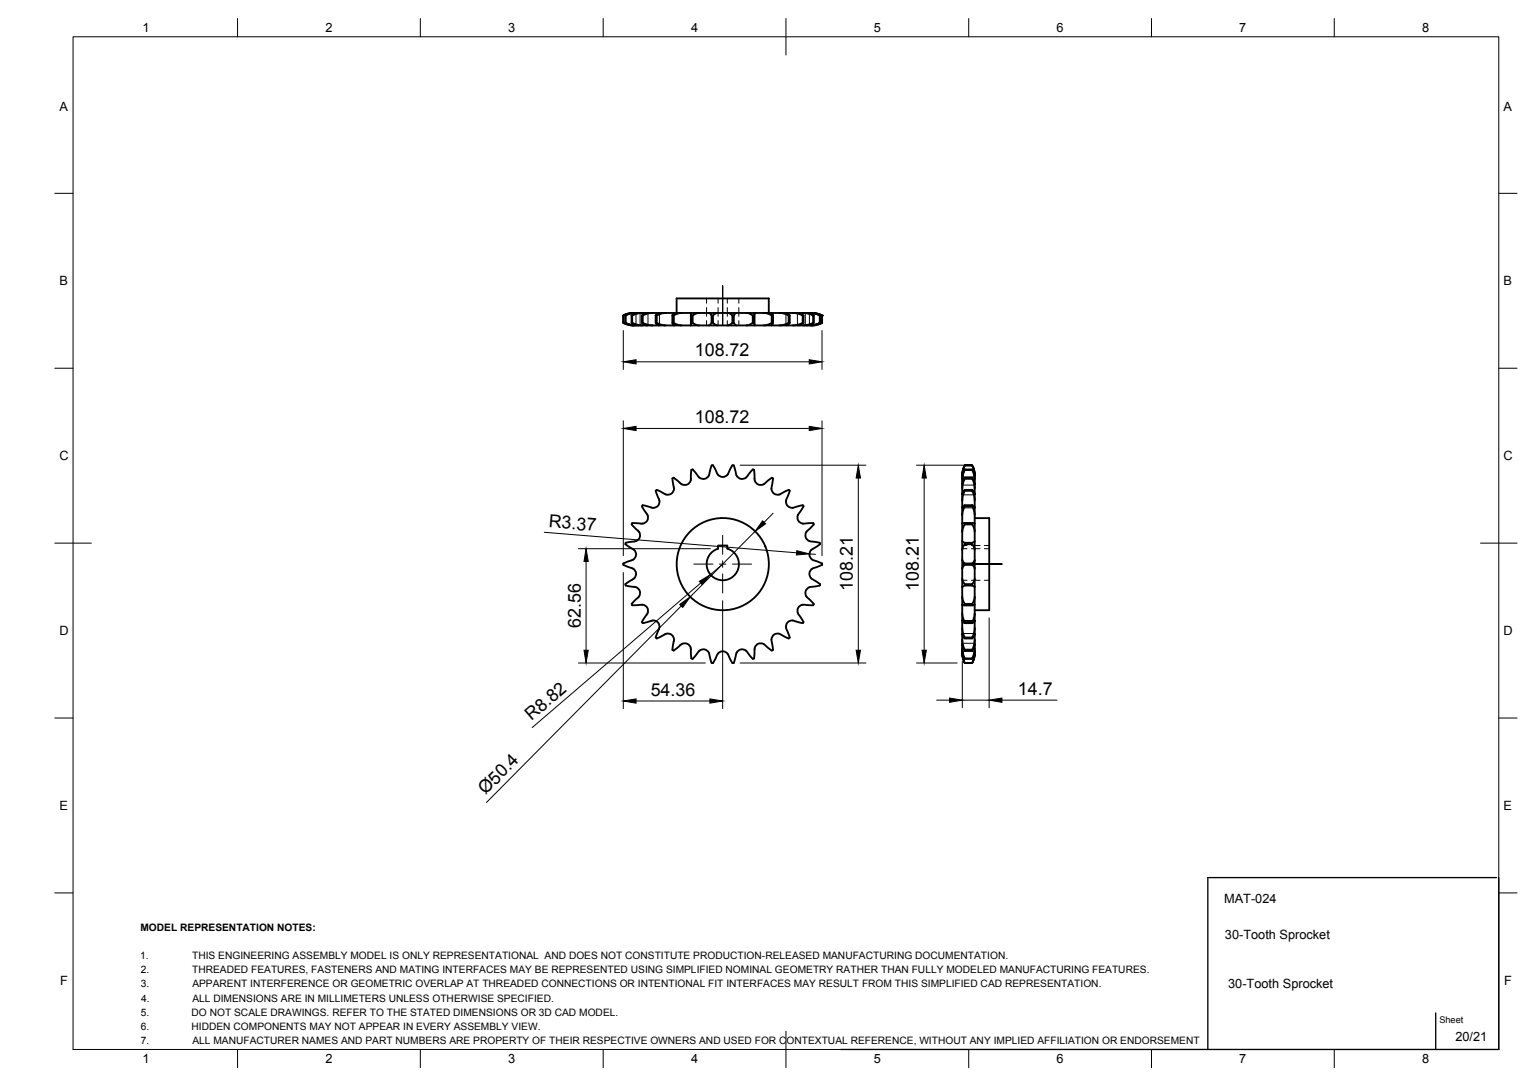
ISO-10303-21;
HEADER;
/* Generated by software containing ST-Developer
 * from STEP Tools, Inc. (www.steptools.com) 
 */

FILE_DESCRIPTION(
/* description */ ('STEP AP214'),
/* implementation_level */ '2;1');

FILE_NAME(
/* name */ '30-Tooth Sprocket.step',
/* time_stamp */ '2026-11-14T06:34:07-08:00',
/* author */ (''),
/* organization */ (''),
/* preprocessor_version */ 'ST-DEVELOPER v20.2',
/* originating_system */ 'Autodesk Translation Framework v15.17.0.0',
/* authorisation */ '');

FILE_SCHEMA (('AUTOMOTIVE_DESIGN { 1 0 10303 214 3 1 1 }'));
ENDSEC;

DATA;
#10=MECHANICAL_DESIGN_GEOMETRIC_PRESENTATION_REPRESENTATION('',(#7281),#310623);
#4055=TOROIDAL_SURFACE('',#103548,25.536,0.336);
#4056=TOROIDAL_SURFACE('',#103592,49.1019873874548,10.668);
#4057=TOROIDAL_SURFACE('',#103597,49.1019873874548,10.668);
#4058=TOROIDAL_SURFACE('',#103651,49.1019873874548,10.668);
#4059=TOROIDAL_SURFACE('',#103653,49.1019873874548,10.668);
#4060=TOROIDAL_SURFACE('',#103655,49.1019873874548,10.668);
#4061=TOROIDAL_SURFACE('',#103657,49.1019873874548,10.668);
#4062=TOROIDAL_SURFACE('',#103659,49.1019873874548,10.668);
#4063=TOROIDAL_SURFACE('',#103661,49.1019873874548,10.668);
#4064=TOROIDAL_SURFACE('',#103663,49.1019873874548,10.668);
#4065=TOROIDAL_SURFACE('',#103665,49.1019873874548,10.668);
#4066=TOROIDAL_SURFACE('',#103667,49.1019873874548,10.668);
#4067=TOROIDAL_SURFACE('',#103669,49.1019873874548,10.668);
#4068=TOROIDAL_SURFACE('',#103671,49.1019873874548,10.668);
#4069=TOROIDAL_SURFACE('',#103673,49.1019873874548,10.668);
#4070=TOROIDAL_SURFACE('',#103675,49.1019873874548,10.668);
#4071=TOROIDAL_SURFACE('',#103677,49.1019873874548,10.668);
#4072=TOROIDAL_SURFACE('',#103679,49.1019873874548,10.668);
#4073=TOROIDAL_SURFACE('',#103681,49.1019873874548,10.668);
#4074=TOROIDAL_SURFACE('',#103683,49.1019873874548,10.668);
#4075=TOROIDAL_SURFACE('',#103685,49.1019873874548,10.668);
#4076=TOROIDAL_SURFACE('',#103687,49.1019873874548,10.668);
#4077=TOROIDAL_SURFACE('',#103689,49.1019873874548,10.668);
#4078=TOROIDAL_SURFACE('',#103691,49.1019873874548,10.668);
#4079=TOROIDAL_SURFACE('',#103693,49.1019873874548,10.668);
#4080=TOROIDAL_SURFACE('',#103695,49.1019873874548,10.668);
#4081=TOROIDAL_SURFACE('',#103697,49.1019873874548,10.668);
#4082=TOROIDAL_SURFACE('',#103699,49.1019873874548,10.668);
#4083=TOROIDAL_SURFACE('',#103701,49.1019873874548,10.668);
#4084=TOROIDAL_SURFACE('',#103703,49.1019873874548,10.668);
#4085=TOROIDAL_SURFACE('',#103705,49.1019873874548,10.668);
#4086=TOROIDAL_SURFACE('',#103763,49.1019873874548,10.668);
#4087=TOROIDAL_SURFACE('',#103765,49.1019873874548,10.668);
#4088=TOROIDAL_SURFACE('',#103767,49.1019873874548,10.668);
#4089=TOROIDAL_SURFACE('',#103769,49.1019873874548,10.668);
#4090=TOROIDAL_SURFACE('',#103771,49.1019873874548,10.668);
#4091=TOROIDAL_SURFACE('',#103773,49.1019873874548,10.668);
#4092=TOROIDAL_SURFACE('',#103775,49.1019873874548,10.668);
#4093=TOROIDAL_SURFACE('',#103777,49.1019873874548,10.668);
#4094=TOROIDAL_SURFACE('',#103779,49.1019873874548,10.668);
#4095=TOROIDAL_SURFACE('',#103781,49.1019873874548,10.668);
#4096=TOROIDAL_SURFACE('',#103783,49.1019873874548,10.668);
#4097=TOROIDAL_SURFACE('',#103785,49.1019873874548,10.668);
#4098=TOROIDAL_SURFACE('',#103787,49.1019873874548,10.668);
#4099=TOROIDAL_SURFACE('',#103789,49.1019873874548,10.668);
#4100=TOROIDAL_SURFACE('',#103791,49.1019873874548,10.668);
#4101=TOROIDAL_SURFACE('',#103793,49.1019873874548,10.668);
#4102=TOROIDAL_SURFACE('',#103795,49.1019873874548,10.668);
#4103=TOROIDAL_SURFACE('',#103797,49.1019873874548,10.668);
#4104=TOROIDAL_SURFACE('',#103799,49.1019873874548,10.668);
#4105=TOROIDAL_SURFACE('',#103801,49.1019873874548,10.668);
#4106=TOROIDAL_SURFACE('',#103803,49.1019873874548,10.668);
#4107=TOROIDAL_SURFACE('',#103805,49.1019873874548,10.668);
#4108=TOROIDAL_SURFACE('',#103807,49.1019873874548,10.668);
#4109=TOROIDAL_SURFACE('',#103809,49.1019873874548,10.668);
#4110=TOROIDAL_SURFACE('',#103811,49.1019873874548,10.668);
#4111=TOROIDAL_SURFACE('',#103813,49.1019873874548,10.668);
#4112=TOROIDAL_SURFACE('',#103815,49.1019873874548,10.668);
#4113=TOROIDAL_SURFACE('',#103817,49.1019873874548,10.668);
#4114=TOROIDAL_SURFACE('',#103819,49.1019873874548,10.668);
#4115=TOROIDAL_SURFACE('',#103823,49.1019873874548,10.668);
#6426=B_SPLINE_CURVE_WITH_KNOTS('',3,(#272477,#272478,#272479,#272480,#272481,
#272482),.UNSPECIFIED.,.F.,.F.,(4,2,4),(-1.6873876187543,-1.63190661744399,
-1.18678936119335),.UNSPECIFIED.);
#6427=B_SPLINE_CURVE_WITH_KNOTS('',3,(#272486,#272487,#272488,#272489,#272490,
#272491,#272492,#272493),.UNSPECIFIED.,.F.,.F.,(4,2,2,4),(-5.73653316281924,
-5.72047347154335,-5.28796112447222,-5.23617773822564),.UNSPECIFIED.);
#6428=B_SPLINE_CURVE_WITH_KNOTS('',3,(#272498,#272499,#272500,#272501,#272502,
#272503,#272504,#272505),.UNSPECIFIED.,.F.,.F.,(4,2,2,4),(-5.73653316281959,
-5.72047347154369,-5.28796112447255,-5.23617773822598),.UNSPECIFIED.);
#6429=B_SPLINE_CURVE_WITH_KNOTS('',3,(#272509,#272510,#272511,#272512,#272513,
#272514),.UNSPECIFIED.,.F.,.F.,(4,2,4),(-1.68738761875429,-1.63190661744397,
-1.18678936119331),.UNSPECIFIED.);
#6430=B_SPLINE_CURVE_WITH_KNOTS('',3,(#272521,#272522,#272523,#272524,#272525,
#272526,#272527,#272528,#272529,#272530),.UNSPECIFIED.,.F.,.F.,(4,3,3,4),
(0.00710274596862205,0.00747376540688557,0.00783502386845829,0.00801837063754701),
 .UNSPECIFIED.);
#6431=B_SPLINE_CURVE_WITH_KNOTS('',3,(#272534,#272535,#272536,#272537),
 .UNSPECIFIED.,.F.,.F.,(4,4),(0.673390429668365,0.765903724821262),
 .UNSPECIFIED.);
#6432=B_SPLINE_CURVE_WITH_KNOTS('',3,(#272541,#272542,#272543,#272544,#272545,
#272546,#272547,#272548,#272549,#272550),.UNSPECIFIED.,.F.,.F.,(4,3,3,4),
(0.00710284094402589,0.00747383068998922,0.00783505699281219,0.0080184642589637),
 .UNSPECIFIED.);
#6433=B_SPLINE_CURVE_WITH_KNOTS('',3,(#272553,#272554,#272555,#272556,#272557,
#272558),.UNSPECIFIED.,.F.,.F.,(4,2,4),(1.75167822390513,1.82489845087556,
1.84415950245262),.UNSPECIFIED.);
#6434=B_SPLINE_CURVE_WITH_KNOTS('',3,(#272564,#272565,#272566,#272567,#272568,
#272569,#272570,#272571,#272572,#272573),.UNSPECIFIED.,.F.,.F.,(4,3,3,4),
(0.00710274294853988,0.00747376648681281,0.00783502929878955,0.00801836762245747),
 .UNSPECIFIED.);
#6435=B_SPLINE_CURVE_WITH_KNOTS('',3,(#272577,#272578,#272579,#272580),
 .UNSPECIFIED.,.F.,.F.,(4,4),(0.673390429683384,0.765903724839824),
 .UNSPECIFIED.);
#6436=B_SPLINE_CURVE_WITH_KNOTS('',3,(#272584,#272585,#272586,#272587,#272588,
#272589,#272590,#272591,#272592,#272593),.UNSPECIFIED.,.F.,.F.,(4,3,3,4),
(0.0071027909646029,0.00747379949023628,0.00783504604208146,0.00801841495400679),
 .UNSPECIFIED.);
#6437=B_SPLINE_CURVE_WITH_KNOTS('',3,(#272596,#272597,#272598,#272599,#272600,
#272601),.UNSPECIFIED.,.F.,.F.,(4,2,4),(1.7516782239595,1.82489845093397,
1.84415950251209),.UNSPECIFIED.);
#6438=B_SPLINE_CURVE_WITH_KNOTS('',3,(#272607,#272608,#272609,#272610,#272611,
#272612,#272613,#272614,#272615,#272616),.UNSPECIFIED.,.F.,.F.,(4,3,3,4),
(0.00710274848401425,0.00747377224143413,0.00783503523508107,0.00801837305550075),
 .UNSPECIFIED.);
#6439=B_SPLINE_CURVE_WITH_KNOTS('',3,(#272620,#272621,#272622,#272623),
 .UNSPECIFIED.,.F.,.F.,(4,4),(0.673390432198586,0.765903727898388),
 .UNSPECIFIED.);
#6440=B_SPLINE_CURVE_WITH_KNOTS('',3,(#272627,#272628,#272629,#272630,#272631,
#272632,#272633,#272634,#272635,#272636),.UNSPECIFIED.,.F.,.F.,(4,3,3,4),
(0.00710275267632021,0.00747377512290787,0.00783503669679513,0.00801837718804213),
 .UNSPECIFIED.);
#6441=B_SPLINE_CURVE_WITH_KNOTS('',3,(#272639,#272640,#272641,#272642,#272643,
#272644),.UNSPECIFIED.,.F.,.F.,(4,2,4),(1.75167822396455,1.82489845093931,
1.84415950251752),.UNSPECIFIED.);
#6442=B_SPLINE_CURVE_WITH_KNOTS('',3,(#272650,#272651,#272652,#272653,#272654,
#272655,#272656,#272657,#272658,#272659),.UNSPECIFIED.,.F.,.F.,(4,3,3,4),
(0.00710274372650064,0.00747376845075347,0.00783503250649641,0.00801836837208912),
 .UNSPECIFIED.);
#6443=B_SPLINE_CURVE_WITH_KNOTS('',3,(#272663,#272664,#272665,#272666),
 .UNSPECIFIED.,.F.,.F.,(4,4),(0.673390432227944,0.765903727934262),
 .UNSPECIFIED.);
#6444=B_SPLINE_CURVE_WITH_KNOTS('',3,(#272670,#272671,#272672,#272673,#272674,
#272675,#272676,#272677,#272678,#272679),.UNSPECIFIED.,.F.,.F.,(4,3,3,4),
(0.00710276617990407,0.00747378388366959,0.00783504033541444,0.00801839050540093),
 .UNSPECIFIED.);
#6445=B_SPLINE_CURVE_WITH_KNOTS('',3,(#272682,#272683,#272684,#272685,#272686,
#272687),.UNSPECIFIED.,.F.,.F.,(4,2,4),(1.7516782239634,1.82489845093825,
1.84415950251648),.UNSPECIFIED.);
#6446=B_SPLINE_CURVE_WITH_KNOTS('',3,(#272691,#272692,#272693,#272694,#272695,
#272696),.UNSPECIFIED.,.F.,.F.,(4,2,4),(0.311414679923399,0.386708223984938,
0.403787209257592),.UNSPECIFIED.);
#6447=B_SPLINE_CURVE_WITH_KNOTS('',3,(#272700,#272701,#272702,#272703),
 .UNSPECIFIED.,.F.,.F.,(4,4),(0.673390427100202,0.765903721697738),
 .UNSPECIFIED.);
#6448=B_SPLINE_CURVE_WITH_KNOTS('',3,(#272707,#272708,#272709,#272710,#272711,
#272712,#272713,#272714,#272715,#272716),.UNSPECIFIED.,.F.,.F.,(4,3,3,4),
(0.00710274287152855,0.00747376729113706,0.00783503103327042,0.00801836753620372),
 .UNSPECIFIED.);
#6449=B_SPLINE_CURVE_WITH_KNOTS('',3,(#272720,#272721,#272722,#272723,#272724,
#272725),.UNSPECIFIED.,.F.,.F.,(4,2,4),(1.75167822395949,1.82489845093397,
1.8441595025121),.UNSPECIFIED.);
#6450=B_SPLINE_CURVE_WITH_KNOTS('',3,(#272730,#272731,#272732,#272733,#272734,
#272735),.UNSPECIFIED.,.F.,.F.,(4,2,4),(0.311414679921635,0.386708223982506,
0.403787209254994),.UNSPECIFIED.);
#6451=B_SPLINE_CURVE_WITH_KNOTS('',3,(#272739,#272740,#272741,#272742),
 .UNSPECIFIED.,.F.,.F.,(4,4),(0.67339042968077,0.765903724836084),
 .UNSPECIFIED.);
#6452=B_SPLINE_CURVE_WITH_KNOTS('',3,(#272746,#272747,#272748,#272749,#272750,
#272751,#272752,#272753,#272754,#272755),.UNSPECIFIED.,.F.,.F.,(4,3,3,4),
(0.00710274556156679,0.00747377006444483,0.00783503387032176,0.00801837017674505),
 .UNSPECIFIED.);
#6453=B_SPLINE_CURVE_WITH_KNOTS('',3,(#272759,#272760,#272761,#272762,#272763,
#272764),.UNSPECIFIED.,.F.,.F.,(4,2,4),(1.75167822393186,1.82489845090426,
1.84415950248185),.UNSPECIFIED.);
#6454=B_SPLINE_CURVE_WITH_KNOTS('',3,(#272769,#272770,#272771,#272772,#272773,
#272774),.UNSPECIFIED.,.F.,.F.,(4,2,4),(1.75167822396114,1.82489845093575,
1.84415950251343),.UNSPECIFIED.);
#6455=B_SPLINE_CURVE_WITH_KNOTS('',3,(#272778,#272779,#272780,#272781,#272782,
#272783,#272784,#272785,#272786,#272787),.UNSPECIFIED.,.F.,.F.,(4,3,3,4),
(0.00710274556156676,0.00747377006444954,0.00783503387033569,0.00801837017674508),
 .UNSPECIFIED.);
#6456=B_SPLINE_CURVE_WITH_KNOTS('',3,(#272791,#272792,#272793,#272794),
 .UNSPECIFIED.,.F.,.F.,(4,4),(0.673390429683286,0.765903724839261),
 .UNSPECIFIED.);
#6457=B_SPLINE_CURVE_WITH_KNOTS('',3,(#272798,#272799,#272800,#272801,#272802,
#272803),.UNSPECIFIED.,.F.,.F.,(4,2,4),(1.38841536190411,1.44431919666813,
1.480702891614),.UNSPECIFIED.);
#6458=B_SPLINE_CURVE_WITH_KNOTS('',3,(#272810,#272811,#272812,#272813,#272814,
#272815,#272816,#272817,#272818,#272819),.UNSPECIFIED.,.F.,.F.,(4,3,3,4),
(0.00710275267632017,0.00747377512292421,0.00783503669676932,0.00801837718804213),
 .UNSPECIFIED.);
#6459=B_SPLINE_CURVE_WITH_KNOTS('',3,(#272823,#272824,#272825,#272826),
 .UNSPECIFIED.,.F.,.F.,(4,4),(0.673390429659051,0.765903724809687),
 .UNSPECIFIED.);
#6460=B_SPLINE_CURVE_WITH_KNOTS('',3,(#272830,#272831,#272832,#272833,#272834,
#272835,#272836,#272837,#272838,#272839),.UNSPECIFIED.,.F.,.F.,(4,3,3,4),
(0.00710274848401431,0.00747377224144616,0.00783503523508854,0.00801837305550078),
 .UNSPECIFIED.);
#6461=B_SPLINE_CURVE_WITH_KNOTS('',3,(#272842,#272843,#272844,#272845,#272846,
#272847),.UNSPECIFIED.,.F.,.F.,(4,2,4),(1.75167822393867,1.82489845091149,
1.8441595024892),.UNSPECIFIED.);
#6462=B_SPLINE_CURVE_WITH_KNOTS('',3,(#272851,#272852,#272853,#272854,#272855,
#272856),.UNSPECIFIED.,.F.,.F.,(4,2,4),(1.75167822389203,1.8248984508612,
1.84415950243739),.UNSPECIFIED.);
#6463=B_SPLINE_CURVE_WITH_KNOTS('',3,(#272860,#272861,#272862,#272863,#272864,
#272865,#272866,#272867,#272868,#272869),.UNSPECIFIED.,.F.,.F.,(4,3,3,4),
(0.00710274287152849,0.00747376729116317,0.00783503103329361,0.00801836753620371),
 .UNSPECIFIED.);
#6464=B_SPLINE_CURVE_WITH_KNOTS('',3,(#272873,#272874,#272875,#272876),
 .UNSPECIFIED.,.F.,.F.,(4,4),(0.673390429665128,0.765903724817488),
 .UNSPECIFIED.);
#6465=B_SPLINE_CURVE_WITH_KNOTS('',3,(#272880,#272881,#272882,#272883,#272884,
#272885),.UNSPECIFIED.,.F.,.F.,(4,2,4),(1.38841536184886,1.444319196609,
1.48070289155233),.UNSPECIFIED.);
#6466=B_SPLINE_CURVE_WITH_KNOTS('',3,(#272892,#272893,#272894,#272895,#272896,
#272897,#272898,#272899,#272900,#272901),.UNSPECIFIED.,.F.,.F.,(4,3,3,4),
(0.00710276617990401,0.00747378388366924,0.00783504033542184,0.00801839050540089),
 .UNSPECIFIED.);
#6467=B_SPLINE_CURVE_WITH_KNOTS('',3,(#272905,#272906,#272907,#272908),
 .UNSPECIFIED.,.F.,.F.,(4,4),(0.673390432231233,0.765903727938084),
 .UNSPECIFIED.);
#6468=B_SPLINE_CURVE_WITH_KNOTS('',3,(#272912,#272913,#272914,#272915,#272916,
#272917,#272918,#272919,#272920,#272921),.UNSPECIFIED.,.F.,.F.,(4,3,3,4),
(0.00710274372650068,0.00747376845078837,0.00783503250653971,0.00801836837208909),
 .UNSPECIFIED.);
#6469=B_SPLINE_CURVE_WITH_KNOTS('',3,(#272924,#272925,#272926,#272927,#272928,
#272929),.UNSPECIFIED.,.F.,.F.,(4,2,4),(1.75167822389501,1.82489845086412,
1.84415950244083),.UNSPECIFIED.);
#6470=B_SPLINE_CURVE_WITH_KNOTS('',3,(#272935,#272936,#272937,#272938,#272939,
#272940,#272941,#272942,#272943,#272944),.UNSPECIFIED.,.F.,.F.,(4,3,3,4),
(0.00710279096460286,0.00747379949026601,0.00783504604209238,0.0080184149540068),
 .UNSPECIFIED.);
#6471=B_SPLINE_CURVE_WITH_KNOTS('',3,(#272948,#272949,#272950,#272951),
 .UNSPECIFIED.,.F.,.F.,(4,4),(0.673390429675743,0.765903724830226),
 .UNSPECIFIED.);
#6472=B_SPLINE_CURVE_WITH_KNOTS('',3,(#272955,#272956,#272957,#272958,#272959,
#272960,#272961,#272962,#272963,#272964),.UNSPECIFIED.,.F.,.F.,(4,3,3,4),
(0.00710274294853991,0.0074737664867412,0.0078350292986902,0.00801836762245745),
 .UNSPECIFIED.);
#6473=B_SPLINE_CURVE_WITH_KNOTS('',3,(#272967,#272968,#272969,#272970,#272971,
#272972),.UNSPECIFIED.,.F.,.F.,(4,2,4),(1.75167822398024,1.82489845095654,
1.8441595025352),.UNSPECIFIED.);
#6474=B_SPLINE_CURVE_WITH_KNOTS('',3,(#272978,#272979,#272980,#272981,#272982,
#272983,#272984,#272985,#272986,#272987),.UNSPECIFIED.,.F.,.F.,(4,3,3,4),
(0.00710284094402584,0.00747383069000615,0.00783505699282562,0.00801846425896367),
 .UNSPECIFIED.);
#6475=B_SPLINE_CURVE_WITH_KNOTS('',3,(#272991,#272992,#272993,#272994),
 .UNSPECIFIED.,.F.,.F.,(4,4),(0.673390429692054,0.765903724850254),
 .UNSPECIFIED.);
#6476=B_SPLINE_CURVE_WITH_KNOTS('',3,(#272998,#272999,#273000,#273001,#273002,
#273003,#273004,#273005,#273006,#273007),.UNSPECIFIED.,.F.,.F.,(4,3,3,4),
(0.00710274596862209,0.00747376540702079,0.00783502386859213,0.00801837063754698),
 .UNSPECIFIED.);
#6477=B_SPLINE_CURVE_WITH_KNOTS('',3,(#273010,#273011,#273012,#273013,#273014,
#273015),.UNSPECIFIED.,.F.,.F.,(4,2,4),(1.75167822394042,1.82489845091343,
1.84415950249118),.UNSPECIFIED.);
#6478=B_SPLINE_CURVE_WITH_KNOTS('',3,(#273021,#273022,#273023,#273024,#273025,
#273026),.UNSPECIFIED.,.F.,.F.,(4,2,4),(-1.68738761875423,-1.63190661744391,
-1.18678936119335),.UNSPECIFIED.);
#6479=B_SPLINE_CURVE_WITH_KNOTS('',3,(#273028,#273029,#273030,#273031,#273032,
#273033,#273034,#273035,#273036,#273037),.UNSPECIFIED.,.F.,.F.,(4,3,3,4),
(0.00710284094402589,0.00747383068999436,0.00783505699281514,0.0080184642589637),
 .UNSPECIFIED.);
#6480=B_SPLINE_CURVE_WITH_KNOTS('',3,(#273041,#273042,#273043,#273044),
 .UNSPECIFIED.,.F.,.F.,(4,4),(0.673390429666604,0.7659037248194),
 .UNSPECIFIED.);
#6481=B_SPLINE_CURVE_WITH_KNOTS('',3,(#273045,#273046,#273047,#273048,#273049,
#273050,#273051,#273052),.UNSPECIFIED.,.F.,.F.,(4,2,2,4),(-5.73653316281647,
-5.7204734715406,-5.28796112446986,-5.23617773822333),.UNSPECIFIED.);
#6482=B_SPLINE_CURVE_WITH_KNOTS('',3,(#273064,#273065,#273066,#273067,#273068,
#273069),.UNSPECIFIED.,.F.,.F.,(4,2,4),(1.75167822396951,1.82489845094498,
1.84415950252339),.UNSPECIFIED.);
#6483=B_SPLINE_CURVE_WITH_KNOTS('',3,(#273070,#273071,#273072,#273073,#273074,
#273075,#273076,#273077),.UNSPECIFIED.,.F.,.F.,(4,2,2,4),(-5.73653316281843,
-5.72047347154254,-5.28796112447152,-5.23617773822495),.UNSPECIFIED.);
#6484=B_SPLINE_CURVE_WITH_KNOTS('',3,(#273079,#273080,#273081,#273082,#273083,
#273084),.UNSPECIFIED.,.F.,.F.,(4,2,4),(-1.68738761875408,-1.63190661744377,
-1.18678936119326),.UNSPECIFIED.);
#6485=B_SPLINE_CURVE_WITH_KNOTS('',3,(#273085,#273086,#273087,#273088,#273089,
#273090,#273091,#273092,#273093,#273094),.UNSPECIFIED.,.F.,.F.,(4,3,3,4),
(0.00710284094402584,0.00747383068999716,0.00783505699282223,0.00801846425896371),
 .UNSPECIFIED.);
#6486=B_SPLINE_CURVE_WITH_KNOTS('',3,(#273200,#273201,#273202,#273203,#273204,
#273205,#273206,#273207),.UNSPECIFIED.,.F.,.F.,(4,2,2,4),(-5.73653316281843,
-5.72047347154255,-5.28796112447153,-5.23617773822497),.UNSPECIFIED.);
#6487=B_SPLINE_CURVE_WITH_KNOTS('',3,(#273211,#273212,#273213,#273214,#273215,
#273216),.UNSPECIFIED.,.F.,.F.,(4,2,4),(-1.68738761875411,-1.6319066174438,
-1.18678936119328),.UNSPECIFIED.);
#6488=B_SPLINE_CURVE_WITH_KNOTS('',3,(#273217,#273218,#273219,#273220,#273221,
#273222,#273223,#273224,#273225,#273226),.UNSPECIFIED.,.F.,.F.,(4,3,3,4),
(0.00710279096460287,0.00747379949022753,0.00783504604206607,0.00801841495400678),
 .UNSPECIFIED.);
#6489=B_SPLINE_CURVE_WITH_KNOTS('',3,(#273227,#273228,#273229,#273230,#273231,
#273232),.UNSPECIFIED.,.F.,.F.,(4,2,4),(1.75167822397008,1.82489845094558,
1.84415950252402),.UNSPECIFIED.);
#6490=B_SPLINE_CURVE_WITH_KNOTS('',3,(#273235,#273236,#273237,#273238,#273239,
#273240,#273241,#273242,#273243,#273244),.UNSPECIFIED.,.F.,.F.,(4,3,3,4),
(0.00710274596862205,0.00747376540693236,0.00783502386849402,0.00801837063754702),
 .UNSPECIFIED.);
#6491=B_SPLINE_CURVE_WITH_KNOTS('',3,(#273246,#273247,#273248,#273249,#273250,
#273251),.UNSPECIFIED.,.F.,.F.,(4,2,4),(1.75167822396416,1.82489845093897,
1.84415950251715),.UNSPECIFIED.);
#6492=B_SPLINE_CURVE_WITH_KNOTS('',3,(#273253,#273254,#273255,#273256,#273257,
#273258,#273259,#273260),.UNSPECIFIED.,.F.,.F.,(4,2,2,4),(-5.73653316281831,
-5.72047347154243,-5.28796112447143,-5.23617773822487),.UNSPECIFIED.);
#6493=B_SPLINE_CURVE_WITH_KNOTS('',3,(#273263,#273264,#273265,#273266,#273267,
#273268),.UNSPECIFIED.,.F.,.F.,(4,2,4),(-1.68738761875401,-1.63190661744371,
-1.18678936119322),.UNSPECIFIED.);
#6494=B_SPLINE_CURVE_WITH_KNOTS('',3,(#273271,#273272,#273273,#273274,#273275,
#273276,#273277,#273278,#273279,#273280),.UNSPECIFIED.,.F.,.F.,(4,3,3,4),
(0.00710274294853987,0.00747376648670428,0.00783502929868148,0.00801836762245748),
 .UNSPECIFIED.);
#6495=B_SPLINE_CURVE_WITH_KNOTS('',3,(#273282,#273283,#273284,#273285,#273286,
#273287),.UNSPECIFIED.,.F.,.F.,(4,2,4),(1.75167822398049,1.82489845095657,
1.84415950253511),.UNSPECIFIED.);
#6496=B_SPLINE_CURVE_WITH_KNOTS('',3,(#273289,#273290,#273291,#273292,#273293,
#273294,#273295,#273296),.UNSPECIFIED.,.F.,.F.,(4,2,2,4),(-5.73653316281822,
-5.72047347154233,-5.28796112447135,-5.23617773822479),.UNSPECIFIED.);
#6497=B_SPLINE_CURVE_WITH_KNOTS('',3,(#273299,#273300,#273301,#273302,#273303,
#273304),.UNSPECIFIED.,.F.,.F.,(4,2,4),(-1.68738761875411,-1.6319066174438,
-1.18678936119327),.UNSPECIFIED.);
#6498=B_SPLINE_CURVE_WITH_KNOTS('',3,(#273307,#273308,#273309,#273310,#273311,
#273312,#273313,#273314,#273315,#273316),.UNSPECIFIED.,.F.,.F.,(4,3,3,4),
(0.00710274372650065,0.00747376845074211,0.00783503250649763,0.00801836837208913),
 .UNSPECIFIED.);
#6499=B_SPLINE_CURVE_WITH_KNOTS('',3,(#273318,#273319,#273320,#273321,#273322,
#273323),.UNSPECIFIED.,.F.,.F.,(4,2,4),(1.75167822398513,1.82489845096143,
1.84415950254005),.UNSPECIFIED.);
#6500=B_SPLINE_CURVE_WITH_KNOTS('',3,(#273325,#273326,#273327,#273328,#273329,
#273330,#273331,#273332),.UNSPECIFIED.,.F.,.F.,(4,2,2,4),(-5.73653316281763,
-5.72047347154175,-5.2879611244708,-5.23617773822424),.UNSPECIFIED.);
#6501=B_SPLINE_CURVE_WITH_KNOTS('',3,(#273335,#273336,#273337,#273338,#273339,
#273340),.UNSPECIFIED.,.F.,.F.,(4,2,4),(-1.68738761875406,-1.63190661744375,
-1.18678936119324),.UNSPECIFIED.);
#6502=B_SPLINE_CURVE_WITH_KNOTS('',3,(#273344,#273345,#273346,#273347,#273348,
#273349,#273350,#273351),.UNSPECIFIED.,.F.,.F.,(4,2,2,4),(-5.73653316281763,
-5.72047347154175,-5.28796112447086,-5.2361777382243),.UNSPECIFIED.);
#6503=B_SPLINE_CURVE_WITH_KNOTS('',3,(#273355,#273356,#273357,#273358,#273359,
#273360),.UNSPECIFIED.,.F.,.F.,(4,2,4),(-1.6873876187539,-1.6319066174436,
-1.18678936119314),.UNSPECIFIED.);
#6504=B_SPLINE_CURVE_WITH_KNOTS('',3,(#273361,#273362,#273363,#273364,#273365,
#273366,#273367,#273368,#273369,#273370),.UNSPECIFIED.,.F.,.F.,(4,3,3,4),
(0.00710275842609582,0.00747377890657602,0.00783503835572276,0.00801838285788017),
 .UNSPECIFIED.);
#6505=B_SPLINE_CURVE_WITH_KNOTS('',3,(#273371,#273372,#273373,#273374,#273375,
#273376),.UNSPECIFIED.,.F.,.F.,(4,2,4),(1.75167822396027,1.82489845093474,
1.84415950251286),.UNSPECIFIED.);
#6506=B_SPLINE_CURVE_WITH_KNOTS('',3,(#273378,#273379,#273380,#273381,#273382,
#273383,#273384,#273385,#273386,#273387),.UNSPECIFIED.,.F.,.F.,(4,3,3,4),
(0.00710277664195228,0.00747379050272964,0.00783504280851268,0.00801840082520104),
 .UNSPECIFIED.);
#6507=B_SPLINE_CURVE_WITH_KNOTS('',3,(#273389,#273390,#273391,#273392,#273393,
#273394),.UNSPECIFIED.,.F.,.F.,(4,2,4),(1.75167822402901,1.82489845100883,
1.84415950258839),.UNSPECIFIED.);
#6508=B_SPLINE_CURVE_WITH_KNOTS('',3,(#273396,#273397,#273398,#273399,#273400,
#273401,#273402,#273403),.UNSPECIFIED.,.F.,.F.,(4,2,2,4),(-5.73653316281821,
-5.72047347154232,-5.28796112447134,-5.23617773822477),.UNSPECIFIED.);
#6509=B_SPLINE_CURVE_WITH_KNOTS('',3,(#273407,#273408,#273409,#273410,#273411,
#273412,#273413,#273414,#273415,#273416),.UNSPECIFIED.,.F.,.F.,(4,3,3,4),
(0.00710274848401426,0.00747377224139712,0.00783503523503374,0.00801837305550079),
 .UNSPECIFIED.);
#6510=B_SPLINE_CURVE_WITH_KNOTS('',3,(#273418,#273419,#273420,#273421,#273422,
#273423),.UNSPECIFIED.,.F.,.F.,(4,2,4),(1.75167822392663,1.82489845089845,
1.84415950247588),.UNSPECIFIED.);
#6511=B_SPLINE_CURVE_WITH_KNOTS('',3,(#273425,#273426,#273427,#273428,#273429,
#273430,#273431,#273432),.UNSPECIFIED.,.F.,.F.,(4,2,2,4),(-5.73653316281796,
-5.72047347154208,-5.28796112447113,-5.23617773822457),.UNSPECIFIED.);
#6512=B_SPLINE_CURVE_WITH_KNOTS('',3,(#273435,#273436,#273437,#273438,#273439,
#273440),.UNSPECIFIED.,.F.,.F.,(4,2,4),(-1.68738761875412,-1.63190661744382,
-1.1867893611933),.UNSPECIFIED.);
#6513=B_SPLINE_CURVE_WITH_KNOTS('',3,(#273444,#273445,#273446,#273447,#273448,
#273449,#273450,#273451),.UNSPECIFIED.,.F.,.F.,(4,2,2,4),(-5.73653316281711,
-5.72047347154123,-5.28796112447036,-5.23617773822381),.UNSPECIFIED.);
#6514=B_SPLINE_CURVE_WITH_KNOTS('',3,(#273455,#273456,#273457,#273458,#273459,
#273460),.UNSPECIFIED.,.F.,.F.,(4,2,4),(-1.68738761875405,-1.63190661744374,
-1.18678936119325),.UNSPECIFIED.);
#6515=B_SPLINE_CURVE_WITH_KNOTS('',3,(#273461,#273462,#273463,#273464,#273465,
#273466,#273467,#273468,#273469,#273470),.UNSPECIFIED.,.F.,.F.,(4,3,3,4),
(0.00710281114521604,0.00747381210003836,0.00783505048827464,0.00801843486213954),
 .UNSPECIFIED.);
#6516=B_SPLINE_CURVE_WITH_KNOTS('',3,(#273471,#273472,#273473,#273474,#273475,
#273476),.UNSPECIFIED.,.F.,.F.,(4,2,4),(1.75167822397278,1.8248984509485,
1.84415950252695),.UNSPECIFIED.);
#6517=B_SPLINE_CURVE_WITH_KNOTS('',3,(#273479,#273480,#273481,#273482,#273483,
#273484,#273485,#273486,#273487,#273488),.UNSPECIFIED.,.F.,.F.,(4,3,3,4),
(0.0071027490873384,0.00747377283389233,0.0078350358106713,0.00801837364807993),
 .UNSPECIFIED.);
#6518=B_SPLINE_CURVE_WITH_KNOTS('',3,(#273490,#273491,#273492,#273493,#273494,
#273495),.UNSPECIFIED.,.F.,.F.,(4,2,4),(1.75167822393089,1.82489845090296,
1.84415950248043),.UNSPECIFIED.);
#6519=B_SPLINE_CURVE_WITH_KNOTS('',3,(#273497,#273498,#273499,#273500,#273501,
#273502,#273503,#273504),.UNSPECIFIED.,.F.,.F.,(4,2,2,4),(-5.73653316281819,
-5.7204734715423,-5.2879611244713,-5.23617773822474),.UNSPECIFIED.);
#6520=B_SPLINE_CURVE_WITH_KNOTS('',3,(#273507,#273508,#273509,#273510,#273511,
#273512),.UNSPECIFIED.,.F.,.F.,(4,2,4),(-1.68738761875405,-1.63190661744374,
-1.18678936119326),.UNSPECIFIED.);
#6521=B_SPLINE_CURVE_WITH_KNOTS('',3,(#273515,#273516,#273517,#273518,#273519,
#273520,#273521,#273522,#273523,#273524),.UNSPECIFIED.,.F.,.F.,(4,3,3,4),
(0.00710274396181581,0.00747376592129383,0.00783502705943546,0.00801836863650809),
 .UNSPECIFIED.);
#6522=B_SPLINE_CURVE_WITH_KNOTS('',3,(#273525,#273526,#273527,#273528,#273529,
#273530),.UNSPECIFIED.,.F.,.F.,(4,2,4),(1.75167822392141,1.82489845089256,
1.84415950246982),.UNSPECIFIED.);
#6523=B_SPLINE_CURVE_WITH_KNOTS('',3,(#273533,#273534,#273535,#273536,#273537,
#273538),.UNSPECIFIED.,.F.,.F.,(4,2,4),(-1.68738761875407,-1.63190661744377,
-1.18678936119326),.UNSPECIFIED.);
#6524=B_SPLINE_CURVE_WITH_KNOTS('',3,(#273542,#273543,#273544,#273545,#273546,
#273547,#273548,#273549),.UNSPECIFIED.,.F.,.F.,(4,2,2,4),(-5.73653316281851,
-5.72047347154262,-5.2879611244716,-5.23617773822503),.UNSPECIFIED.);
#6525=B_SPLINE_CURVE_WITH_KNOTS('',3,(#273553,#273554,#273555,#273556,#273557,
#273558),.UNSPECIFIED.,.F.,.F.,(4,2,4),(-1.68738761875428,-1.63190661744396,
-1.18678936119339),.UNSPECIFIED.);
#6526=B_SPLINE_CURVE_WITH_KNOTS('',3,(#273559,#273560,#273561,#273562,#273563,
#273564,#273565,#273566,#273567,#273568),.UNSPECIFIED.,.F.,.F.,(4,3,3,4),
(0.00710274287152851,0.00747376729109832,0.00783503103323433,0.00801836753620372),
 .UNSPECIFIED.);
#6527=B_SPLINE_CURVE_WITH_KNOTS('',3,(#273569,#273570,#273571,#273572,#273573,
#273574),.UNSPECIFIED.,.F.,.F.,(4,2,4),(1.75167822396654,1.8248984509415,
1.84415950251975),.UNSPECIFIED.);
#6528=B_SPLINE_CURVE_WITH_KNOTS('',3,(#273577,#273578,#273579,#273580,#273581,
#273582,#273583,#273584,#273585,#273586),.UNSPECIFIED.,.F.,.F.,(4,3,3,4),
(0.00710274556156676,0.00747377006442299,0.00783503387029698,0.00801837017674507),
 .UNSPECIFIED.);
#6529=B_SPLINE_CURVE_WITH_KNOTS('',3,(#273588,#273589,#273590,#273591,#273592,
#273593),.UNSPECIFIED.,.F.,.F.,(4,2,4),(1.75167822394173,1.82489845091482,
1.84415950249256),.UNSPECIFIED.);
#6530=B_SPLINE_CURVE_WITH_KNOTS('',3,(#273595,#273596,#273597,#273598,#273599,
#273600,#273601,#273602),.UNSPECIFIED.,.F.,.F.,(4,2,2,4),(-5.73653316281893,
-5.72047347154304,-5.28796112447197,-5.23617773822539),.UNSPECIFIED.);
#6531=B_SPLINE_CURVE_WITH_KNOTS('',3,(#273605,#273606,#273607,#273608,#273609,
#273610),.UNSPECIFIED.,.F.,.F.,(4,2,4),(-1.68738761875412,-1.63190661744381,
-1.1867893611933),.UNSPECIFIED.);
#6532=B_SPLINE_CURVE_WITH_KNOTS('',3,(#273614,#273615,#273616,#273617,#273618,
#273619,#273620,#273621),.UNSPECIFIED.,.F.,.F.,(4,2,2,4),(-5.73653316281756,
-5.72047347154168,-5.28796112447075,-5.2361777382242),.UNSPECIFIED.);
#6533=B_SPLINE_CURVE_WITH_KNOTS('',3,(#273625,#273626,#273627,#273628,#273629,
#273630),.UNSPECIFIED.,.F.,.F.,(4,2,4),(-1.68738761875423,-1.63190661744392,
-1.18678936119336),.UNSPECIFIED.);
#6534=B_SPLINE_CURVE_WITH_KNOTS('',3,(#273631,#273632,#273633,#273634,#273635,
#273636,#273637,#273638,#273639,#273640),.UNSPECIFIED.,.F.,.F.,(4,3,3,4),
(0.00710275267632017,0.00747377512286913,0.00783503669672892,0.00801837718804214),
 .UNSPECIFIED.);
#6535=B_SPLINE_CURVE_WITH_KNOTS('',3,(#273641,#273642,#273643,#273644,#273645,
#273646),.UNSPECIFIED.,.F.,.F.,(4,2,4),(1.75167822394468,1.82489845091785,
1.84415950249561),.UNSPECIFIED.);
#6536=B_SPLINE_CURVE_WITH_KNOTS('',3,(#273649,#273650,#273651,#273652,#273653,
#273654,#273655,#273656,#273657,#273658),.UNSPECIFIED.,.F.,.F.,(4,3,3,4),
(0.00710276617990402,0.00747378388367883,0.00783504033543201,0.00801839050540095),
 .UNSPECIFIED.);
#6537=B_SPLINE_CURVE_WITH_KNOTS('',3,(#273660,#273661,#273662,#273663,#273664,
#273665),.UNSPECIFIED.,.F.,.F.,(4,2,4),(1.75167822395908,1.82489845093353,
1.84415950251173),.UNSPECIFIED.);
#6538=B_SPLINE_CURVE_WITH_KNOTS('',3,(#273667,#273668,#273669,#273670,#273671,
#273672,#273673,#273674),.UNSPECIFIED.,.F.,.F.,(4,2,2,4),(-5.73653316281958,
-5.72047347154368,-5.28796112447252,-5.23617773822594),.UNSPECIFIED.);
#6539=B_SPLINE_CURVE_WITH_KNOTS('',3,(#273677,#273678,#273679,#273680,#273681,
#273682),.UNSPECIFIED.,.F.,.F.,(4,2,4),(-1.68738761875405,-1.63190661744374,
-1.18678936119325),.UNSPECIFIED.);
#6540=B_SPLINE_CURVE_WITH_KNOTS('',3,(#273685,#273686,#273687,#273688,#273689,
#273690,#273691,#273692),.UNSPECIFIED.,.F.,.F.,(4,2,2,4),(-5.73653316281852,
-5.72047347154263,-5.28796112447155,-5.23617773822497),.UNSPECIFIED.);
#6541=B_SPLINE_CURVE_WITH_KNOTS('',3,(#273695,#273696,#273697,#273698,#273699,
#273700),.UNSPECIFIED.,.F.,.F.,(4,2,4),(-1.68738761875409,-1.63190661744378,
-1.18678936119328),.UNSPECIFIED.);
#6542=B_SPLINE_CURVE_WITH_KNOTS('',3,(#273703,#273704,#273705,#273706,#273707,
#273708,#273709,#273710),.UNSPECIFIED.,.F.,.F.,(4,2,2,4),(-5.73653316281855,
-5.72047347154266,-5.28796112447163,-5.23617773822506),.UNSPECIFIED.);
#6543=B_SPLINE_CURVE_WITH_KNOTS('',3,(#273713,#273714,#273715,#273716,#273717,
#273718),.UNSPECIFIED.,.F.,.F.,(4,2,4),(-1.68738761875414,-1.63190661744383,
-1.18678936119329),.UNSPECIFIED.);
#6544=B_SPLINE_CURVE_WITH_KNOTS('',3,(#273721,#273722,#273723,#273724,#273725,
#273726,#273727,#273728),.UNSPECIFIED.,.F.,.F.,(4,2,2,4),(-5.73653316281849,
-5.7204734715426,-5.28796112447158,-5.23617773822501),.UNSPECIFIED.);
#6545=B_SPLINE_CURVE_WITH_KNOTS('',3,(#273731,#273732,#273733,#273734,#273735,
#273736),.UNSPECIFIED.,.F.,.F.,(4,2,4),(-1.68738761875438,-1.63190661744405,
-1.18678936119344),.UNSPECIFIED.);
#6546=B_SPLINE_CURVE_WITH_KNOTS('',3,(#273739,#273740,#273741,#273742,#273743,
#273744,#273745,#273746),.UNSPECIFIED.,.F.,.F.,(4,2,2,4),(-5.73653316281912,
-5.72047347154323,-5.28796112447213,-5.23617773822555),.UNSPECIFIED.);
#6547=B_SPLINE_CURVE_WITH_KNOTS('',3,(#273749,#273750,#273751,#273752,#273753,
#273754),.UNSPECIFIED.,.F.,.F.,(4,2,4),(-1.68738761875427,-1.63190661744396,
-1.18678936119339),.UNSPECIFIED.);
#6548=B_SPLINE_CURVE_WITH_KNOTS('',3,(#273757,#273758,#273759,#273760,#273761,
#273762,#273763,#273764),.UNSPECIFIED.,.F.,.F.,(4,2,2,4),(-5.73653316281971,
-5.72047347154382,-5.28796112447267,-5.23617773822609),.UNSPECIFIED.);
#6549=B_SPLINE_CURVE_WITH_KNOTS('',3,(#273767,#273768,#273769,#273770,#273771,
#273772),.UNSPECIFIED.,.F.,.F.,(4,2,4),(-1.68738761875429,-1.63190661744397,
-1.18678936119339),.UNSPECIFIED.);
#6550=B_SPLINE_CURVE_WITH_KNOTS('',3,(#273775,#273776,#273777,#273778,#273779,
#273780,#273781,#273782),.UNSPECIFIED.,.F.,.F.,(4,2,2,4),(-5.73653316281998,
-5.72047347154409,-5.28796112447289,-5.2361777382263),.UNSPECIFIED.);
#6551=B_SPLINE_CURVE_WITH_KNOTS('',3,(#273785,#273786,#273787,#273788,#273789,
#273790),.UNSPECIFIED.,.F.,.F.,(4,2,4),(-1.68738761875409,-1.63190661744378,
-1.18678936119326),.UNSPECIFIED.);
#6552=B_SPLINE_CURVE_WITH_KNOTS('',3,(#273793,#273794,#273795,#273796,#273797,
#273798),.UNSPECIFIED.,.F.,.F.,(4,2,4),(1.75167822400724,1.82489845098526,
1.84415950256435),.UNSPECIFIED.);
#6553=B_SPLINE_CURVE_WITH_KNOTS('',3,(#273800,#273801,#273802,#273803,#273804,
#273805,#273806,#273807),.UNSPECIFIED.,.F.,.F.,(4,2,2,4),(-5.73653316281915,
-5.72047347154326,-5.28796112447218,-5.2361777382256),.UNSPECIFIED.);
#6554=B_SPLINE_CURVE_WITH_KNOTS('',3,(#273810,#273811,#273812,#273813,#273814,
#273815),.UNSPECIFIED.,.F.,.F.,(4,2,4),(-1.68738761875405,-1.63190661744374,
-1.18678936119324),.UNSPECIFIED.);
#6555=B_SPLINE_CURVE_WITH_KNOTS('',3,(#273818,#273819,#273820,#273821,#273822,
#273823,#273824,#273825),.UNSPECIFIED.,.F.,.F.,(4,2,2,4),(-5.73653316281814,
-5.72047347154225,-5.28796112447131,-5.23617773822475),.UNSPECIFIED.);
#6556=B_SPLINE_CURVE_WITH_KNOTS('',3,(#273828,#273829,#273830,#273831,#273832,
#273833),.UNSPECIFIED.,.F.,.F.,(4,2,4),(-1.68738761875419,-1.63190661744387,
-1.1867893611933),.UNSPECIFIED.);
#6557=B_SPLINE_CURVE_WITH_KNOTS('',3,(#273836,#273837,#273838,#273839,#273840,
#273841,#273842,#273843),.UNSPECIFIED.,.F.,.F.,(4,2,2,4),(-5.73653316281769,
-5.7204734715418,-5.28796112447084,-5.23617773822428),.UNSPECIFIED.);
#6558=B_SPLINE_CURVE_WITH_KNOTS('',3,(#273846,#273847,#273848,#273849,#273850,
#273851),.UNSPECIFIED.,.F.,.F.,(4,2,4),(-1.68738761875417,-1.63190661744386,
-1.18678936119329),.UNSPECIFIED.);
#6559=B_SPLINE_CURVE_WITH_KNOTS('',3,(#273854,#273855,#273856,#273857,#273858,
#273859,#273860,#273861),.UNSPECIFIED.,.F.,.F.,(4,2,2,4),(-5.73653316281814,
-5.72047347154225,-5.2879611244713,-5.23617773822474),.UNSPECIFIED.);
#6560=B_SPLINE_CURVE_WITH_KNOTS('',3,(#273864,#273865,#273866,#273867,#273868,
#273869),.UNSPECIFIED.,.F.,.F.,(4,2,4),(-1.6873876187541,-1.63190661744379,
-1.18678936119325),.UNSPECIFIED.);
#6561=B_SPLINE_CURVE_WITH_KNOTS('',3,(#273872,#273873,#273874,#273875,#273876,
#273877,#273878,#273879),.UNSPECIFIED.,.F.,.F.,(4,2,2,4),(-5.73653316281885,
-5.72047347154296,-5.28796112447182,-5.23617773822524),.UNSPECIFIED.);
#6562=B_SPLINE_CURVE_WITH_KNOTS('',3,(#273883,#273884,#273885,#273886,#273887,
#273888),.UNSPECIFIED.,.F.,.F.,(4,2,4),(-1.68738761875405,-1.63190661744374,
-1.18678936119323),.UNSPECIFIED.);
#6563=B_SPLINE_CURVE_WITH_KNOTS('',3,(#273889,#273890,#273891,#273892,#273893,
#273894,#273895,#273896,#273897,#273898),.UNSPECIFIED.,.F.,.F.,(4,3,3,4),
(0.00710274396181582,0.00747376592129673,0.0078350270594336,0.0080183686365081),
 .UNSPECIFIED.);
#6564=B_SPLINE_CURVE_WITH_KNOTS('',3,(#273902,#273903,#273904,#273905,#273906,
#273907,#273908,#273909),.UNSPECIFIED.,.F.,.F.,(4,2,2,4),(-5.73653316281769,
-5.7204734715418,-5.2879611244709,-5.23617773822434),.UNSPECIFIED.);
#6565=B_SPLINE_CURVE_WITH_KNOTS('',3,(#273913,#273914,#273915,#273916,#273917,
#273918),.UNSPECIFIED.,.F.,.F.,(4,2,4),(-1.68738761875409,-1.63190661744378,
-1.18678936119327),.UNSPECIFIED.);
#6566=B_SPLINE_CURVE_WITH_KNOTS('',3,(#273919,#273920,#273921,#273922,#273923,
#273924,#273925,#273926,#273927,#273928),.UNSPECIFIED.,.F.,.F.,(4,3,3,4),
(0.00710274908733836,0.00747377283388781,0.00783503581067877,0.00801837364807989),
 .UNSPECIFIED.);
#6567=B_SPLINE_CURVE_WITH_KNOTS('',3,(#273929,#273930,#273931,#273932,#273933,
#273934),.UNSPECIFIED.,.F.,.F.,(4,2,4),(1.75167822398879,1.82489845096549,
1.84415950254423),.UNSPECIFIED.);
#6568=B_SPLINE_CURVE_WITH_KNOTS('',3,(#273937,#273938,#273939,#273940,#273941,
#273942,#273943,#273944),.UNSPECIFIED.,.F.,.F.,(4,2,2,4),(-5.73653316281731,
-5.72047347154143,-5.28796112447051,-5.23617773822395),.UNSPECIFIED.);
#6569=B_SPLINE_CURVE_WITH_KNOTS('',3,(#273947,#273948,#273949,#273950,#273951,
#273952),.UNSPECIFIED.,.F.,.F.,(4,2,4),(-1.68738761875397,-1.63190661744366,
-1.18678936119318),.UNSPECIFIED.);
#6570=B_SPLINE_CURVE_WITH_KNOTS('',3,(#273955,#273956,#273957,#273958,#273959,
#273960,#273961,#273962),.UNSPECIFIED.,.F.,.F.,(4,2,2,4),(-5.73653316281751,
-5.72047347154163,-5.28796112447074,-5.23617773822419),.UNSPECIFIED.);
#6571=B_SPLINE_CURVE_WITH_KNOTS('',3,(#273965,#273966,#273967,#273968,#273969,
#273970),.UNSPECIFIED.,.F.,.F.,(4,2,4),(-1.6873876187541,-1.63190661744379,
-1.18678936119324),.UNSPECIFIED.);
#6572=B_SPLINE_CURVE_WITH_KNOTS('',3,(#274137,#274138,#274139,#274140,#274141,
#274142),.UNSPECIFIED.,.F.,.F.,(4,2,4),(-1.68738761875416,-1.63190661744385,
-1.18678936119333),.UNSPECIFIED.);
#6573=B_SPLINE_CURVE_WITH_KNOTS('',3,(#274144,#274145,#274146,#274147,#274148,
#274149,#274150,#274151,#274152,#274153),.UNSPECIFIED.,.F.,.F.,(4,3,3,4),
(0.00710274596862211,0.00747376540693313,0.00783502386849516,0.00801837063754701),
 .UNSPECIFIED.);
#6574=B_SPLINE_CURVE_WITH_KNOTS('',3,(#274157,#274158,#274159,#274160),
 .UNSPECIFIED.,.F.,.F.,(4,4),(0.673390429676812,0.765903724831544),
 .UNSPECIFIED.);
#6575=B_SPLINE_CURVE_WITH_KNOTS('',3,(#274161,#274162,#274163,#274164,#274165,
#274166,#274167,#274168),.UNSPECIFIED.,.F.,.F.,(4,2,2,4),(-5.73653316281784,
-5.72047347154196,-5.287961124471,-5.23617773822444),.UNSPECIFIED.);
#6576=B_SPLINE_CURVE_WITH_KNOTS('',3,(#274172,#274173,#274174,#274175),
 .UNSPECIFIED.,.F.,.F.,(4,4),(0.673390429666292,0.765903724818824),
 .UNSPECIFIED.);
#6577=B_SPLINE_CURVE_WITH_KNOTS('',3,(#274176,#274177,#274178,#274179,#274180,
#274181,#274182,#274183),.UNSPECIFIED.,.F.,.F.,(4,2,2,4),(-5.73653316281748,
-5.7204734715416,-5.28796112447073,-5.23617773822417),.UNSPECIFIED.);
#6578=B_SPLINE_CURVE_WITH_KNOTS('',3,(#274185,#274186,#274187,#274188,#274189,
#274190),.UNSPECIFIED.,.F.,.F.,(4,2,4),(-1.68738761875411,-1.63190661744379,
-1.18678936119327),.UNSPECIFIED.);
#6579=B_SPLINE_CURVE_WITH_KNOTS('',3,(#274192,#274193,#274194,#274195,#274196,
#274197,#274198,#274199,#274200,#274201),.UNSPECIFIED.,.F.,.F.,(4,3,3,4),
(0.0071027909646029,0.00747379949021994,0.00783504604206349,0.00801841495400679),
 .UNSPECIFIED.);
#6580=B_SPLINE_CURVE_WITH_KNOTS('',3,(#274206,#274207,#274208,#274209),
 .UNSPECIFIED.,.F.,.F.,(4,4),(0.673390429691577,0.765903724849725),
 .UNSPECIFIED.);
#6581=B_SPLINE_CURVE_WITH_KNOTS('',3,(#274210,#274211,#274212,#274213,#274214,
#274215,#274216,#274217),.UNSPECIFIED.,.F.,.F.,(4,2,2,4),(-5.73653316281866,
-5.72047347154278,-5.28796112447173,-5.23617773822516),.UNSPECIFIED.);
#6582=B_SPLINE_CURVE_WITH_KNOTS('',3,(#274219,#274220,#274221,#274222,#274223,
#274224),.UNSPECIFIED.,.F.,.F.,(4,2,4),(-1.68738761875417,-1.63190661744386,
-1.18678936119332),.UNSPECIFIED.);
#6583=B_SPLINE_CURVE_WITH_KNOTS('',3,(#274226,#274227,#274228,#274229,#274230,
#274231,#274232,#274233,#274234,#274235),.UNSPECIFIED.,.F.,.F.,(4,3,3,4),
(0.00710276617990406,0.00747378388368516,0.00783504033543666,0.00801839050540092),
 .UNSPECIFIED.);
#6584=B_SPLINE_CURVE_WITH_KNOTS('',3,(#274240,#274241,#274242,#274243),
 .UNSPECIFIED.,.F.,.F.,(4,4),(0.673390429669713,0.765903724823031),
 .UNSPECIFIED.);
#6585=B_SPLINE_CURVE_WITH_KNOTS('',3,(#274244,#274245,#274246,#274247,#274248,
#274249,#274250,#274251),.UNSPECIFIED.,.F.,.F.,(4,2,2,4),(-5.73653316281874,
-5.72047347154286,-5.2879611244718,-5.23617773822523),.UNSPECIFIED.);
#6586=B_SPLINE_CURVE_WITH_KNOTS('',3,(#274253,#274254,#274255,#274256,#274257,
#274258),.UNSPECIFIED.,.F.,.F.,(4,2,4),(-1.68738761875415,-1.63190661744384,
-1.1867893611933),.UNSPECIFIED.);
#6587=B_SPLINE_CURVE_WITH_KNOTS('',3,(#274260,#274261,#274262,#274263,#274264,
#274265,#274266,#274267,#274268,#274269),.UNSPECIFIED.,.F.,.F.,(4,3,3,4),
(0.00710275267632021,0.0074737751228719,0.00783503669673661,0.00801837718804212),
 .UNSPECIFIED.);
#6588=B_SPLINE_CURVE_WITH_KNOTS('',3,(#274273,#274274,#274275,#274276,#274277,
#274278),.UNSPECIFIED.,.F.,.F.,(4,2,4),(-1.68738761875413,-1.63190661744382,
-1.18678936119329),.UNSPECIFIED.);
#6589=B_SPLINE_CURVE_WITH_KNOTS('',3,(#274280,#274281,#274282,#274283,#274284,
#274285,#274286,#274287,#274288,#274289),.UNSPECIFIED.,.F.,.F.,(4,3,3,4),
(0.00710274287152854,0.00747376729108694,0.00783503103322807,0.00801836753620372),
 .UNSPECIFIED.);
#6590=B_SPLINE_CURVE_WITH_KNOTS('',3,(#274293,#274294,#274295,#274296),
 .UNSPECIFIED.,.F.,.F.,(4,4),(0.673390429683854,0.765903724840037),
 .UNSPECIFIED.);
#6591=B_SPLINE_CURVE_WITH_KNOTS('',3,(#274297,#274298,#274299,#274300,#274301,
#274302,#274303,#274304),.UNSPECIFIED.,.F.,.F.,(4,2,2,4),(-5.73653316281854,
-5.72047347154266,-5.28796112447161,-5.23617773822503),.UNSPECIFIED.);
#6592=B_SPLINE_CURVE_WITH_KNOTS('',3,(#274307,#274308,#274309,#274310),
 .UNSPECIFIED.,.F.,.F.,(4,4),(0.673390429668841,0.765903724822033),
 .UNSPECIFIED.);
#6593=B_SPLINE_CURVE_WITH_KNOTS('',3,(#274312,#274313,#274314,#274315,#274316,
#274317),.UNSPECIFIED.,.F.,.F.,(4,2,4),(-1.68738761875431,-1.63190661744399,
-1.18678936119339),.UNSPECIFIED.);
#6594=B_SPLINE_CURVE_WITH_KNOTS('',3,(#274319,#274320,#274321,#274322,#274323,
#274324,#274325,#274326,#274327,#274328),.UNSPECIFIED.,.F.,.F.,(4,3,3,4),
(0.00710274396181585,0.00747376592127879,0.00783502705942774,0.00801836863650806),
 .UNSPECIFIED.);
#6595=B_SPLINE_CURVE_WITH_KNOTS('',3,(#274333,#274334,#274335,#274336),
 .UNSPECIFIED.,.F.,.F.,(4,4),(0.673390429663607,0.765903724815473),
 .UNSPECIFIED.);
#6596=B_SPLINE_CURVE_WITH_KNOTS('',3,(#274337,#274338,#274339,#274340,#274341,
#274342,#274343,#274344),.UNSPECIFIED.,.F.,.F.,(4,2,2,4),(-5.73653316281882,
-5.72047347154294,-5.28796112447192,-5.23617773822535),.UNSPECIFIED.);
#6597=B_SPLINE_CURVE_WITH_KNOTS('',3,(#274346,#274347,#274348,#274349,#274350,
#274351),.UNSPECIFIED.,.F.,.F.,(4,2,4),(-1.68738761875414,-1.63190661744383,
-1.18678936119329),.UNSPECIFIED.);
#6598=B_SPLINE_CURVE_WITH_KNOTS('',3,(#274353,#274354,#274355,#274356,#274357,
#274358,#274359,#274360,#274361,#274362),.UNSPECIFIED.,.F.,.F.,(4,3,3,4),
(0.0071027455615668,0.0074737700644107,0.00783503387028777,0.00801837017674507),
 .UNSPECIFIED.);
#6599=B_SPLINE_CURVE_WITH_KNOTS('',3,(#274366,#274367,#274368,#274369,#274370,
#274371),.UNSPECIFIED.,.F.,.F.,(4,2,4),(-1.68738761875419,-1.63190661744387,
-1.18678936119332),.UNSPECIFIED.);
#6600=B_SPLINE_CURVE_WITH_KNOTS('',3,(#274373,#274374,#274375,#274376,#274377,
#274378,#274379,#274380,#274381,#274382),.UNSPECIFIED.,.F.,.F.,(4,3,3,4),
(0.00710274908733838,0.00747377283384765,0.00783503581062305,0.00801837364807991),
 .UNSPECIFIED.);
#6601=B_SPLINE_CURVE_WITH_KNOTS('',3,(#274386,#274387,#274388,#274389),
 .UNSPECIFIED.,.F.,.F.,(4,4),(0.673390429687081,0.765903724844288),
 .UNSPECIFIED.);
#6602=B_SPLINE_CURVE_WITH_KNOTS('',3,(#274390,#274391,#274392,#274393,#274394,
#274395,#274396,#274397),.UNSPECIFIED.,.F.,.F.,(4,2,2,4),(-5.73653316281885,
-5.72047347154297,-5.28796112447191,-5.23617773822534),.UNSPECIFIED.);
#6603=B_SPLINE_CURVE_WITH_KNOTS('',3,(#274401,#274402,#274403,#274404),
 .UNSPECIFIED.,.F.,.F.,(4,4),(0.673390432246977,0.765903727957335),
 .UNSPECIFIED.);
#6604=B_SPLINE_CURVE_WITH_KNOTS('',3,(#274405,#274406,#274407,#274408,#274409,
#274410,#274411,#274412),.UNSPECIFIED.,.F.,.F.,(4,2,2,4),(-5.73653316281879,
-5.72047347154291,-5.28796112447184,-5.23617773822526),.UNSPECIFIED.);
#6605=B_SPLINE_CURVE_WITH_KNOTS('',3,(#274414,#274415,#274416,#274417,#274418,
#274419),.UNSPECIFIED.,.F.,.F.,(4,2,4),(-1.68738761875414,-1.63190661744383,
-1.1867893611933),.UNSPECIFIED.);
#6606=B_SPLINE_CURVE_WITH_KNOTS('',3,(#274421,#274422,#274423,#274424,#274425,
#274426,#274427,#274428,#274429,#274430),.UNSPECIFIED.,.F.,.F.,(4,3,3,4),
(0.00710281114521608,0.00747381210005874,0.00783505048828664,0.00801843486213951),
 .UNSPECIFIED.);
#6607=B_SPLINE_CURVE_WITH_KNOTS('',3,(#274435,#274436,#274437,#274438),
 .UNSPECIFIED.,.F.,.F.,(4,4),(0.673390429686447,0.765903724843666),
 .UNSPECIFIED.);
#6608=B_SPLINE_CURVE_WITH_KNOTS('',3,(#274439,#274440,#274441,#274442,#274443,
#274444,#274445,#274446),.UNSPECIFIED.,.F.,.F.,(4,2,2,4),(-5.7365331628184,
-5.72047347154252,-5.28796112447152,-5.23617773822495),.UNSPECIFIED.);
#6609=B_SPLINE_CURVE_WITH_KNOTS('',3,(#274448,#274449,#274450,#274451,#274452,
#274453,#274454,#274455,#274456,#274457),.UNSPECIFIED.,.F.,.F.,(4,3,3,4),
(0.00710277664195233,0.00747379050279132,0.00783504280857186,0.00801840082520103),
 .UNSPECIFIED.);
#6610=B_SPLINE_CURVE_WITH_KNOTS('',3,(#274461,#274462,#274463,#274464,#274465,
#274466),.UNSPECIFIED.,.F.,.F.,(4,2,4),(-1.68738761875411,-1.6319066174438,
-1.18678936119329),.UNSPECIFIED.);
#6611=B_SPLINE_CURVE_WITH_KNOTS('',3,(#274468,#274469,#274470,#274471,#274472,
#274473,#274474,#274475,#274476,#274477),.UNSPECIFIED.,.F.,.F.,(4,3,3,4),
(0.00710275842609585,0.00747377890659939,0.0078350383557556,0.00801838285788014),
 .UNSPECIFIED.);
#6612=B_SPLINE_CURVE_WITH_KNOTS('',3,(#274481,#274482,#274483,#274484),
 .UNSPECIFIED.,.F.,.F.,(4,4),(0.673390432223755,0.765903727929032),
 .UNSPECIFIED.);
#6613=B_SPLINE_CURVE_WITH_KNOTS('',3,(#274485,#274486,#274487,#274488,#274489,
#274490,#274491,#274492),.UNSPECIFIED.,.F.,.F.,(4,2,2,4),(-5.73653316281933,
-5.72047347154344,-5.28796112447234,-5.23617773822576),.UNSPECIFIED.);
#6614=B_SPLINE_CURVE_WITH_KNOTS('',3,(#274496,#274497,#274498,#274499),
 .UNSPECIFIED.,.F.,.F.,(4,4),(0.673390429678433,0.765903724833911),
 .UNSPECIFIED.);
#6615=B_SPLINE_CURVE_WITH_KNOTS('',3,(#274500,#274501,#274502,#274503,#274504,
#274505,#274506,#274507),.UNSPECIFIED.,.F.,.F.,(4,2,2,4),(-5.73653316281869,
-5.7204734715428,-5.28796112447175,-5.23617773822517),.UNSPECIFIED.);
#6616=B_SPLINE_CURVE_WITH_KNOTS('',3,(#274509,#274510,#274511,#274512,#274513,
#274514),.UNSPECIFIED.,.F.,.F.,(4,2,4),(-1.68738761875428,-1.63190661744396,
-1.1867893611934),.UNSPECIFIED.);
#6617=B_SPLINE_CURVE_WITH_KNOTS('',3,(#274516,#274517,#274518,#274519,#274520,
#274521,#274522,#274523,#274524,#274525),.UNSPECIFIED.,.F.,.F.,(4,3,3,4),
(0.00710274848401432,0.00747377224140442,0.00783503523505279,0.00801837305550079),
 .UNSPECIFIED.);
#6618=B_SPLINE_CURVE_WITH_KNOTS('',3,(#274529,#274530,#274531,#274532,#274533,
#274534),.UNSPECIFIED.,.F.,.F.,(4,2,4),(-1.68738761875434,-1.63190661744402,
-1.18678936119343),.UNSPECIFIED.);
#6619=B_SPLINE_CURVE_WITH_KNOTS('',3,(#274536,#274537,#274538,#274539,#274540,
#274541,#274542,#274543,#274544,#274545),.UNSPECIFIED.,.F.,.F.,(4,3,3,4),
(0.00710274372650068,0.00747376845073826,0.00783503250649141,0.0080183683720891),
 .UNSPECIFIED.);
#6620=B_SPLINE_CURVE_WITH_KNOTS('',3,(#274549,#274550,#274551,#274552),
 .UNSPECIFIED.,.F.,.F.,(4,4),(0.673390427101013,0.765903721698924),
 .UNSPECIFIED.);
#6621=B_SPLINE_CURVE_WITH_KNOTS('',3,(#274553,#274554,#274555,#274556,#274557,
#274558,#274559,#274560),.UNSPECIFIED.,.F.,.F.,(4,2,2,4),(-5.73653316281909,
-5.7204734715432,-5.28796112447211,-5.23617773822553),.UNSPECIFIED.);
#6622=B_SPLINE_CURVE_WITH_KNOTS('',3,(#274564,#274565,#274566,#274567),
 .UNSPECIFIED.,.F.,.F.,(4,4),(0.673390429693342,0.765903724851547),
 .UNSPECIFIED.);
#6623=B_SPLINE_CURVE_WITH_KNOTS('',3,(#274568,#274569,#274570,#274571,#274572,
#274573,#274574,#274575),.UNSPECIFIED.,.F.,.F.,(4,2,2,4),(-5.73653316281968,
-5.72047347154379,-5.28796112447263,-5.23617773822604),.UNSPECIFIED.);
#6624=B_SPLINE_CURVE_WITH_KNOTS('',3,(#274577,#274578,#274579,#274580,#274581,
#274582),.UNSPECIFIED.,.F.,.F.,(4,2,4),(-1.68738761875421,-1.6319066174439,
-1.18678936119335),.UNSPECIFIED.);
#6625=B_SPLINE_CURVE_WITH_KNOTS('',3,(#274584,#274585,#274586,#274587,#274588,
#274589,#274590,#274591,#274592,#274593),.UNSPECIFIED.,.F.,.F.,(4,3,3,4),
(0.00710274294853989,0.00747376648671073,0.0078350292986873,0.00801836762245744),
 .UNSPECIFIED.);
#6626=B_SPLINE_CURVE_WITH_KNOTS('',3,(#274596,#274597,#274598,#274599,#274600,
#274601),.UNSPECIFIED.,.F.,.F.,(4,2,4),(-1.68738761875434,-1.63190661744402,
-1.18678936119342),.UNSPECIFIED.);
#6627=B_SPLINE_CURVE_WITH_KNOTS('',3,(#274603,#274604,#274605,#274606,#274607,
#274608,#274609,#274610),.UNSPECIFIED.,.F.,.F.,(4,2,2,4),(-5.73653316282004,
-5.72047347154415,-5.28796112447295,-5.23617773822635),.UNSPECIFIED.);
#6628=B_SPLINE_CURVE_WITH_KNOTS('',3,(#274612,#274613,#274614,#274615,#274616,
#274617,#274618,#274619),.UNSPECIFIED.,.F.,.F.,(4,2,2,4),(-5.73653316281866,
-5.72047347154277,-5.28796112447173,-5.23617773822515),.UNSPECIFIED.);
#6629=B_SPLINE_CURVE_WITH_KNOTS('',3,(#274620,#274621,#274622,#274623,#274624,
#274625),.UNSPECIFIED.,.F.,.F.,(4,2,4),(-1.68738761875433,-1.63190661744401,
-1.18678936119343),.UNSPECIFIED.);
#6630=B_SPLINE_CURVE_WITH_KNOTS('',3,(#274628,#274629,#274630,#274631,#274632,
#274633,#274634,#274635),.UNSPECIFIED.,.F.,.F.,(4,2,2,4),(-5.73653316281802,
-5.72047347154213,-5.28796112447117,-5.23617773822461),.UNSPECIFIED.);
#6631=B_SPLINE_CURVE_WITH_KNOTS('',3,(#274636,#274637,#274638,#274639,#274640,
#274641),.UNSPECIFIED.,.F.,.F.,(4,2,4),(-1.68738761875432,-1.631906617444,
-1.18678936119341),.UNSPECIFIED.);
#6632=B_SPLINE_CURVE_WITH_KNOTS('',3,(#274644,#274645,#274646,#274647,#274648,
#274649),.UNSPECIFIED.,.F.,.F.,(4,2,4),(-1.68738761875423,-1.63190661744392,
-1.18678936119335),.UNSPECIFIED.);
#6633=B_SPLINE_CURVE_WITH_KNOTS('',3,(#274651,#274652,#274653,#274654,#274655,
#274656,#274657,#274658),.UNSPECIFIED.,.F.,.F.,(4,2,2,4),(-5.73653316281873,
-5.72047347154284,-5.2879611244718,-5.23617773822523),.UNSPECIFIED.);
#6634=B_SPLINE_CURVE_WITH_KNOTS('',3,(#274660,#274661,#274662,#274663,#274664,
#274665,#274666,#274667),.UNSPECIFIED.,.F.,.F.,(4,2,2,4),(-5.7365331628187,
-5.72047347154281,-5.28796112447176,-5.2361777382252),.UNSPECIFIED.);
#6635=B_SPLINE_CURVE_WITH_KNOTS('',3,(#274668,#274669,#274670,#274671,#274672,
#274673),.UNSPECIFIED.,.F.,.F.,(4,2,4),(-1.6873876187541,-1.63190661744378,
-1.18678936119327),.UNSPECIFIED.);
#6636=B_SPLINE_CURVE_WITH_KNOTS('',3,(#274676,#274677,#274678,#274679,#274680,
#274681),.UNSPECIFIED.,.F.,.F.,(4,2,4),(-1.68738761875444,-1.63190661744411,
-1.18678936119347),.UNSPECIFIED.);
#6637=B_SPLINE_CURVE_WITH_KNOTS('',3,(#274683,#274684,#274685,#274686,#274687,
#274688,#274689,#274690),.UNSPECIFIED.,.F.,.F.,(4,2,2,4),(-5.73653316281952,
-5.72047347154364,-5.2879611244725,-5.23617773822591),.UNSPECIFIED.);
#6638=B_SPLINE_CURVE_WITH_KNOTS('',3,(#274692,#274693,#274694,#274695,#274696,
#274697,#274698,#274699),.UNSPECIFIED.,.F.,.F.,(4,2,2,4),(-5.73653316281812,
-5.72047347154224,-5.28796112447125,-5.23617773822468),.UNSPECIFIED.);
#6639=B_SPLINE_CURVE_WITH_KNOTS('',3,(#274701,#274702,#274703,#274704,#274705,
#274706),.UNSPECIFIED.,.F.,.F.,(4,2,4),(-1.68738761875419,-1.63190661744387,
-1.18678936119332),.UNSPECIFIED.);
#6640=B_SPLINE_CURVE_WITH_KNOTS('',3,(#274708,#274709,#274710,#274711,#274712,
#274713,#274714,#274715,#274716,#274717),.UNSPECIFIED.,.F.,.F.,(4,3,3,4),
(0.00710274396181585,0.0074737659213073,0.00783502705945658,0.00801836863650807),
 .UNSPECIFIED.);
#6641=B_SPLINE_CURVE_WITH_KNOTS('',3,(#274720,#274721,#274722,#274723,#274724,
#274725),.UNSPECIFIED.,.F.,.F.,(4,2,4),(-1.68738761875417,-1.63190661744386,
-1.18678936119332),.UNSPECIFIED.);
#6642=B_SPLINE_CURVE_WITH_KNOTS('',3,(#274727,#274728,#274729,#274730,#274731,
#274732,#274733,#274734),.UNSPECIFIED.,.F.,.F.,(4,2,2,4),(-5.73653316282042,
-5.72047347154453,-5.28796112447321,-5.2361777382266),.UNSPECIFIED.);
#6643=B_SPLINE_CURVE_WITH_KNOTS('',3,(#274736,#274737,#274738,#274739,#274740,
#274741,#274742,#274743),.UNSPECIFIED.,.F.,.F.,(4,2,2,4),(-5.73653316281903,
-5.72047347154315,-5.28796112447213,-5.23617773822556),.UNSPECIFIED.);
#6644=B_SPLINE_CURVE_WITH_KNOTS('',3,(#274744,#274745,#274746,#274747,#274748,
#274749),.UNSPECIFIED.,.F.,.F.,(4,2,4),(-1.68738761875402,-1.63190661744372,
-1.18678936119324),.UNSPECIFIED.);
#6645=B_SPLINE_CURVE_WITH_KNOTS('',3,(#274752,#274753,#274754,#274755,#274756,
#274757,#274758,#274759),.UNSPECIFIED.,.F.,.F.,(4,2,2,4),(-5.73653316282014,
-5.72047347154425,-5.28796112447299,-5.23617773822639),.UNSPECIFIED.);
#6646=B_SPLINE_CURVE_WITH_KNOTS('',3,(#274760,#274761,#274762,#274763,#274764,
#274765),.UNSPECIFIED.,.F.,.F.,(4,2,4),(-1.68738761875435,-1.63190661744403,
-1.18678936119343),.UNSPECIFIED.);
#6647=B_SPLINE_CURVE_WITH_KNOTS('',3,(#274768,#274769,#274770,#274771,#274772,
#274773),.UNSPECIFIED.,.F.,.F.,(4,2,4),(-1.6873876187543,-1.63190661744398,
-1.1867893611934),.UNSPECIFIED.);
#6648=B_SPLINE_CURVE_WITH_KNOTS('',3,(#274777,#274778,#274779,#274780),
 .UNSPECIFIED.,.F.,.F.,(4,4),(0.673390429688366,0.765903724845993),
 .UNSPECIFIED.);
#6649=B_SPLINE_CURVE_WITH_KNOTS('',3,(#274781,#274782,#274783,#274784,#274785,
#274786,#274787,#274788),.UNSPECIFIED.,.F.,.F.,(4,2,2,4),(-5.73653316281831,
-5.72047347154242,-5.28796112447148,-5.23617773822492),.UNSPECIFIED.);
#6650=B_SPLINE_CURVE_WITH_KNOTS('',3,(#274791,#274792,#274793,#274794,#274795,
#274796),.UNSPECIFIED.,.F.,.F.,(4,2,4),(-1.68738761875411,-1.6319066174438,
-1.18678936119327),.UNSPECIFIED.);
#6651=B_SPLINE_CURVE_WITH_KNOTS('',3,(#274798,#274799,#274800,#274801,#274802,
#274803,#274804,#274805,#274806,#274807),.UNSPECIFIED.,.F.,.F.,(4,3,3,4),
(0.00710281114521606,0.00747381210002463,0.00783505048825559,0.00801843486213951),
 .UNSPECIFIED.);
#6652=B_SPLINE_CURVE_WITH_KNOTS('',3,(#274811,#274812,#274813,#274814),
 .UNSPECIFIED.,.F.,.F.,(4,4),(0.673390429663033,0.765903724814501),
 .UNSPECIFIED.);
#6653=B_SPLINE_CURVE_WITH_KNOTS('',3,(#274815,#274816,#274817,#274818,#274819,
#274820,#274821,#274822),.UNSPECIFIED.,.F.,.F.,(4,2,2,4),(-5.73653316281795,
-5.72047347154207,-5.2879611244711,-5.23617773822453),.UNSPECIFIED.);
#6654=B_SPLINE_CURVE_WITH_KNOTS('',3,(#274824,#274825,#274826,#274827,#274828,
#274829,#274830,#274831),.UNSPECIFIED.,.F.,.F.,(4,2,2,4),(-5.73653316281885,
-5.72047347154296,-5.28796112447191,-5.23617773822534),.UNSPECIFIED.);
#6655=B_SPLINE_CURVE_WITH_KNOTS('',3,(#274832,#274833,#274834,#274835,#274836,
#274837),.UNSPECIFIED.,.F.,.F.,(4,2,4),(-1.68738761875433,-1.63190661744402,
-1.18678936119343),.UNSPECIFIED.);
#6656=B_SPLINE_CURVE_WITH_KNOTS('',3,(#274840,#274841,#274842,#274843,#274844,
#274845,#274846,#274847),.UNSPECIFIED.,.F.,.F.,(4,2,2,4),(-5.73653316281845,
-5.72047347154257,-5.28796112447156,-5.23617773822498),.UNSPECIFIED.);
#6657=B_SPLINE_CURVE_WITH_KNOTS('',3,(#274848,#274849,#274850,#274851,#274852,
#274853),.UNSPECIFIED.,.F.,.F.,(4,2,4),(-1.6873876187544,-1.63190661744407,
-1.18678936119345),.UNSPECIFIED.);
#6658=B_SPLINE_CURVE_WITH_KNOTS('',3,(#274857,#274858,#274859,#274860,#274861,
#274862,#274863,#274864,#274865,#274866),.UNSPECIFIED.,.F.,.F.,(4,3,3,4),
(0.00710281114521603,0.00747381210002846,0.00783505048825458,0.00801843486213948),
 .UNSPECIFIED.);
#6659=B_SPLINE_CURVE_WITH_KNOTS('',3,(#274868,#274869,#274870,#274871,#274872,
#274873),.UNSPECIFIED.,.F.,.F.,(4,2,4),(1.75167822400075,1.82489845097847,
1.84415950255741),.UNSPECIFIED.);
#6660=B_SPLINE_CURVE_WITH_KNOTS('',3,(#274875,#274876,#274877,#274878,#274879,
#274880,#274881,#274882),.UNSPECIFIED.,.F.,.F.,(4,2,2,4),(-5.73653316281845,
-5.72047347154257,-5.28796112447152,-5.23617773822495),.UNSPECIFIED.);
#6661=B_SPLINE_CURVE_WITH_KNOTS('',3,(#274885,#274886,#274887,#274888,#274889,
#274890),.UNSPECIFIED.,.F.,.F.,(4,2,4),(-1.68738761875408,-1.63190661744377,
-1.18678936119327),.UNSPECIFIED.);
#6662=B_SPLINE_CURVE_WITH_KNOTS('',3,(#274900,#274901,#274902,#274903),
 .UNSPECIFIED.,.F.,.F.,(4,4),(0.673390429683733,0.765903724840068),
 .UNSPECIFIED.);
#6663=B_SPLINE_CURVE_WITH_KNOTS('',3,(#274904,#274905,#274906,#274907,#274908,
#274909,#274910,#274911),.UNSPECIFIED.,.F.,.F.,(4,2,2,4),(-5.73653316281842,
-5.72047347154254,-5.28796112447156,-5.236177738225),.UNSPECIFIED.);
#6664=B_SPLINE_CURVE_WITH_KNOTS('',3,(#274913,#274914,#274915,#274916,#274917,
#274918),.UNSPECIFIED.,.F.,.F.,(4,2,4),(-1.68738761875398,-1.63190661744368,
-1.18678936119318),.UNSPECIFIED.);
#6665=B_SPLINE_CURVE_WITH_KNOTS('',3,(#274920,#274921,#274922,#274923,#274924,
#274925,#274926,#274927,#274928,#274929),.UNSPECIFIED.,.F.,.F.,(4,3,3,4),
(0.00710274908733839,0.0074737728338415,0.00783503581060294,0.00801837364807991),
 .UNSPECIFIED.);
#7227=SHAPE_REPRESENTATION_RELATIONSHIP('SRR','None',#310900,#7244);
#7244=ADVANCED_BREP_SHAPE_REPRESENTATION('',(#7349),#310609);
#7281=STYLED_ITEM('',(#311003),#7349);
#7349=MANIFOLD_SOLID_BREP('Body1',#93731);
#7627=FACE_BOUND('',#19737,.T.);
#7628=FACE_BOUND('',#19739,.T.);
#7629=FACE_BOUND('',#19828,.T.);
#8535=PLANE('',#103602);
#8536=PLANE('',#103650);
#8537=PLANE('',#103825);
#8538=PLANE('',#103920);
#8539=PLANE('',#103921);
#8540=PLANE('',#103922);
#13741=FACE_OUTER_BOUND('',#19716,.T.);
#13742=FACE_OUTER_BOUND('',#19717,.T.);
#13743=FACE_OUTER_BOUND('',#19718,.T.);
#13744=FACE_OUTER_BOUND('',#19719,.T.);
#13745=FACE_OUTER_BOUND('',#19720,.T.);
#13746=FACE_OUTER_BOUND('',#19721,.T.);
#13747=FACE_OUTER_BOUND('',#19722,.T.);
#13748=FACE_OUTER_BOUND('',#19723,.T.);
#13749=FACE_OUTER_BOUND('',#19724,.T.);
#13750=FACE_OUTER_BOUND('',#19725,.T.);
#13751=FACE_OUTER_BOUND('',#19726,.T.);
#13752=FACE_OUTER_BOUND('',#19727,.T.);
#13753=FACE_OUTER_BOUND('',#19728,.T.);
#13754=FACE_OUTER_BOUND('',#19729,.T.);
#13755=FACE_OUTER_BOUND('',#19730,.T.);
#13756=FACE_OUTER_BOUND('',#19731,.T.);
#13757=FACE_OUTER_BOUND('',#19732,.T.);
#13758=FACE_OUTER_BOUND('',#19733,.T.);
#13759=FACE_OUTER_BOUND('',#19734,.T.);
#13760=FACE_OUTER_BOUND('',#19735,.T.);
#13761=FACE_OUTER_BOUND('',#19736,.T.);
#13762=FACE_OUTER_BOUND('',#19738,.T.);
#13763=FACE_OUTER_BOUND('',#19740,.T.);
#13764=FACE_OUTER_BOUND('',#19741,.T.);
#13765=FACE_OUTER_BOUND('',#19742,.T.);
#13766=FACE_OUTER_BOUND('',#19743,.T.);
#13767=FACE_OUTER_BOUND('',#19744,.T.);
#13768=FACE_OUTER_BOUND('',#19745,.T.);
#13769=FACE_OUTER_BOUND('',#19746,.T.);
#13770=FACE_OUTER_BOUND('',#19747,.T.);
#13771=FACE_OUTER_BOUND('',#19748,.T.);
#13772=FACE_OUTER_BOUND('',#19749,.T.);
#13773=FACE_OUTER_BOUND('',#19750,.T.);
#13774=FACE_OUTER_BOUND('',#19751,.T.);
#13775=FACE_OUTER_BOUND('',#19752,.T.);
#13776=FACE_OUTER_BOUND('',#19753,.T.);
#13777=FACE_OUTER_BOUND('',#19754,.T.);
#13778=FACE_OUTER_BOUND('',#19755,.T.);
#13779=FACE_OUTER_BOUND('',#19756,.T.);
#13780=FACE_OUTER_BOUND('',#19757,.T.);
#13781=FACE_OUTER_BOUND('',#19758,.T.);
#13782=FACE_OUTER_BOUND('',#19759,.T.);
#13783=FACE_OUTER_BOUND('',#19760,.T.);
#13784=FACE_OUTER_BOUND('',#19761,.T.);
#13785=FACE_OUTER_BOUND('',#19762,.T.);
#13786=FACE_OUTER_BOUND('',#19763,.T.);
#13787=FACE_OUTER_BOUND('',#19764,.T.);
#13788=FACE_OUTER_BOUND('',#19765,.T.);
#13789=FACE_OUTER_BOUND('',#19766,.T.);
#13790=FACE_OUTER_BOUND('',#19767,.T.);
#13791=FACE_OUTER_BOUND('',#19768,.T.);
#13792=FACE_OUTER_BOUND('',#19769,.T.);
#13793=FACE_OUTER_BOUND('',#19770,.T.);
#13794=FACE_OUTER_BOUND('',#19771,.T.);
#13795=FACE_OUTER_BOUND('',#19772,.T.);
#13796=FACE_OUTER_BOUND('',#19773,.T.);
#13797=FACE_OUTER_BOUND('',#19774,.T.);
#13798=FACE_OUTER_BOUND('',#19775,.T.);
#13799=FACE_OUTER_BOUND('',#19776,.T.);
#13800=FACE_OUTER_BOUND('',#19777,.T.);
#13801=FACE_OUTER_BOUND('',#19778,.T.);
#13802=FACE_OUTER_BOUND('',#19779,.T.);
#13803=FACE_OUTER_BOUND('',#19780,.T.);
#13804=FACE_OUTER_BOUND('',#19781,.T.);
#13805=FACE_OUTER_BOUND('',#19782,.T.);
#13806=FACE_OUTER_BOUND('',#19783,.T.);
#13807=FACE_OUTER_BOUND('',#19784,.T.);
#13808=FACE_OUTER_BOUND('',#19785,.T.);
#13809=FACE_OUTER_BOUND('',#19786,.T.);
#13810=FACE_OUTER_BOUND('',#19787,.T.);
#13811=FACE_OUTER_BOUND('',#19788,.T.);
#13812=FACE_OUTER_BOUND('',#19789,.T.);
#13813=FACE_OUTER_BOUND('',#19790,.T.);
#13814=FACE_OUTER_BOUND('',#19791,.T.);
#13815=FACE_OUTER_BOUND('',#19792,.T.);
#13816=FACE_OUTER_BOUND('',#19793,.T.);
#13817=FACE_OUTER_BOUND('',#19794,.T.);
#13818=FACE_OUTER_BOUND('',#19795,.T.);
#13819=FACE_OUTER_BOUND('',#19796,.T.);
#13820=FACE_OUTER_BOUND('',#19797,.T.);
#13821=FACE_OUTER_BOUND('',#19798,.T.);
#13822=FACE_OUTER_BOUND('',#19799,.T.);
#13823=FACE_OUTER_BOUND('',#19800,.T.);
#13824=FACE_OUTER_BOUND('',#19801,.T.);
#13825=FACE_OUTER_BOUND('',#19802,.T.);
#13826=FACE_OUTER_BOUND('',#19803,.T.);
#13827=FACE_OUTER_BOUND('',#19804,.T.);
#13828=FACE_OUTER_BOUND('',#19805,.T.);
#13829=FACE_OUTER_BOUND('',#19806,.T.);
#13830=FACE_OUTER_BOUND('',#19807,.T.);
#13831=FACE_OUTER_BOUND('',#19808,.T.);
#13832=FACE_OUTER_BOUND('',#19809,.T.);
#13833=FACE_OUTER_BOUND('',#19810,.T.);
#13834=FACE_OUTER_BOUND('',#19811,.T.);
#13835=FACE_OUTER_BOUND('',#19812,.T.);
#13836=FACE_OUTER_BOUND('',#19813,.T.);
#13837=FACE_OUTER_BOUND('',#19814,.T.);
#13838=FACE_OUTER_BOUND('',#19815,.T.);
#13839=FACE_OUTER_BOUND('',#19816,.T.);
#13840=FACE_OUTER_BOUND('',#19817,.T.);
#13841=FACE_OUTER_BOUND('',#19818,.T.);
#13842=FACE_OUTER_BOUND('',#19819,.T.);
#13843=FACE_OUTER_BOUND('',#19820,.T.);
#13844=FACE_OUTER_BOUND('',#19821,.T.);
#13845=FACE_OUTER_BOUND('',#19822,.T.);
#13846=FACE_OUTER_BOUND('',#19823,.T.);
#13847=FACE_OUTER_BOUND('',#19824,.T.);
#13848=FACE_OUTER_BOUND('',#19825,.T.);
#13849=FACE_OUTER_BOUND('',#19826,.T.);
#13850=FACE_OUTER_BOUND('',#19827,.T.);
#13851=FACE_OUTER_BOUND('',#19829,.T.);
#13852=FACE_OUTER_BOUND('',#19830,.T.);
#13853=FACE_OUTER_BOUND('',#19831,.T.);
#13854=FACE_OUTER_BOUND('',#19832,.T.);
#13855=FACE_OUTER_BOUND('',#19833,.T.);
#13856=FACE_OUTER_BOUND('',#19834,.T.);
#13857=FACE_OUTER_BOUND('',#19835,.T.);
#13858=FACE_OUTER_BOUND('',#19836,.T.);
#13859=FACE_OUTER_BOUND('',#19837,.T.);
#13860=FACE_OUTER_BOUND('',#19838,.T.);
#13861=FACE_OUTER_BOUND('',#19839,.T.);
#13862=FACE_OUTER_BOUND('',#19840,.T.);
#13863=FACE_OUTER_BOUND('',#19841,.T.);
#13864=FACE_OUTER_BOUND('',#19842,.T.);
#13865=FACE_OUTER_BOUND('',#19843,.T.);
#13866=FACE_OUTER_BOUND('',#19844,.T.);
#13867=FACE_OUTER_BOUND('',#19845,.T.);
#13868=FACE_OUTER_BOUND('',#19846,.T.);
#13869=FACE_OUTER_BOUND('',#19847,.T.);
#13870=FACE_OUTER_BOUND('',#19848,.T.);
#13871=FACE_OUTER_BOUND('',#19849,.T.);
#13872=FACE_OUTER_BOUND('',#19850,.T.);
#13873=FACE_OUTER_BOUND('',#19851,.T.);
#13874=FACE_OUTER_BOUND('',#19852,.T.);
#13875=FACE_OUTER_BOUND('',#19853,.T.);
#13876=FACE_OUTER_BOUND('',#19854,.T.);
#13877=FACE_OUTER_BOUND('',#19855,.T.);
#13878=FACE_OUTER_BOUND('',#19856,.T.);
#13879=FACE_OUTER_BOUND('',#19857,.T.);
#13880=FACE_OUTER_BOUND('',#19858,.T.);
#13881=FACE_OUTER_BOUND('',#19859,.T.);
#13882=FACE_OUTER_BOUND('',#19860,.T.);
#13883=FACE_OUTER_BOUND('',#19861,.T.);
#13884=FACE_OUTER_BOUND('',#19862,.T.);
#13885=FACE_OUTER_BOUND('',#19863,.T.);
#13886=FACE_OUTER_BOUND('',#19864,.T.);
#13887=FACE_OUTER_BOUND('',#19865,.T.);
#13888=FACE_OUTER_BOUND('',#19866,.T.);
#13889=FACE_OUTER_BOUND('',#19867,.T.);
#13890=FACE_OUTER_BOUND('',#19868,.T.);
#13891=FACE_OUTER_BOUND('',#19869,.T.);
#13892=FACE_OUTER_BOUND('',#19870,.T.);
#13893=FACE_OUTER_BOUND('',#19871,.T.);
#13894=FACE_OUTER_BOUND('',#19872,.T.);
#13895=FACE_OUTER_BOUND('',#19873,.T.);
#13896=FACE_OUTER_BOUND('',#19874,.T.);
#13897=FACE_OUTER_BOUND('',#19875,.T.);
#13898=FACE_OUTER_BOUND('',#19876,.T.);
#13899=FACE_OUTER_BOUND('',#19877,.T.);
#13900=FACE_OUTER_BOUND('',#19878,.T.);
#13901=FACE_OUTER_BOUND('',#19879,.T.);
#13902=FACE_OUTER_BOUND('',#19880,.T.);
#13903=FACE_OUTER_BOUND('',#19881,.T.);
#13904=FACE_OUTER_BOUND('',#19882,.T.);
#13905=FACE_OUTER_BOUND('',#19883,.T.);
#13906=FACE_OUTER_BOUND('',#19884,.T.);
#13907=FACE_OUTER_BOUND('',#19885,.T.);
#13908=FACE_OUTER_BOUND('',#19886,.T.);
#13909=FACE_OUTER_BOUND('',#19887,.T.);
#13910=FACE_OUTER_BOUND('',#19888,.T.);
#13911=FACE_OUTER_BOUND('',#19889,.T.);
#13912=FACE_OUTER_BOUND('',#19890,.T.);
#13913=FACE_OUTER_BOUND('',#19891,.T.);
#13914=FACE_OUTER_BOUND('',#19892,.T.);
#13915=FACE_OUTER_BOUND('',#19893,.T.);
#13916=FACE_OUTER_BOUND('',#19894,.T.);
#13917=FACE_OUTER_BOUND('',#19895,.T.);
#13918=FACE_OUTER_BOUND('',#19896,.T.);
#13919=FACE_OUTER_BOUND('',#19897,.T.);
#13920=FACE_OUTER_BOUND('',#19898,.T.);
#13921=FACE_OUTER_BOUND('',#19899,.T.);
#13922=FACE_OUTER_BOUND('',#19900,.T.);
#13923=FACE_OUTER_BOUND('',#19901,.T.);
#13924=FACE_OUTER_BOUND('',#19902,.T.);
#13925=FACE_OUTER_BOUND('',#19903,.T.);
#13926=FACE_OUTER_BOUND('',#19904,.T.);
#13927=FACE_OUTER_BOUND('',#19905,.T.);
#13928=FACE_OUTER_BOUND('',#19906,.T.);
#13929=FACE_OUTER_BOUND('',#19907,.T.);
#19716=EDGE_LOOP('',(#82321,#82322,#82323,#82324));
#19717=EDGE_LOOP('',(#82325,#82326,#82327,#82328));
#19718=EDGE_LOOP('',(#82329,#82330,#82331,#82332));
#19719=EDGE_LOOP('',(#82333,#82334,#82335,#82336));
#19720=EDGE_LOOP('',(#82337,#82338,#82339,#82340,#82341,#82342,#82343,#82344));
#19721=EDGE_LOOP('',(#82345,#82346,#82347,#82348,#82349,#82350,#82351,#82352));
#19722=EDGE_LOOP('',(#82353,#82354,#82355,#82356,#82357,#82358,#82359,#82360));
#19723=EDGE_LOOP('',(#82361,#82362,#82363,#82364,#82365,#82366,#82367,#82368));
#19724=EDGE_LOOP('',(#82369,#82370,#82371,#82372,#82373,#82374,#82375,#82376));
#19725=EDGE_LOOP('',(#82377,#82378,#82379,#82380,#82381,#82382,#82383,#82384));
#19726=EDGE_LOOP('',(#82385,#82386,#82387,#82388,#82389,#82390,#82391,#82392));
#19727=EDGE_LOOP('',(#82393,#82394,#82395,#82396,#82397,#82398,#82399,#82400));
#19728=EDGE_LOOP('',(#82401,#82402,#82403,#82404,#82405,#82406,#82407,#82408));
#19729=EDGE_LOOP('',(#82409,#82410,#82411,#82412,#82413,#82414,#82415,#82416));
#19730=EDGE_LOOP('',(#82417,#82418,#82419,#82420,#82421,#82422,#82423,#82424));
#19731=EDGE_LOOP('',(#82425,#82426,#82427,#82428,#82429,#82430,#82431,#82432));
#19732=EDGE_LOOP('',(#82433,#82434,#82435,#82436,#82437,#82438));
#19733=EDGE_LOOP('',(#82439,#82440,#82441,#82442));
#19734=EDGE_LOOP('',(#82443,#82444,#82445,#82446,#82447,#82448));
#19735=EDGE_LOOP('',(#82449,#82450,#82451,#82452));
#19736=EDGE_LOOP('',(#82453,#82454,#82455,#82456,#82457,#82458,#82459,#82460,
#82461,#82462,#82463,#82464,#82465,#82466,#82467,#82468,#82469,#82470,#82471,
#82472,#82473,#82474,#82475,#82476,#82477,#82478,#82479,#82480,#82481,#82482,
#82483,#82484,#82485,#82486,#82487,#82488,#82489,#82490,#82491,#82492,#82493,
#82494,#82495,#82496,#82497,#82498,#82499,#82500,#82501,#82502,#82503,#82504,
#82505,#82506,#82507,#82508,#82509,#82510,#82511,#82512));
#19737=EDGE_LOOP('',(#82513,#82514,#82515,#82516));
#19738=EDGE_LOOP('',(#82517));
#19739=EDGE_LOOP('',(#82518,#82519,#82520,#82521));
#19740=EDGE_LOOP('',(#82522,#82523,#82524,#82525,#82526,#82527));
#19741=EDGE_LOOP('',(#82528,#82529,#82530,#82531,#82532,#82533));
#19742=EDGE_LOOP('',(#82534,#82535,#82536,#82537,#82538,#82539));
#19743=EDGE_LOOP('',(#82540,#82541,#82542,#82543,#82544,#82545));
#19744=EDGE_LOOP('',(#82546,#82547,#82548,#82549,#82550,#82551));
#19745=EDGE_LOOP('',(#82552,#82553,#82554,#82555,#82556,#82557));
#19746=EDGE_LOOP('',(#82558,#82559,#82560,#82561,#82562,#82563));
#19747=EDGE_LOOP('',(#82564,#82565,#82566,#82567,#82568,#82569));
#19748=EDGE_LOOP('',(#82570,#82571,#82572,#82573,#82574,#82575));
#19749=EDGE_LOOP('',(#82576,#82577,#82578,#82579,#82580,#82581));
#19750=EDGE_LOOP('',(#82582,#82583,#82584,#82585,#82586,#82587));
#19751=EDGE_LOOP('',(#82588,#82589,#82590,#82591,#82592,#82593));
#19752=EDGE_LOOP('',(#82594,#82595,#82596,#82597,#82598,#82599));
#19753=EDGE_LOOP('',(#82600,#82601,#82602,#82603,#82604,#82605));
#19754=EDGE_LOOP('',(#82606,#82607,#82608,#82609,#82610,#82611));
#19755=EDGE_LOOP('',(#82612,#82613,#82614,#82615,#82616,#82617));
#19756=EDGE_LOOP('',(#82618,#82619,#82620,#82621,#82622,#82623));
#19757=EDGE_LOOP('',(#82624,#82625,#82626,#82627,#82628,#82629));
#19758=EDGE_LOOP('',(#82630,#82631,#82632,#82633,#82634,#82635));
#19759=EDGE_LOOP('',(#82636,#82637,#82638,#82639,#82640,#82641));
#19760=EDGE_LOOP('',(#82642,#82643,#82644,#82645,#82646,#82647));
#19761=EDGE_LOOP('',(#82648,#82649,#82650,#82651,#82652,#82653));
#19762=EDGE_LOOP('',(#82654,#82655,#82656,#82657,#82658,#82659));
#19763=EDGE_LOOP('',(#82660,#82661,#82662,#82663,#82664,#82665));
#19764=EDGE_LOOP('',(#82666,#82667,#82668,#82669,#82670,#82671));
#19765=EDGE_LOOP('',(#82672,#82673,#82674,#82675,#82676,#82677));
#19766=EDGE_LOOP('',(#82678,#82679,#82680,#82681,#82682,#82683));
#19767=EDGE_LOOP('',(#82684,#82685,#82686,#82687,#82688,#82689));
#19768=EDGE_LOOP('',(#82690,#82691,#82692,#82693));
#19769=EDGE_LOOP('',(#82694,#82695,#82696,#82697));
#19770=EDGE_LOOP('',(#82698,#82699,#82700,#82701));
#19771=EDGE_LOOP('',(#82702,#82703,#82704,#82705));
#19772=EDGE_LOOP('',(#82706,#82707,#82708,#82709));
#19773=EDGE_LOOP('',(#82710,#82711,#82712,#82713));
#19774=EDGE_LOOP('',(#82714,#82715,#82716,#82717));
#19775=EDGE_LOOP('',(#82718,#82719,#82720,#82721));
#19776=EDGE_LOOP('',(#82722,#82723,#82724,#82725));
#19777=EDGE_LOOP('',(#82726,#82727,#82728,#82729));
#19778=EDGE_LOOP('',(#82730,#82731,#82732,#82733));
#19779=EDGE_LOOP('',(#82734,#82735,#82736,#82737));
#19780=EDGE_LOOP('',(#82738,#82739,#82740,#82741));
#19781=EDGE_LOOP('',(#82742,#82743,#82744,#82745));
#19782=EDGE_LOOP('',(#82746,#82747,#82748,#82749));
#19783=EDGE_LOOP('',(#82750,#82751,#82752,#82753));
#19784=EDGE_LOOP('',(#82754,#82755,#82756,#82757));
#19785=EDGE_LOOP('',(#82758,#82759,#82760,#82761));
#19786=EDGE_LOOP('',(#82762,#82763,#82764,#82765));
#19787=EDGE_LOOP('',(#82766,#82767,#82768,#82769));
#19788=EDGE_LOOP('',(#82770,#82771,#82772,#82773));
#19789=EDGE_LOOP('',(#82774,#82775,#82776,#82777));
#19790=EDGE_LOOP('',(#82778,#82779,#82780,#82781));
#19791=EDGE_LOOP('',(#82782,#82783,#82784,#82785));
#19792=EDGE_LOOP('',(#82786,#82787,#82788,#82789));
#19793=EDGE_LOOP('',(#82790,#82791,#82792,#82793));
#19794=EDGE_LOOP('',(#82794,#82795,#82796,#82797));
#19795=EDGE_LOOP('',(#82798,#82799,#82800,#82801));
#19796=EDGE_LOOP('',(#82802,#82803,#82804,#82805,#82806,#82807));
#19797=EDGE_LOOP('',(#82808,#82809,#82810,#82811,#82812,#82813));
#19798=EDGE_LOOP('',(#82814,#82815,#82816,#82817,#82818,#82819));
#19799=EDGE_LOOP('',(#82820,#82821,#82822,#82823,#82824,#82825));
#19800=EDGE_LOOP('',(#82826,#82827,#82828,#82829,#82830,#82831));
#19801=EDGE_LOOP('',(#82832,#82833,#82834,#82835,#82836,#82837));
#19802=EDGE_LOOP('',(#82838,#82839,#82840,#82841,#82842,#82843));
#19803=EDGE_LOOP('',(#82844,#82845,#82846,#82847,#82848,#82849));
#19804=EDGE_LOOP('',(#82850,#82851,#82852,#82853,#82854,#82855));
#19805=EDGE_LOOP('',(#82856,#82857,#82858,#82859,#82860,#82861));
#19806=EDGE_LOOP('',(#82862,#82863,#82864,#82865,#82866,#82867));
#19807=EDGE_LOOP('',(#82868,#82869,#82870,#82871,#82872,#82873));
#19808=EDGE_LOOP('',(#82874,#82875,#82876,#82877,#82878,#82879));
#19809=EDGE_LOOP('',(#82880,#82881,#82882,#82883,#82884,#82885));
#19810=EDGE_LOOP('',(#82886,#82887,#82888,#82889,#82890,#82891));
#19811=EDGE_LOOP('',(#82892,#82893,#82894,#82895,#82896,#82897));
#19812=EDGE_LOOP('',(#82898,#82899,#82900,#82901,#82902,#82903));
#19813=EDGE_LOOP('',(#82904,#82905,#82906,#82907,#82908,#82909));
#19814=EDGE_LOOP('',(#82910,#82911,#82912,#82913,#82914,#82915));
#19815=EDGE_LOOP('',(#82916,#82917,#82918,#82919,#82920,#82921));
#19816=EDGE_LOOP('',(#82922,#82923,#82924,#82925,#82926,#82927));
#19817=EDGE_LOOP('',(#82928,#82929,#82930,#82931,#82932,#82933));
#19818=EDGE_LOOP('',(#82934,#82935,#82936,#82937,#82938,#82939));
#19819=EDGE_LOOP('',(#82940,#82941,#82942,#82943,#82944,#82945));
#19820=EDGE_LOOP('',(#82946,#82947,#82948,#82949,#82950,#82951));
#19821=EDGE_LOOP('',(#82952,#82953,#82954,#82955,#82956,#82957));
#19822=EDGE_LOOP('',(#82958,#82959,#82960,#82961,#82962,#82963));
#19823=EDGE_LOOP('',(#82964,#82965,#82966,#82967,#82968,#82969));
#19824=EDGE_LOOP('',(#82970,#82971,#82972,#82973,#82974,#82975));
#19825=EDGE_LOOP('',(#82976,#82977,#82978,#82979));
#19826=EDGE_LOOP('',(#82980,#82981,#82982,#82983,#82984,#82985));
#19827=EDGE_LOOP('',(#82986,#82987,#82988,#82989,#82990,#82991,#82992,#82993,
#82994,#82995,#82996,#82997,#82998,#82999,#83000,#83001,#83002,#83003,#83004,
#83005,#83006,#83007,#83008,#83009,#83010,#83011,#83012,#83013,#83014,#83015,
#83016,#83017,#83018,#83019,#83020,#83021,#83022,#83023,#83024,#83025,#83026,
#83027,#83028,#83029,#83030,#83031,#83032,#83033,#83034,#83035,#83036,#83037,
#83038,#83039,#83040,#83041,#83042,#83043,#83044,#83045));
#19828=EDGE_LOOP('',(#83046));
#19829=EDGE_LOOP('',(#83047,#83048,#83049,#83050));
#19830=EDGE_LOOP('',(#83051,#83052,#83053,#83054));
#19831=EDGE_LOOP('',(#83055,#83056,#83057,#83058,#83059,#83060,#83061,#83062));
#19832=EDGE_LOOP('',(#83063,#83064,#83065,#83066));
#19833=EDGE_LOOP('',(#83067,#83068,#83069,#83070));
#19834=EDGE_LOOP('',(#83071,#83072,#83073,#83074,#83075,#83076,#83077,#83078));
#19835=EDGE_LOOP('',(#83079,#83080,#83081,#83082));
#19836=EDGE_LOOP('',(#83083,#83084,#83085,#83086));
#19837=EDGE_LOOP('',(#83087,#83088,#83089,#83090));
#19838=EDGE_LOOP('',(#83091,#83092,#83093,#83094));
#19839=EDGE_LOOP('',(#83095,#83096,#83097,#83098));
#19840=EDGE_LOOP('',(#83099,#83100,#83101,#83102));
#19841=EDGE_LOOP('',(#83103,#83104,#83105,#83106));
#19842=EDGE_LOOP('',(#83107,#83108,#83109,#83110));
#19843=EDGE_LOOP('',(#83111,#83112,#83113,#83114,#83115,#83116,#83117,#83118));
#19844=EDGE_LOOP('',(#83119,#83120,#83121,#83122));
#19845=EDGE_LOOP('',(#83123,#83124,#83125,#83126));
#19846=EDGE_LOOP('',(#83127,#83128,#83129,#83130));
#19847=EDGE_LOOP('',(#83131,#83132,#83133,#83134));
#19848=EDGE_LOOP('',(#83135,#83136,#83137,#83138));
#19849=EDGE_LOOP('',(#83139,#83140,#83141,#83142));
#19850=EDGE_LOOP('',(#83143,#83144,#83145,#83146));
#19851=EDGE_LOOP('',(#83147,#83148,#83149,#83150));
#19852=EDGE_LOOP('',(#83151,#83152,#83153,#83154,#83155,#83156,#83157,#83158));
#19853=EDGE_LOOP('',(#83159,#83160,#83161,#83162));
#19854=EDGE_LOOP('',(#83163,#83164,#83165,#83166));
#19855=EDGE_LOOP('',(#83167,#83168,#83169,#83170));
#19856=EDGE_LOOP('',(#83171,#83172,#83173,#83174));
#19857=EDGE_LOOP('',(#83175,#83176,#83177,#83178));
#19858=EDGE_LOOP('',(#83179,#83180,#83181,#83182));
#19859=EDGE_LOOP('',(#83183,#83184,#83185,#83186));
#19860=EDGE_LOOP('',(#83187,#83188,#83189,#83190));
#19861=EDGE_LOOP('',(#83191,#83192,#83193,#83194));
#19862=EDGE_LOOP('',(#83195,#83196,#83197,#83198));
#19863=EDGE_LOOP('',(#83199,#83200,#83201,#83202));
#19864=EDGE_LOOP('',(#83203,#83204,#83205,#83206));
#19865=EDGE_LOOP('',(#83207,#83208,#83209,#83210));
#19866=EDGE_LOOP('',(#83211,#83212,#83213,#83214));
#19867=EDGE_LOOP('',(#83215,#83216,#83217,#83218,#83219,#83220,#83221,#83222));
#19868=EDGE_LOOP('',(#83223,#83224,#83225,#83226));
#19869=EDGE_LOOP('',(#83227,#83228,#83229,#83230));
#19870=EDGE_LOOP('',(#83231,#83232,#83233,#83234,#83235,#83236,#83237,#83238));
#19871=EDGE_LOOP('',(#83239,#83240,#83241,#83242));
#19872=EDGE_LOOP('',(#83243,#83244,#83245,#83246));
#19873=EDGE_LOOP('',(#83247,#83248,#83249,#83250,#83251,#83252,#83253,#83254));
#19874=EDGE_LOOP('',(#83255,#83256,#83257,#83258));
#19875=EDGE_LOOP('',(#83259,#83260,#83261,#83262,#83263,#83264,#83265,#83266));
#19876=EDGE_LOOP('',(#83267,#83268,#83269,#83270));
#19877=EDGE_LOOP('',(#83271,#83272,#83273,#83274));
#19878=EDGE_LOOP('',(#83275,#83276,#83277,#83278,#83279,#83280,#83281,#83282));
#19879=EDGE_LOOP('',(#83283,#83284,#83285,#83286));
#19880=EDGE_LOOP('',(#83287,#83288,#83289,#83290));
#19881=EDGE_LOOP('',(#83291,#83292,#83293,#83294,#83295,#83296,#83297,#83298));
#19882=EDGE_LOOP('',(#83299,#83300,#83301,#83302));
#19883=EDGE_LOOP('',(#83303,#83304,#83305,#83306));
#19884=EDGE_LOOP('',(#83307,#83308,#83309,#83310,#83311,#83312,#83313,#83314));
#19885=EDGE_LOOP('',(#83315,#83316,#83317,#83318));
#19886=EDGE_LOOP('',(#83319,#83320,#83321,#83322));
#19887=EDGE_LOOP('',(#83323,#83324,#83325,#83326,#83327,#83328,#83329,#83330));
#19888=EDGE_LOOP('',(#83331,#83332,#83333,#83334));
#19889=EDGE_LOOP('',(#83335,#83336,#83337,#83338));
#19890=EDGE_LOOP('',(#83339,#83340,#83341,#83342,#83343,#83344,#83345,#83346));
#19891=EDGE_LOOP('',(#83347,#83348,#83349,#83350));
#19892=EDGE_LOOP('',(#83351,#83352,#83353,#83354,#83355,#83356,#83357,#83358));
#19893=EDGE_LOOP('',(#83359,#83360,#83361,#83362));
#19894=EDGE_LOOP('',(#83363,#83364,#83365,#83366));
#19895=EDGE_LOOP('',(#83367,#83368,#83369,#83370,#83371,#83372,#83373,#83374));
#19896=EDGE_LOOP('',(#83375,#83376,#83377,#83378));
#19897=EDGE_LOOP('',(#83379,#83380,#83381,#83382));
#19898=EDGE_LOOP('',(#83383,#83384,#83385,#83386,#83387,#83388,#83389,#83390));
#19899=EDGE_LOOP('',(#83391,#83392,#83393,#83394));
#19900=EDGE_LOOP('',(#83395,#83396,#83397,#83398));
#19901=EDGE_LOOP('',(#83399,#83400,#83401,#83402,#83403,#83404,#83405,#83406));
#19902=EDGE_LOOP('',(#83407,#83408,#83409,#83410));
#19903=EDGE_LOOP('',(#83411,#83412,#83413,#83414));
#19904=EDGE_LOOP('',(#83415,#83416,#83417,#83418,#83419,#83420,#83421,#83422));
#19905=EDGE_LOOP('',(#83423,#83424,#83425,#83426));
#19906=EDGE_LOOP('',(#83427,#83428,#83429,#83430));
#19907=EDGE_LOOP('',(#83431,#83432,#83433,#83434));
#24286=LINE('',#272472,#28633);
#24287=LINE('',#272484,#28634);
#24288=LINE('',#272494,#28635);
#24289=LINE('',#272507,#28636);
#24290=LINE('',#272515,#28637);
#24291=LINE('',#272532,#28638);
#24292=LINE('',#272552,#28639);
#24293=LINE('',#272575,#28640);
#24294=LINE('',#272595,#28641);
#24295=LINE('',#272618,#28642);
#24296=LINE('',#272638,#28643);
#24297=LINE('',#272661,#28644);
#24298=LINE('',#272681,#28645);
#24299=LINE('',#272698,#28646);
#24300=LINE('',#272718,#28647);
#24301=LINE('',#272737,#28648);
#24302=LINE('',#272757,#28649);
#24303=LINE('',#272789,#28650);
#24304=LINE('',#272804,#28651);
#24305=LINE('',#272821,#28652);
#24306=LINE('',#272841,#28653);
#24307=LINE('',#272871,#28654);
#24308=LINE('',#272886,#28655);
#24309=LINE('',#272903,#28656);
#24310=LINE('',#272923,#28657);
#24311=LINE('',#272946,#28658);
#24312=LINE('',#272966,#28659);
#24313=LINE('',#272989,#28660);
#24314=LINE('',#273009,#28661);
#24315=LINE('',#273057,#28662);
#24316=LINE('',#273058,#28663);
#24317=LINE('',#273100,#28664);
#24318=LINE('',#273103,#28665);
#24319=LINE('',#273187,#28666);
#24320=LINE('',#273189,#28667);
#24321=LINE('',#273190,#28668);
#24322=LINE('',#273193,#28669);
#24323=LINE('',#273195,#28670);
#24324=LINE('',#273196,#28671);
#24325=LINE('',#273973,#28672);
#24326=LINE('',#273976,#28673);
#24327=LINE('',#273979,#28674);
#24328=LINE('',#273981,#28675);
#24329=LINE('',#273985,#28676);
#24330=LINE('',#273987,#28677);
#24331=LINE('',#273991,#28678);
#24332=LINE('',#273993,#28679);
#24333=LINE('',#273997,#28680);
#24334=LINE('',#274000,#28681);
#24335=LINE('',#274003,#28682);
#24336=LINE('',#274007,#28683);
#24337=LINE('',#274009,#28684);
#24338=LINE('',#274013,#28685);
#24339=LINE('',#274016,#28686);
#24340=LINE('',#274019,#28687);
#24341=LINE('',#274021,#28688);
#24342=LINE('',#274025,#28689);
#24343=LINE('',#274029,#28690);
#24344=LINE('',#274032,#28691);
#24345=LINE('',#274035,#28692);
#24346=LINE('',#274037,#28693);
#24347=LINE('',#274041,#28694);
#24348=LINE('',#274044,#28695);
#24349=LINE('',#274047,#28696);
#24350=LINE('',#274049,#28697);
#24351=LINE('',#274053,#28698);
#24352=LINE('',#274056,#28699);
#24353=LINE('',#274059,#28700);
#24354=LINE('',#274061,#28701);
#24355=LINE('',#274065,#28702);
#24356=LINE('',#274067,#28703);
#24357=LINE('',#274071,#28704);
#24358=LINE('',#274074,#28705);
#24359=LINE('',#274077,#28706);
#24360=LINE('',#274079,#28707);
#24361=LINE('',#274083,#28708);
#24362=LINE('',#274086,#28709);
#24363=LINE('',#274089,#28710);
#24364=LINE('',#274091,#28711);
#24365=LINE('',#274095,#28712);
#24366=LINE('',#274098,#28713);
#24367=LINE('',#274101,#28714);
#24368=LINE('',#274103,#28715);
#24369=LINE('',#274107,#28716);
#24370=LINE('',#274109,#28717);
#24371=LINE('',#274113,#28718);
#24372=LINE('',#274116,#28719);
#24373=LINE('',#274119,#28720);
#24374=LINE('',#274122,#28721);
#24375=LINE('',#274125,#28722);
#24376=LINE('',#274127,#28723);
#24377=LINE('',#274131,#28724);
#24378=LINE('',#274133,#28725);
#24379=LINE('',#274893,#28726);
#24380=LINE('',#274895,#28727);
#24381=LINE('',#274951,#28728);
#24382=LINE('',#274953,#28729);
#24383=LINE('',#274956,#28730);
#24384=LINE('',#274958,#28731);
#24385=LINE('',#274967,#28732);
#24386=LINE('',#274969,#28733);
#24387=LINE('',#274978,#28734);
#24388=LINE('',#274980,#28735);
#24389=LINE('',#274995,#28736);
#24390=LINE('',#274997,#28737);
#24391=LINE('',#275000,#28738);
#24392=LINE('',#275002,#28739);
#24393=LINE('',#275005,#28740);
#24394=LINE('',#275007,#28741);
#24395=LINE('',#275010,#28742);
#24396=LINE('',#275013,#28743);
#24397=LINE('',#275015,#28744);
#24398=LINE('',#275018,#28745);
#24399=LINE('',#275020,#28746);
#24400=LINE('',#275023,#28747);
#24401=LINE('',#275025,#28748);
#24402=LINE('',#275028,#28749);
#24403=LINE('',#275030,#28750);
#24404=LINE('',#275033,#28751);
#24405=LINE('',#275035,#28752);
#24406=LINE('',#275038,#28753);
#24407=LINE('',#275041,#28754);
#24408=LINE('',#275043,#28755);
#24409=LINE('',#275046,#28756);
#24410=LINE('',#275048,#28757);
#24411=LINE('',#275051,#28758);
#24412=LINE('',#275053,#28759);
#24413=LINE('',#275056,#28760);
#24414=LINE('',#275058,#28761);
#24415=LINE('',#275061,#28762);
#24416=LINE('',#275062,#28763);
#28633=VECTOR('',#127849,25.2);
#28634=VECTOR('',#127854,1000.);
#28635=VECTOR('',#127855,1000.);
#28636=VECTOR('',#127858,1000.);
#28637=VECTOR('',#127859,1000.);
#28638=VECTOR('',#127864,1000.);
#28639=VECTOR('',#127867,1000.);
#28640=VECTOR('',#127872,1000.);
#28641=VECTOR('',#127875,1000.);
#28642=VECTOR('',#127880,1000.);
#28643=VECTOR('',#127883,1000.);
#28644=VECTOR('',#127888,1000.);
#28645=VECTOR('',#127891,1000.);
#28646=VECTOR('',#127894,1000.);
#28647=VECTOR('',#127897,1000.);
#28648=VECTOR('',#127902,1000.);
#28649=VECTOR('',#127905,1000.);
#28650=VECTOR('',#127912,1000.);
#28651=VECTOR('',#127915,1000.);
#28652=VECTOR('',#127920,1000.);
#28653=VECTOR('',#127923,1000.);
#28654=VECTOR('',#127928,1000.);
#28655=VECTOR('',#127931,1000.);
#28656=VECTOR('',#127936,1000.);
#28657=VECTOR('',#127939,1000.);
#28658=VECTOR('',#127944,1000.);
#28659=VECTOR('',#127947,1000.);
#28660=VECTOR('',#127952,1000.);
#28661=VECTOR('',#127955,1000.);
#28662=VECTOR('',#127966,1000.);
#28663=VECTOR('',#127967,1000.);
#28664=VECTOR('',#127976,1000.);
#28665=VECTOR('',#127979,1000.);
#28666=VECTOR('',#128076,1000.);
#28667=VECTOR('',#128077,1000.);
#28668=VECTOR('',#128078,1000.);
#28669=VECTOR('',#128081,1000.);
#28670=VECTOR('',#128082,1000.);
#28671=VECTOR('',#128083,1000.);
#28672=VECTOR('',#128198,1000.);
#28673=VECTOR('',#128201,1000.);
#28674=VECTOR('',#128204,1000.);
#28675=VECTOR('',#128205,1000.);
#28676=VECTOR('',#128210,1000.);
#28677=VECTOR('',#128211,1000.);
#28678=VECTOR('',#128216,1000.);
#28679=VECTOR('',#128217,1000.);
#28680=VECTOR('',#128222,1000.);
#28681=VECTOR('',#128225,1000.);
#28682=VECTOR('',#128228,1000.);
#28683=VECTOR('',#128233,1000.);
#28684=VECTOR('',#128234,1000.);
#28685=VECTOR('',#128239,1000.);
#28686=VECTOR('',#128242,1000.);
#28687=VECTOR('',#128245,1000.);
#28688=VECTOR('',#128246,1000.);
#28689=VECTOR('',#128251,1000.);
#28690=VECTOR('',#128256,1000.);
#28691=VECTOR('',#128259,1000.);
#28692=VECTOR('',#128262,1000.);
#28693=VECTOR('',#128263,1000.);
#28694=VECTOR('',#128268,1000.);
#28695=VECTOR('',#128271,1000.);
#28696=VECTOR('',#128274,1000.);
#28697=VECTOR('',#128275,1000.);
#28698=VECTOR('',#128280,1000.);
#28699=VECTOR('',#128283,1000.);
#28700=VECTOR('',#128286,1000.);
#28701=VECTOR('',#128287,1000.);
#28702=VECTOR('',#128292,1000.);
#28703=VECTOR('',#128293,1000.);
#28704=VECTOR('',#128298,1000.);
#28705=VECTOR('',#128301,1000.);
#28706=VECTOR('',#128304,1000.);
#28707=VECTOR('',#128305,1000.);
#28708=VECTOR('',#128310,1000.);
#28709=VECTOR('',#128313,1000.);
#28710=VECTOR('',#128316,1000.);
#28711=VECTOR('',#128317,1000.);
#28712=VECTOR('',#128322,1000.);
#28713=VECTOR('',#128325,1000.);
#28714=VECTOR('',#128328,1000.);
#28715=VECTOR('',#128329,1000.);
#28716=VECTOR('',#128334,1000.);
#28717=VECTOR('',#128335,1000.);
#28718=VECTOR('',#128340,1000.);
#28719=VECTOR('',#128343,1000.);
#28720=VECTOR('',#128346,1000.);
#28721=VECTOR('',#128349,1000.);
#28722=VECTOR('',#128352,1000.);
#28723=VECTOR('',#128353,1000.);
#28724=VECTOR('',#128358,1000.);
#28725=VECTOR('',#128359,1000.);
#28726=VECTOR('',#128480,1000.);
#28727=VECTOR('',#128481,1000.);
#28728=VECTOR('',#128528,1000.);
#28729=VECTOR('',#128531,1000.);
#28730=VECTOR('',#128536,1000.);
#28731=VECTOR('',#128539,1000.);
#28732=VECTOR('',#128556,1000.);
#28733=VECTOR('',#128559,1000.);
#28734=VECTOR('',#128576,1000.);
#28735=VECTOR('',#128579,1000.);
#28736=VECTOR('',#128608,1000.);
#28737=VECTOR('',#128611,1000.);
#28738=VECTOR('',#128616,1000.);
#28739=VECTOR('',#128619,1000.);
#28740=VECTOR('',#128624,1000.);
#28741=VECTOR('',#128627,1000.);
#28742=VECTOR('',#128632,1000.);
#28743=VECTOR('',#128637,1000.);
#28744=VECTOR('',#128640,1000.);
#28745=VECTOR('',#128645,1000.);
#28746=VECTOR('',#128648,1000.);
#28747=VECTOR('',#128653,1000.);
#28748=VECTOR('',#128656,1000.);
#28749=VECTOR('',#128661,1000.);
#28750=VECTOR('',#128664,1000.);
#28751=VECTOR('',#128669,1000.);
#28752=VECTOR('',#128672,1000.);
#28753=VECTOR('',#128677,1000.);
#28754=VECTOR('',#128682,1000.);
#28755=VECTOR('',#128685,1000.);
#28756=VECTOR('',#128690,1000.);
#28757=VECTOR('',#128693,1000.);
#28758=VECTOR('',#128698,1000.);
#28759=VECTOR('',#128701,1000.);
#28760=VECTOR('',#128706,1000.);
#28761=VECTOR('',#128709,1000.);
#28762=VECTOR('',#128714,1000.);
#28763=VECTOR('',#128715,1000.);
#34665=CIRCLE('',#103549,25.536);
#34666=CIRCLE('',#103550,0.336);
#34667=CIRCLE('',#103551,25.2);
#34668=CIRCLE('',#103553,25.2);
#34669=CIRCLE('',#103557,3.36814799999999);
#34670=CIRCLE('',#103558,3.36814799999999);
#34671=CIRCLE('',#103560,3.368148);
#34672=CIRCLE('',#103561,3.36814799999999);
#34673=CIRCLE('',#103563,3.36814799999999);
#34674=CIRCLE('',#103564,3.36814799999999);
#34675=CIRCLE('',#103566,3.36814799999999);
#34676=CIRCLE('',#103567,3.36814799999999);
#34677=CIRCLE('',#103569,3.36814799999999);
#34678=CIRCLE('',#103570,3.36814799999999);
#34679=CIRCLE('',#103572,3.36814799999999);
#34680=CIRCLE('',#103573,3.368148);
#34681=CIRCLE('',#103575,3.36814799999999);
#34682=CIRCLE('',#103576,3.36814799999999);
#34683=CIRCLE('',#103578,3.36814799999999);
#34684=CIRCLE('',#103579,3.36814799999999);
#34685=CIRCLE('',#103581,3.368148);
#34686=CIRCLE('',#103582,3.36814799999999);
#34687=CIRCLE('',#103584,3.36814799999999);
#34688=CIRCLE('',#103585,3.36814799999999);
#34689=CIRCLE('',#103587,3.36814799999999);
#34690=CIRCLE('',#103588,3.36814799999999);
#34691=CIRCLE('',#103590,3.368148);
#34692=CIRCLE('',#103591,3.36814799999999);
#34693=CIRCLE('',#103593,54.361863151615);
#34694=CIRCLE('',#103594,49.1019873874548);
#34695=CIRCLE('',#103596,54.361863151615);
#34696=CIRCLE('',#103598,49.1019873874548);
#34697=CIRCLE('',#103600,8.82);
#34698=CIRCLE('',#103601,8.82);
#34699=CIRCLE('',#103603,3.368148);
#34700=CIRCLE('',#103604,49.1019873874548);
#34701=CIRCLE('',#103605,3.368148);
#34702=CIRCLE('',#103606,49.1019873874548);
#34703=CIRCLE('',#103607,3.36814799999999);
#34704=CIRCLE('',#103608,49.1019873874548);
#34705=CIRCLE('',#103609,3.368148);
#34706=CIRCLE('',#103610,49.1019873874548);
#34707=CIRCLE('',#103611,3.368148);
#34708=CIRCLE('',#103612,49.1019873874548);
#34709=CIRCLE('',#103613,3.36814799999999);
#34710=CIRCLE('',#103614,49.1019873874548);
#34711=CIRCLE('',#103615,3.36814799999999);
#34712=CIRCLE('',#103616,49.1019873874548);
#34713=CIRCLE('',#103617,3.36814799999999);
#34714=CIRCLE('',#103618,49.1019873874548);
#34715=CIRCLE('',#103619,3.36814799999999);
#34716=CIRCLE('',#103620,49.1019873874548);
#34717=CIRCLE('',#103621,49.1019873874548);
#34718=CIRCLE('',#103622,49.1019873874548);
#34719=CIRCLE('',#103623,49.1019873874548);
#34720=CIRCLE('',#103624,49.1019873874548);
#34721=CIRCLE('',#103625,49.1019873874548);
#34722=CIRCLE('',#103626,49.1019873874548);
#34723=CIRCLE('',#103627,49.1019873874548);
#34724=CIRCLE('',#103628,49.1019873874548);
#34725=CIRCLE('',#103629,49.1019873874548);
#34726=CIRCLE('',#103630,49.1019873874548);
#34727=CIRCLE('',#103631,49.1019873874548);
#34728=CIRCLE('',#103632,49.1019873874548);
#34729=CIRCLE('',#103633,3.36814799999999);
#34730=CIRCLE('',#103634,49.1019873874548);
#34731=CIRCLE('',#103635,3.36814799999999);
#34732=CIRCLE('',#103636,49.1019873874548);
#34733=CIRCLE('',#103637,3.36814799999999);
#34734=CIRCLE('',#103638,49.1019873874548);
#34735=CIRCLE('',#103639,3.36814799999999);
#34736=CIRCLE('',#103640,49.1019873874548);
#34737=CIRCLE('',#103641,3.36814799999999);
#34738=CIRCLE('',#103642,49.1019873874548);
#34739=CIRCLE('',#103643,3.36814799999999);
#34740=CIRCLE('',#103644,49.1019873874548);
#34741=CIRCLE('',#103645,3.368148);
#34742=CIRCLE('',#103646,49.1019873874548);
#34743=CIRCLE('',#103647,3.36814799999999);
#34744=CIRCLE('',#103648,49.1019873874548);
#34745=CIRCLE('',#103649,3.368148);
#34746=CIRCLE('',#103652,54.361863151615);
#34747=CIRCLE('',#103654,54.361863151615);
#34748=CIRCLE('',#103656,54.361863151615);
#34749=CIRCLE('',#103658,54.361863151615);
#34750=CIRCLE('',#103660,54.361863151615);
#34751=CIRCLE('',#103662,54.361863151615);
#34752=CIRCLE('',#103664,54.361863151615);
#34753=CIRCLE('',#103666,54.361863151615);
#34754=CIRCLE('',#103668,54.361863151615);
#34755=CIRCLE('',#103670,54.361863151615);
#34756=CIRCLE('',#103672,54.361863151615);
#34757=CIRCLE('',#103674,54.361863151615);
#34758=CIRCLE('',#103676,54.361863151615);
#34759=CIRCLE('',#103678,54.361863151615);
#34760=CIRCLE('',#103680,54.361863151615);
#34761=CIRCLE('',#103682,54.361863151615);
#34762=CIRCLE('',#103684,54.361863151615);
#34763=CIRCLE('',#103686,54.361863151615);
#34764=CIRCLE('',#103688,54.361863151615);
#34765=CIRCLE('',#103690,54.361863151615);
#34766=CIRCLE('',#103692,54.361863151615);
#34767=CIRCLE('',#103694,54.361863151615);
#34768=CIRCLE('',#103696,54.361863151615);
#34769=CIRCLE('',#103698,54.361863151615);
#34770=CIRCLE('',#103700,54.361863151615);
#34771=CIRCLE('',#103702,54.361863151615);
#34772=CIRCLE('',#103704,54.361863151615);
#34773=CIRCLE('',#103706,54.361863151615);
#34774=CIRCLE('',#103708,54.361863151615);
#34775=CIRCLE('',#103710,54.361863151615);
#34776=CIRCLE('',#103712,54.361863151615);
#34777=CIRCLE('',#103714,54.361863151615);
#34778=CIRCLE('',#103716,54.361863151615);
#34779=CIRCLE('',#103718,54.361863151615);
#34780=CIRCLE('',#103720,54.361863151615);
#34781=CIRCLE('',#103722,54.361863151615);
#34782=CIRCLE('',#103724,54.361863151615);
#34783=CIRCLE('',#103726,54.361863151615);
#34784=CIRCLE('',#103728,54.361863151615);
#34785=CIRCLE('',#103730,54.361863151615);
#34786=CIRCLE('',#103732,54.361863151615);
#34787=CIRCLE('',#103734,54.361863151615);
#34788=CIRCLE('',#103736,54.361863151615);
#34789=CIRCLE('',#103738,54.361863151615);
#34790=CIRCLE('',#103740,54.361863151615);
#34791=CIRCLE('',#103742,54.361863151615);
#34792=CIRCLE('',#103744,54.361863151615);
#34793=CIRCLE('',#103746,54.361863151615);
#34794=CIRCLE('',#103748,54.361863151615);
#34795=CIRCLE('',#103750,54.361863151615);
#34796=CIRCLE('',#103752,54.361863151615);
#34797=CIRCLE('',#103754,54.361863151615);
#34798=CIRCLE('',#103756,54.361863151615);
#34799=CIRCLE('',#103758,54.361863151615);
#34800=CIRCLE('',#103760,54.361863151615);
#34801=CIRCLE('',#103762,54.361863151615);
#34802=CIRCLE('',#103764,49.1019873874548);
#34803=CIRCLE('',#103766,49.1019873874548);
#34804=CIRCLE('',#103768,49.1019873874548);
#34805=CIRCLE('',#103770,49.1019873874548);
#34806=CIRCLE('',#103772,49.1019873874548);
#34807=CIRCLE('',#103774,49.1019873874548);
#34808=CIRCLE('',#103776,49.1019873874548);
#34809=CIRCLE('',#103778,49.1019873874548);
#34810=CIRCLE('',#103780,49.1019873874548);
#34811=CIRCLE('',#103782,49.1019873874548);
#34812=CIRCLE('',#103784,49.1019873874548);
#34813=CIRCLE('',#103786,49.1019873874548);
#34814=CIRCLE('',#103788,49.1019873874548);
#34815=CIRCLE('',#103790,49.1019873874548);
#34816=CIRCLE('',#103792,49.1019873874548);
#34817=CIRCLE('',#103794,49.1019873874548);
#34818=CIRCLE('',#103796,49.1019873874548);
#34819=CIRCLE('',#103798,49.1019873874548);
#34820=CIRCLE('',#103800,49.1019873874548);
#34821=CIRCLE('',#103802,49.1019873874548);
#34822=CIRCLE('',#103804,49.1019873874548);
#34823=CIRCLE('',#103806,49.1019873874548);
#34824=CIRCLE('',#103808,49.1019873874548);
#34825=CIRCLE('',#103810,49.1019873874548);
#34826=CIRCLE('',#103812,49.1019873874548);
#34827=CIRCLE('',#103814,49.1019873874548);
#34828=CIRCLE('',#103816,49.1019873874548);
#34829=CIRCLE('',#103818,49.1019873874548);
#34830=CIRCLE('',#103820,54.361863151615);
#34831=CIRCLE('',#103822,54.361863151615);
#34832=CIRCLE('',#103824,49.1019873874548);
#34833=CIRCLE('',#103826,3.36814799999999);
#34834=CIRCLE('',#103827,3.36814799999999);
#34835=CIRCLE('',#103828,3.36814799999999);
#34836=CIRCLE('',#103829,3.36814799999999);
#34837=CIRCLE('',#103830,3.36814799999999);
#34838=CIRCLE('',#103831,3.36814799999999);
#34839=CIRCLE('',#103832,3.36814799999999);
#34840=CIRCLE('',#103833,3.36814799999999);
#34841=CIRCLE('',#103834,3.36814799999999);
#34842=CIRCLE('',#103835,3.36814799999999);
#34843=CIRCLE('',#103836,3.36814799999999);
#34844=CIRCLE('',#103837,3.36814799999999);
#34845=CIRCLE('',#103838,3.36814799999999);
#34846=CIRCLE('',#103839,3.36814799999999);
#34847=CIRCLE('',#103840,3.36814799999999);
#34848=CIRCLE('',#103841,3.36814799999999);
#34849=CIRCLE('',#103842,3.36814799999999);
#34850=CIRCLE('',#103843,3.36814799999999);
#42454=VERTEX_POINT('',#272465);
#42455=VERTEX_POINT('',#272467);
#42456=VERTEX_POINT('',#272471);
#42457=VERTEX_POINT('',#272475);
#42458=VERTEX_POINT('',#272476);
#42459=VERTEX_POINT('',#272483);
#42460=VERTEX_POINT('',#272485);
#42461=VERTEX_POINT('',#272496);
#42462=VERTEX_POINT('',#272497);
#42463=VERTEX_POINT('',#272506);
#42464=VERTEX_POINT('',#272508);
#42465=VERTEX_POINT('',#272517);
#42466=VERTEX_POINT('',#272518);
#42467=VERTEX_POINT('',#272520);
#42468=VERTEX_POINT('',#272531);
#42469=VERTEX_POINT('',#272533);
#42470=VERTEX_POINT('',#272538);
#42471=VERTEX_POINT('',#272540);
#42472=VERTEX_POINT('',#272551);
#42473=VERTEX_POINT('',#272560);
#42474=VERTEX_POINT('',#272561);
#42475=VERTEX_POINT('',#272563);
#42476=VERTEX_POINT('',#272574);
#42477=VERTEX_POINT('',#272576);
#42478=VERTEX_POINT('',#272581);
#42479=VERTEX_POINT('',#272583);
#42480=VERTEX_POINT('',#272594);
#42481=VERTEX_POINT('',#272603);
#42482=VERTEX_POINT('',#272604);
#42483=VERTEX_POINT('',#272606);
#42484=VERTEX_POINT('',#272617);
#42485=VERTEX_POINT('',#272619);
#42486=VERTEX_POINT('',#272624);
#42487=VERTEX_POINT('',#272626);
#42488=VERTEX_POINT('',#272637);
#42489=VERTEX_POINT('',#272646);
#42490=VERTEX_POINT('',#272647);
#42491=VERTEX_POINT('',#272649);
#42492=VERTEX_POINT('',#272660);
#42493=VERTEX_POINT('',#272662);
#42494=VERTEX_POINT('',#272667);
#42495=VERTEX_POINT('',#272669);
#42496=VERTEX_POINT('',#272680);
#42497=VERTEX_POINT('',#272689);
#42498=VERTEX_POINT('',#272690);
#42499=VERTEX_POINT('',#272697);
#42500=VERTEX_POINT('',#272699);
#42501=VERTEX_POINT('',#272704);
#42502=VERTEX_POINT('',#272706);
#42503=VERTEX_POINT('',#272717);
#42504=VERTEX_POINT('',#272719);
#42505=VERTEX_POINT('',#272728);
#42506=VERTEX_POINT('',#272729);
#42507=VERTEX_POINT('',#272736);
#42508=VERTEX_POINT('',#272738);
#42509=VERTEX_POINT('',#272743);
#42510=VERTEX_POINT('',#272745);
#42511=VERTEX_POINT('',#272756);
#42512=VERTEX_POINT('',#272758);
#42513=VERTEX_POINT('',#272767);
#42514=VERTEX_POINT('',#272768);
#42515=VERTEX_POINT('',#272775);
#42516=VERTEX_POINT('',#272777);
#42517=VERTEX_POINT('',#272788);
#42518=VERTEX_POINT('',#272790);
#42519=VERTEX_POINT('',#272795);
#42520=VERTEX_POINT('',#272797);
#42521=VERTEX_POINT('',#272806);
#42522=VERTEX_POINT('',#272807);
#42523=VERTEX_POINT('',#272809);
#42524=VERTEX_POINT('',#272820);
#42525=VERTEX_POINT('',#272822);
#42526=VERTEX_POINT('',#272827);
#42527=VERTEX_POINT('',#272829);
#42528=VERTEX_POINT('',#272840);
#42529=VERTEX_POINT('',#272849);
#42530=VERTEX_POINT('',#272850);
#42531=VERTEX_POINT('',#272857);
#42532=VERTEX_POINT('',#272859);
#42533=VERTEX_POINT('',#272870);
#42534=VERTEX_POINT('',#272872);
#42535=VERTEX_POINT('',#272877);
#42536=VERTEX_POINT('',#272879);
#42537=VERTEX_POINT('',#272888);
#42538=VERTEX_POINT('',#272889);
#42539=VERTEX_POINT('',#272891);
#42540=VERTEX_POINT('',#272902);
#42541=VERTEX_POINT('',#272904);
#42542=VERTEX_POINT('',#272909);
#42543=VERTEX_POINT('',#272911);
#42544=VERTEX_POINT('',#272922);
#42545=VERTEX_POINT('',#272931);
#42546=VERTEX_POINT('',#272932);
#42547=VERTEX_POINT('',#272934);
#42548=VERTEX_POINT('',#272945);
#42549=VERTEX_POINT('',#272947);
#42550=VERTEX_POINT('',#272952);
#42551=VERTEX_POINT('',#272954);
#42552=VERTEX_POINT('',#272965);
#42553=VERTEX_POINT('',#272974);
#42554=VERTEX_POINT('',#272975);
#42555=VERTEX_POINT('',#272977);
#42556=VERTEX_POINT('',#272988);
#42557=VERTEX_POINT('',#272990);
#42558=VERTEX_POINT('',#272995);
#42559=VERTEX_POINT('',#272997);
#42560=VERTEX_POINT('',#273008);
#42561=VERTEX_POINT('',#273017);
#42562=VERTEX_POINT('',#273018);
#42563=VERTEX_POINT('',#273020);
#42564=VERTEX_POINT('',#273027);
#42565=VERTEX_POINT('',#273038);
#42566=VERTEX_POINT('',#273040);
#42567=VERTEX_POINT('',#273054);
#42568=VERTEX_POINT('',#273055);
#42569=VERTEX_POINT('',#273060);
#42570=VERTEX_POINT('',#273061);
#42571=VERTEX_POINT('',#273063);
#42572=VERTEX_POINT('',#273078);
#42573=VERTEX_POINT('',#273096);
#42574=VERTEX_POINT('',#273097);
#42575=VERTEX_POINT('',#273099);
#42576=VERTEX_POINT('',#273101);
#42577=VERTEX_POINT('',#273105);
#42578=VERTEX_POINT('',#273107);
#42579=VERTEX_POINT('',#273109);
#42580=VERTEX_POINT('',#273111);
#42581=VERTEX_POINT('',#273113);
#42582=VERTEX_POINT('',#273115);
#42583=VERTEX_POINT('',#273117);
#42584=VERTEX_POINT('',#273119);
#42585=VERTEX_POINT('',#273121);
#42586=VERTEX_POINT('',#273123);
#42587=VERTEX_POINT('',#273125);
#42588=VERTEX_POINT('',#273127);
#42589=VERTEX_POINT('',#273129);
#42590=VERTEX_POINT('',#273131);
#42591=VERTEX_POINT('',#273133);
#42592=VERTEX_POINT('',#273135);
#42593=VERTEX_POINT('',#273137);
#42594=VERTEX_POINT('',#273151);
#42595=VERTEX_POINT('',#273153);
#42596=VERTEX_POINT('',#273155);
#42597=VERTEX_POINT('',#273157);
#42598=VERTEX_POINT('',#273159);
#42599=VERTEX_POINT('',#273161);
#42600=VERTEX_POINT('',#273163);
#42601=VERTEX_POINT('',#273165);
#42602=VERTEX_POINT('',#273167);
#42603=VERTEX_POINT('',#273169);
#42604=VERTEX_POINT('',#273171);
#42605=VERTEX_POINT('',#273173);
#42606=VERTEX_POINT('',#273175);
#42607=VERTEX_POINT('',#273177);
#42608=VERTEX_POINT('',#273179);
#42609=VERTEX_POINT('',#273181);
#42610=VERTEX_POINT('',#273183);
#42611=VERTEX_POINT('',#273186);
#42612=VERTEX_POINT('',#273188);
#42613=VERTEX_POINT('',#273192);
#42614=VERTEX_POINT('',#273194);
#42615=VERTEX_POINT('',#273198);
#42616=VERTEX_POINT('',#273199);
#42617=VERTEX_POINT('',#273208);
#42618=VERTEX_POINT('',#273210);
#42619=VERTEX_POINT('',#273234);
#42620=VERTEX_POINT('',#273245);
#42621=VERTEX_POINT('',#273252);
#42622=VERTEX_POINT('',#273261);
#42623=VERTEX_POINT('',#273270);
#42624=VERTEX_POINT('',#273281);
#42625=VERTEX_POINT('',#273288);
#42626=VERTEX_POINT('',#273297);
#42627=VERTEX_POINT('',#273306);
#42628=VERTEX_POINT('',#273317);
#42629=VERTEX_POINT('',#273324);
#42630=VERTEX_POINT('',#273333);
#42631=VERTEX_POINT('',#273342);
#42632=VERTEX_POINT('',#273343);
#42633=VERTEX_POINT('',#273352);
#42634=VERTEX_POINT('',#273354);
#42635=VERTEX_POINT('',#273388);
#42636=VERTEX_POINT('',#273395);
#42637=VERTEX_POINT('',#273406);
#42638=VERTEX_POINT('',#273417);
#42639=VERTEX_POINT('',#273424);
#42640=VERTEX_POINT('',#273433);
#42641=VERTEX_POINT('',#273442);
#42642=VERTEX_POINT('',#273443);
#42643=VERTEX_POINT('',#273452);
#42644=VERTEX_POINT('',#273454);
#42645=VERTEX_POINT('',#273478);
#42646=VERTEX_POINT('',#273489);
#42647=VERTEX_POINT('',#273496);
#42648=VERTEX_POINT('',#273505);
#42649=VERTEX_POINT('',#273514);
#42650=VERTEX_POINT('',#273531);
#42651=VERTEX_POINT('',#273540);
#42652=VERTEX_POINT('',#273541);
#42653=VERTEX_POINT('',#273550);
#42654=VERTEX_POINT('',#273552);
#42655=VERTEX_POINT('',#273576);
#42656=VERTEX_POINT('',#273587);
#42657=VERTEX_POINT('',#273594);
#42658=VERTEX_POINT('',#273603);
#42659=VERTEX_POINT('',#273612);
#42660=VERTEX_POINT('',#273613);
#42661=VERTEX_POINT('',#273622);
#42662=VERTEX_POINT('',#273624);
#42663=VERTEX_POINT('',#273648);
#42664=VERTEX_POINT('',#273659);
#42665=VERTEX_POINT('',#273666);
#42666=VERTEX_POINT('',#273675);
#42667=VERTEX_POINT('',#273684);
#42668=VERTEX_POINT('',#273693);
#42669=VERTEX_POINT('',#273702);
#42670=VERTEX_POINT('',#273711);
#42671=VERTEX_POINT('',#273720);
#42672=VERTEX_POINT('',#273729);
#42673=VERTEX_POINT('',#273738);
#42674=VERTEX_POINT('',#273747);
#42675=VERTEX_POINT('',#273756);
#42676=VERTEX_POINT('',#273765);
#42677=VERTEX_POINT('',#273774);
#42678=VERTEX_POINT('',#273783);
#42679=VERTEX_POINT('',#273792);
#42680=VERTEX_POINT('',#273799);
#42681=VERTEX_POINT('',#273808);
#42682=VERTEX_POINT('',#273817);
#42683=VERTEX_POINT('',#273826);
#42684=VERTEX_POINT('',#273835);
#42685=VERTEX_POINT('',#273844);
#42686=VERTEX_POINT('',#273853);
#42687=VERTEX_POINT('',#273862);
#42688=VERTEX_POINT('',#273871);
#42689=VERTEX_POINT('',#273880);
#42690=VERTEX_POINT('',#273882);
#42691=VERTEX_POINT('',#273900);
#42692=VERTEX_POINT('',#273901);
#42693=VERTEX_POINT('',#273910);
#42694=VERTEX_POINT('',#273912);
#42695=VERTEX_POINT('',#273936);
#42696=VERTEX_POINT('',#273945);
#42697=VERTEX_POINT('',#273954);
#42698=VERTEX_POINT('',#273963);
#42699=VERTEX_POINT('',#273972);
#42700=VERTEX_POINT('',#273974);
#42701=VERTEX_POINT('',#273978);
#42702=VERTEX_POINT('',#273980);
#42703=VERTEX_POINT('',#273984);
#42704=VERTEX_POINT('',#273986);
#42705=VERTEX_POINT('',#273990);
#42706=VERTEX_POINT('',#273992);
#42707=VERTEX_POINT('',#273996);
#42708=VERTEX_POINT('',#273998);
#42709=VERTEX_POINT('',#274002);
#42710=VERTEX_POINT('',#274006);
#42711=VERTEX_POINT('',#274008);
#42712=VERTEX_POINT('',#274012);
#42713=VERTEX_POINT('',#274014);
#42714=VERTEX_POINT('',#274018);
#42715=VERTEX_POINT('',#274020);
#42716=VERTEX_POINT('',#274024);
#42717=VERTEX_POINT('',#274028);
#42718=VERTEX_POINT('',#274030);
#42719=VERTEX_POINT('',#274034);
#42720=VERTEX_POINT('',#274036);
#42721=VERTEX_POINT('',#274040);
#42722=VERTEX_POINT('',#274042);
#42723=VERTEX_POINT('',#274046);
#42724=VERTEX_POINT('',#274048);
#42725=VERTEX_POINT('',#274052);
#42726=VERTEX_POINT('',#274054);
#42727=VERTEX_POINT('',#274058);
#42728=VERTEX_POINT('',#274060);
#42729=VERTEX_POINT('',#274064);
#42730=VERTEX_POINT('',#274066);
#42731=VERTEX_POINT('',#274070);
#42732=VERTEX_POINT('',#274072);
#42733=VERTEX_POINT('',#274076);
#42734=VERTEX_POINT('',#274078);
#42735=VERTEX_POINT('',#274082);
#42736=VERTEX_POINT('',#274084);
#42737=VERTEX_POINT('',#274088);
#42738=VERTEX_POINT('',#274090);
#42739=VERTEX_POINT('',#274094);
#42740=VERTEX_POINT('',#274096);
#42741=VERTEX_POINT('',#274100);
#42742=VERTEX_POINT('',#274102);
#42743=VERTEX_POINT('',#274106);
#42744=VERTEX_POINT('',#274108);
#42745=VERTEX_POINT('',#274112);
#42746=VERTEX_POINT('',#274114);
#42747=VERTEX_POINT('',#274118);
#42748=VERTEX_POINT('',#274120);
#42749=VERTEX_POINT('',#274124);
#42750=VERTEX_POINT('',#274126);
#42751=VERTEX_POINT('',#274130);
#42752=VERTEX_POINT('',#274132);
#42753=VERTEX_POINT('',#274136);
#42754=VERTEX_POINT('',#274143);
#42755=VERTEX_POINT('',#274154);
#42756=VERTEX_POINT('',#274156);
#42757=VERTEX_POINT('',#274170);
#42758=VERTEX_POINT('',#274171);
#42759=VERTEX_POINT('',#274184);
#42760=VERTEX_POINT('',#274191);
#42761=VERTEX_POINT('',#274204);
#42762=VERTEX_POINT('',#274205);
#42763=VERTEX_POINT('',#274218);
#42764=VERTEX_POINT('',#274225);
#42765=VERTEX_POINT('',#274238);
#42766=VERTEX_POINT('',#274239);
#42767=VERTEX_POINT('',#274252);
#42768=VERTEX_POINT('',#274259);
#42769=VERTEX_POINT('',#274272);
#42770=VERTEX_POINT('',#274279);
#42771=VERTEX_POINT('',#274290);
#42772=VERTEX_POINT('',#274292);
#42773=VERTEX_POINT('',#274306);
#42774=VERTEX_POINT('',#274311);
#42775=VERTEX_POINT('',#274318);
#42776=VERTEX_POINT('',#274331);
#42777=VERTEX_POINT('',#274332);
#42778=VERTEX_POINT('',#274345);
#42779=VERTEX_POINT('',#274352);
#42780=VERTEX_POINT('',#274365);
#42781=VERTEX_POINT('',#274372);
#42782=VERTEX_POINT('',#274383);
#42783=VERTEX_POINT('',#274385);
#42784=VERTEX_POINT('',#274399);
#42785=VERTEX_POINT('',#274400);
#42786=VERTEX_POINT('',#274413);
#42787=VERTEX_POINT('',#274420);
#42788=VERTEX_POINT('',#274433);
#42789=VERTEX_POINT('',#274434);
#42790=VERTEX_POINT('',#274447);
#42791=VERTEX_POINT('',#274460);
#42792=VERTEX_POINT('',#274467);
#42793=VERTEX_POINT('',#274478);
#42794=VERTEX_POINT('',#274480);
#42795=VERTEX_POINT('',#274494);
#42796=VERTEX_POINT('',#274495);
#42797=VERTEX_POINT('',#274508);
#42798=VERTEX_POINT('',#274515);
#42799=VERTEX_POINT('',#274528);
#42800=VERTEX_POINT('',#274535);
#42801=VERTEX_POINT('',#274546);
#42802=VERTEX_POINT('',#274548);
#42803=VERTEX_POINT('',#274562);
#42804=VERTEX_POINT('',#274563);
#42805=VERTEX_POINT('',#274576);
#42806=VERTEX_POINT('',#274583);
#42807=VERTEX_POINT('',#274700);
#42808=VERTEX_POINT('',#274707);
#42809=VERTEX_POINT('',#274774);
#42810=VERTEX_POINT('',#274776);
#42811=VERTEX_POINT('',#274790);
#42812=VERTEX_POINT('',#274797);
#42813=VERTEX_POINT('',#274808);
#42814=VERTEX_POINT('',#274810);
#42815=VERTEX_POINT('',#274856);
#42816=VERTEX_POINT('',#274867);
#42817=VERTEX_POINT('',#274874);
#42818=VERTEX_POINT('',#274883);
#42819=VERTEX_POINT('',#274892);
#42820=VERTEX_POINT('',#274894);
#42821=VERTEX_POINT('',#274898);
#42822=VERTEX_POINT('',#274899);
#42823=VERTEX_POINT('',#274912);
#42824=VERTEX_POINT('',#274919);
#55940=EDGE_CURVE('',#42454,#42454,#34665,.T.);
#55941=EDGE_CURVE('',#42454,#42455,#34666,.T.);
#55942=EDGE_CURVE('',#42455,#42455,#34667,.T.);
#55943=EDGE_CURVE('',#42455,#42456,#24286,.T.);
#55944=EDGE_CURVE('',#42456,#42456,#34668,.T.);
#55945=EDGE_CURVE('',#42457,#42458,#6426,.T.);
#55946=EDGE_CURVE('',#42458,#42459,#24287,.T.);
#55947=EDGE_CURVE('',#42459,#42460,#6427,.T.);
#55948=EDGE_CURVE('',#42457,#42460,#24288,.T.);
#55949=EDGE_CURVE('',#42461,#42462,#6428,.T.);
#55950=EDGE_CURVE('',#42462,#42463,#24289,.T.);
#55951=EDGE_CURVE('',#42463,#42464,#6429,.T.);
#55952=EDGE_CURVE('',#42464,#42461,#24290,.T.);
#55953=EDGE_CURVE('',#42465,#42466,#34669,.T.);
#55954=EDGE_CURVE('',#42466,#42467,#6430,.T.);
#55955=EDGE_CURVE('',#42467,#42468,#24291,.T.);
#55956=EDGE_CURVE('',#42468,#42469,#6431,.T.);
#55957=EDGE_CURVE('',#42469,#42470,#34670,.T.);
#55958=EDGE_CURVE('',#42470,#42471,#6432,.T.);
#55959=EDGE_CURVE('',#42472,#42471,#24292,.T.);
#55960=EDGE_CURVE('',#42472,#42465,#6433,.T.);
#55961=EDGE_CURVE('',#42473,#42474,#34671,.T.);
#55962=EDGE_CURVE('',#42474,#42475,#6434,.T.);
#55963=EDGE_CURVE('',#42475,#42476,#24293,.T.);
#55964=EDGE_CURVE('',#42476,#42477,#6435,.T.);
#55965=EDGE_CURVE('',#42477,#42478,#34672,.T.);
#55966=EDGE_CURVE('',#42478,#42479,#6436,.T.);
#55967=EDGE_CURVE('',#42480,#42479,#24294,.T.);
#55968=EDGE_CURVE('',#42480,#42473,#6437,.T.);
#55969=EDGE_CURVE('',#42481,#42482,#34673,.T.);
#55970=EDGE_CURVE('',#42482,#42483,#6438,.T.);
#55971=EDGE_CURVE('',#42483,#42484,#24295,.T.);
#55972=EDGE_CURVE('',#42484,#42485,#6439,.T.);
#55973=EDGE_CURVE('',#42485,#42486,#34674,.T.);
#55974=EDGE_CURVE('',#42486,#42487,#6440,.T.);
#55975=EDGE_CURVE('',#42488,#42487,#24296,.T.);
#55976=EDGE_CURVE('',#42488,#42481,#6441,.T.);
#55977=EDGE_CURVE('',#42489,#42490,#34675,.T.);
#55978=EDGE_CURVE('',#42490,#42491,#6442,.T.);
#55979=EDGE_CURVE('',#42491,#42492,#24297,.T.);
#55980=EDGE_CURVE('',#42492,#42493,#6443,.T.);
#55981=EDGE_CURVE('',#42493,#42494,#34676,.T.);
#55982=EDGE_CURVE('',#42494,#42495,#6444,.T.);
#55983=EDGE_CURVE('',#42496,#42495,#24298,.T.);
#55984=EDGE_CURVE('',#42496,#42489,#6445,.T.);
#55985=EDGE_CURVE('',#42497,#42498,#6446,.T.);
#55986=EDGE_CURVE('',#42498,#42499,#24299,.T.);
#55987=EDGE_CURVE('',#42499,#42500,#6447,.T.);
#55988=EDGE_CURVE('',#42500,#42501,#34677,.T.);
#55989=EDGE_CURVE('',#42501,#42502,#6448,.T.);
#55990=EDGE_CURVE('',#42503,#42502,#24300,.T.);
#55991=EDGE_CURVE('',#42503,#42504,#6449,.T.);
#55992=EDGE_CURVE('',#42504,#42497,#34678,.T.);
#55993=EDGE_CURVE('',#42505,#42506,#6450,.T.);
#55994=EDGE_CURVE('',#42506,#42507,#24301,.T.);
#55995=EDGE_CURVE('',#42507,#42508,#6451,.T.);
#55996=EDGE_CURVE('',#42508,#42509,#34679,.T.);
#55997=EDGE_CURVE('',#42509,#42510,#6452,.T.);
#55998=EDGE_CURVE('',#42511,#42510,#24302,.T.);
#55999=EDGE_CURVE('',#42511,#42512,#6453,.T.);
#56000=EDGE_CURVE('',#42512,#42505,#34680,.T.);
#56001=EDGE_CURVE('',#42513,#42514,#6454,.T.);
#56002=EDGE_CURVE('',#42514,#42515,#34681,.T.);
#56003=EDGE_CURVE('',#42515,#42516,#6455,.T.);
#56004=EDGE_CURVE('',#42516,#42517,#24303,.T.);
#56005=EDGE_CURVE('',#42517,#42518,#6456,.T.);
#56006=EDGE_CURVE('',#42518,#42519,#34682,.T.);
#56007=EDGE_CURVE('',#42519,#42520,#6457,.T.);
#56008=EDGE_CURVE('',#42513,#42520,#24304,.T.);
#56009=EDGE_CURVE('',#42521,#42522,#34683,.T.);
#56010=EDGE_CURVE('',#42522,#42523,#6458,.T.);
#56011=EDGE_CURVE('',#42523,#42524,#24305,.T.);
#56012=EDGE_CURVE('',#42524,#42525,#6459,.T.);
#56013=EDGE_CURVE('',#42525,#42526,#34684,.T.);
#56014=EDGE_CURVE('',#42526,#42527,#6460,.T.);
#56015=EDGE_CURVE('',#42528,#42527,#24306,.T.);
#56016=EDGE_CURVE('',#42528,#42521,#6461,.T.);
#56017=EDGE_CURVE('',#42529,#42530,#6462,.T.);
#56018=EDGE_CURVE('',#42530,#42531,#34685,.T.);
#56019=EDGE_CURVE('',#42531,#42532,#6463,.T.);
#56020=EDGE_CURVE('',#42532,#42533,#24307,.T.);
#56021=EDGE_CURVE('',#42533,#42534,#6464,.T.);
#56022=EDGE_CURVE('',#42534,#42535,#34686,.T.);
#56023=EDGE_CURVE('',#42535,#42536,#6465,.T.);
#56024=EDGE_CURVE('',#42529,#42536,#24308,.T.);
#56025=EDGE_CURVE('',#42537,#42538,#34687,.T.);
#56026=EDGE_CURVE('',#42538,#42539,#6466,.T.);
#56027=EDGE_CURVE('',#42539,#42540,#24309,.T.);
#56028=EDGE_CURVE('',#42540,#42541,#6467,.T.);
#56029=EDGE_CURVE('',#42541,#42542,#34688,.T.);
#56030=EDGE_CURVE('',#42542,#42543,#6468,.T.);
#56031=EDGE_CURVE('',#42544,#42543,#24310,.T.);
#56032=EDGE_CURVE('',#42544,#42537,#6469,.T.);
#56033=EDGE_CURVE('',#42545,#42546,#34689,.T.);
#56034=EDGE_CURVE('',#42546,#42547,#6470,.T.);
#56035=EDGE_CURVE('',#42547,#42548,#24311,.T.);
#56036=EDGE_CURVE('',#42548,#42549,#6471,.T.);
#56037=EDGE_CURVE('',#42549,#42550,#34690,.T.);
#56038=EDGE_CURVE('',#42550,#42551,#6472,.T.);
#56039=EDGE_CURVE('',#42552,#42551,#24312,.T.);
#56040=EDGE_CURVE('',#42552,#42545,#6473,.T.);
#56041=EDGE_CURVE('',#42553,#42554,#34691,.T.);
#56042=EDGE_CURVE('',#42554,#42555,#6474,.T.);
#56043=EDGE_CURVE('',#42555,#42556,#24313,.T.);
#56044=EDGE_CURVE('',#42556,#42557,#6475,.T.);
#56045=EDGE_CURVE('',#42557,#42558,#34692,.T.);
#56046=EDGE_CURVE('',#42558,#42559,#6476,.T.);
#56047=EDGE_CURVE('',#42560,#42559,#24314,.T.);
#56048=EDGE_CURVE('',#42560,#42553,#6477,.T.);
#56049=EDGE_CURVE('',#42561,#42562,#34693,.T.);
#56050=EDGE_CURVE('',#42563,#42562,#6478,.T.);
#56051=EDGE_CURVE('',#42564,#42563,#6479,.T.);
#56052=EDGE_CURVE('',#42565,#42564,#34694,.T.);
#56053=EDGE_CURVE('',#42566,#42565,#6480,.T.);
#56054=EDGE_CURVE('',#42561,#42566,#6481,.T.);
#56055=EDGE_CURVE('',#42567,#42568,#34695,.T.);
#56056=EDGE_CURVE('',#42562,#42568,#24315,.T.);
#56057=EDGE_CURVE('',#42567,#42561,#24316,.T.);
#56058=EDGE_CURVE('',#42569,#42570,#34696,.T.);
#56059=EDGE_CURVE('',#42571,#42570,#6482,.T.);
#56060=EDGE_CURVE('',#42568,#42571,#6483,.T.);
#56061=EDGE_CURVE('',#42572,#42567,#6484,.T.);
#56062=EDGE_CURVE('',#42569,#42572,#6485,.T.);
#56063=EDGE_CURVE('',#42573,#42574,#34697,.T.);
#56064=EDGE_CURVE('',#42574,#42575,#24317,.T.);
#56065=EDGE_CURVE('',#42576,#42575,#34698,.T.);
#56066=EDGE_CURVE('',#42576,#42573,#24318,.T.);
#56067=EDGE_CURVE('',#42577,#42569,#34699,.T.);
#56068=EDGE_CURVE('',#42578,#42577,#34700,.T.);
#56069=EDGE_CURVE('',#42579,#42578,#34701,.T.);
#56070=EDGE_CURVE('',#42580,#42579,#34702,.T.);
#56071=EDGE_CURVE('',#42581,#42580,#34703,.T.);
#56072=EDGE_CURVE('',#42582,#42581,#34704,.T.);
#56073=EDGE_CURVE('',#42583,#42582,#34705,.T.);
#56074=EDGE_CURVE('',#42584,#42583,#34706,.T.);
#56075=EDGE_CURVE('',#42585,#42584,#34707,.T.);
#56076=EDGE_CURVE('',#42586,#42585,#34708,.T.);
#56077=EDGE_CURVE('',#42587,#42586,#34709,.T.);
#56078=EDGE_CURVE('',#42588,#42587,#34710,.T.);
#56079=EDGE_CURVE('',#42589,#42588,#34711,.T.);
#56080=EDGE_CURVE('',#42590,#42589,#34712,.T.);
#56081=EDGE_CURVE('',#42591,#42590,#34713,.T.);
#56082=EDGE_CURVE('',#42592,#42591,#34714,.T.);
#56083=EDGE_CURVE('',#42593,#42592,#34715,.T.);
#56084=EDGE_CURVE('',#42497,#42593,#34716,.T.);
#56085=EDGE_CURVE('',#42505,#42504,#34717,.T.);
#56086=EDGE_CURVE('',#42482,#42512,#34718,.T.);
#56087=EDGE_CURVE('',#42490,#42481,#34719,.T.);
#56088=EDGE_CURVE('',#42474,#42489,#34720,.T.);
#56089=EDGE_CURVE('',#42466,#42473,#34721,.T.);
#56090=EDGE_CURVE('',#42554,#42465,#34722,.T.);
#56091=EDGE_CURVE('',#42546,#42553,#34723,.T.);
#56092=EDGE_CURVE('',#42538,#42545,#34724,.T.);
#56093=EDGE_CURVE('',#42522,#42537,#34725,.T.);
#56094=EDGE_CURVE('',#42515,#42521,#34726,.T.);
#56095=EDGE_CURVE('',#42531,#42514,#34727,.T.);
#56096=EDGE_CURVE('',#42594,#42530,#34728,.T.);
#56097=EDGE_CURVE('',#42595,#42594,#34729,.T.);
#56098=EDGE_CURVE('',#42596,#42595,#34730,.T.);
#56099=EDGE_CURVE('',#42597,#42596,#34731,.T.);
#56100=EDGE_CURVE('',#42598,#42597,#34732,.T.);
#56101=EDGE_CURVE('',#42599,#42598,#34733,.T.);
#56102=EDGE_CURVE('',#42600,#42599,#34734,.T.);
#56103=EDGE_CURVE('',#42601,#42600,#34735,.T.);
#56104=EDGE_CURVE('',#42602,#42601,#34736,.T.);
#56105=EDGE_CURVE('',#42603,#42602,#34737,.T.);
#56106=EDGE_CURVE('',#42604,#42603,#34738,.T.);
#56107=EDGE_CURVE('',#42605,#42604,#34739,.T.);
#56108=EDGE_CURVE('',#42606,#42605,#34740,.T.);
#56109=EDGE_CURVE('',#42607,#42606,#34741,.T.);
#56110=EDGE_CURVE('',#42608,#42607,#34742,.T.);
#56111=EDGE_CURVE('',#42609,#42608,#34743,.T.);
#56112=EDGE_CURVE('',#42610,#42609,#34744,.T.);
#56113=EDGE_CURVE('',#42570,#42610,#34745,.T.);
#56114=EDGE_CURVE('',#42574,#42611,#24319,.T.);
#56115=EDGE_CURVE('',#42612,#42573,#24320,.T.);
#56116=EDGE_CURVE('',#42611,#42612,#24321,.T.);
#56117=EDGE_CURVE('',#42575,#42613,#24322,.T.);
#56118=EDGE_CURVE('',#42613,#42614,#24323,.T.);
#56119=EDGE_CURVE('',#42614,#42576,#24324,.T.);
#56120=EDGE_CURVE('',#42615,#42616,#6486,.T.);
#56121=EDGE_CURVE('',#42617,#42615,#34746,.T.);
#56122=EDGE_CURVE('',#42618,#42617,#6487,.T.);
#56123=EDGE_CURVE('',#42578,#42618,#6488,.T.);
#56124=EDGE_CURVE('',#42616,#42577,#6489,.T.);
#56125=EDGE_CURVE('',#42610,#42619,#6490,.T.);
#56126=EDGE_CURVE('',#42620,#42609,#6491,.T.);
#56127=EDGE_CURVE('',#42621,#42620,#6492,.T.);
#56128=EDGE_CURVE('',#42622,#42621,#34747,.T.);
#56129=EDGE_CURVE('',#42619,#42622,#6493,.T.);
#56130=EDGE_CURVE('',#42608,#42623,#6494,.T.);
#56131=EDGE_CURVE('',#42624,#42607,#6495,.T.);
#56132=EDGE_CURVE('',#42625,#42624,#6496,.T.);
#56133=EDGE_CURVE('',#42626,#42625,#34748,.T.);
#56134=EDGE_CURVE('',#42623,#42626,#6497,.T.);
#56135=EDGE_CURVE('',#42606,#42627,#6498,.T.);
#56136=EDGE_CURVE('',#42628,#42605,#6499,.T.);
#56137=EDGE_CURVE('',#42629,#42628,#6500,.T.);
#56138=EDGE_CURVE('',#42630,#42629,#34749,.T.);
#56139=EDGE_CURVE('',#42627,#42630,#6501,.T.);
#56140=EDGE_CURVE('',#42631,#42632,#6502,.T.);
#56141=EDGE_CURVE('',#42633,#42631,#34750,.T.);
#56142=EDGE_CURVE('',#42634,#42633,#6503,.T.);
#56143=EDGE_CURVE('',#42602,#42634,#6504,.T.);
#56144=EDGE_CURVE('',#42632,#42601,#6505,.T.);
#56145=EDGE_CURVE('',#42600,#42457,#6506,.T.);
#56146=EDGE_CURVE('',#42635,#42599,#6507,.T.);
#56147=EDGE_CURVE('',#42636,#42635,#6508,.T.);
#56148=EDGE_CURVE('',#42458,#42636,#34751,.T.);
#56149=EDGE_CURVE('',#42604,#42637,#6509,.T.);
#56150=EDGE_CURVE('',#42638,#42603,#6510,.T.);
#56151=EDGE_CURVE('',#42639,#42638,#6511,.T.);
#56152=EDGE_CURVE('',#42640,#42639,#34752,.T.);
#56153=EDGE_CURVE('',#42637,#42640,#6512,.T.);
#56154=EDGE_CURVE('',#42641,#42642,#6513,.T.);
#56155=EDGE_CURVE('',#42643,#42641,#34753,.T.);
#56156=EDGE_CURVE('',#42644,#42643,#6514,.T.);
#56157=EDGE_CURVE('',#42592,#42644,#6515,.T.);
#56158=EDGE_CURVE('',#42642,#42591,#6516,.T.);
#56159=EDGE_CURVE('',#42590,#42645,#6517,.T.);
#56160=EDGE_CURVE('',#42646,#42589,#6518,.T.);
#56161=EDGE_CURVE('',#42647,#42646,#6519,.T.);
#56162=EDGE_CURVE('',#42648,#42647,#34754,.T.);
#56163=EDGE_CURVE('',#42645,#42648,#6520,.T.);
#56164=EDGE_CURVE('',#42588,#42649,#6521,.T.);
#56165=EDGE_CURVE('',#42462,#42587,#6522,.T.);
#56166=EDGE_CURVE('',#42650,#42461,#34755,.T.);
#56167=EDGE_CURVE('',#42649,#42650,#6523,.T.);
#56168=EDGE_CURVE('',#42651,#42652,#6524,.T.);
#56169=EDGE_CURVE('',#42653,#42651,#34756,.T.);
#56170=EDGE_CURVE('',#42654,#42653,#6525,.T.);
#56171=EDGE_CURVE('',#42586,#42654,#6526,.T.);
#56172=EDGE_CURVE('',#42652,#42585,#6527,.T.);
#56173=EDGE_CURVE('',#42584,#42655,#6528,.T.);
#56174=EDGE_CURVE('',#42656,#42583,#6529,.T.);
#56175=EDGE_CURVE('',#42657,#42656,#6530,.T.);
#56176=EDGE_CURVE('',#42658,#42657,#34757,.T.);
#56177=EDGE_CURVE('',#42655,#42658,#6531,.T.);
#56178=EDGE_CURVE('',#42659,#42660,#6532,.T.);
#56179=EDGE_CURVE('',#42661,#42659,#34758,.T.);
#56180=EDGE_CURVE('',#42662,#42661,#6533,.T.);
#56181=EDGE_CURVE('',#42582,#42662,#6534,.T.);
#56182=EDGE_CURVE('',#42660,#42581,#6535,.T.);
#56183=EDGE_CURVE('',#42580,#42663,#6536,.T.);
#56184=EDGE_CURVE('',#42664,#42579,#6537,.T.);
#56185=EDGE_CURVE('',#42665,#42664,#6538,.T.);
#56186=EDGE_CURVE('',#42666,#42665,#34759,.T.);
#56187=EDGE_CURVE('',#42663,#42666,#6539,.T.);
#56188=EDGE_CURVE('',#42667,#42472,#6540,.T.);
#56189=EDGE_CURVE('',#42668,#42667,#34760,.T.);
#56190=EDGE_CURVE('',#42555,#42668,#6541,.T.);
#56191=EDGE_CURVE('',#42669,#42480,#6542,.T.);
#56192=EDGE_CURVE('',#42670,#42669,#34761,.T.);
#56193=EDGE_CURVE('',#42467,#42670,#6543,.T.);
#56194=EDGE_CURVE('',#42671,#42496,#6544,.T.);
#56195=EDGE_CURVE('',#42672,#42671,#34762,.T.);
#56196=EDGE_CURVE('',#42475,#42672,#6545,.T.);
#56197=EDGE_CURVE('',#42673,#42488,#6546,.T.);
#56198=EDGE_CURVE('',#42674,#42673,#34763,.T.);
#56199=EDGE_CURVE('',#42491,#42674,#6547,.T.);
#56200=EDGE_CURVE('',#42675,#42511,#6548,.T.);
#56201=EDGE_CURVE('',#42676,#42675,#34764,.T.);
#56202=EDGE_CURVE('',#42483,#42676,#6549,.T.);
#56203=EDGE_CURVE('',#42677,#42503,#6550,.T.);
#56204=EDGE_CURVE('',#42678,#42677,#34765,.T.);
#56205=EDGE_CURVE('',#42506,#42678,#6551,.T.);
#56206=EDGE_CURVE('',#42679,#42593,#6552,.T.);
#56207=EDGE_CURVE('',#42680,#42679,#6553,.T.);
#56208=EDGE_CURVE('',#42681,#42680,#34766,.T.);
#56209=EDGE_CURVE('',#42498,#42681,#6554,.T.);
#56210=EDGE_CURVE('',#42682,#42513,#6555,.T.);
#56211=EDGE_CURVE('',#42683,#42682,#34767,.T.);
#56212=EDGE_CURVE('',#42532,#42683,#6556,.T.);
#56213=EDGE_CURVE('',#42684,#42528,#6557,.T.);
#56214=EDGE_CURVE('',#42685,#42684,#34768,.T.);
#56215=EDGE_CURVE('',#42516,#42685,#6558,.T.);
#56216=EDGE_CURVE('',#42686,#42544,#6559,.T.);
#56217=EDGE_CURVE('',#42687,#42686,#34769,.T.);
#56218=EDGE_CURVE('',#42523,#42687,#6560,.T.);
#56219=EDGE_CURVE('',#42688,#42529,#6561,.T.);
#56220=EDGE_CURVE('',#42689,#42688,#34770,.T.);
#56221=EDGE_CURVE('',#42690,#42689,#6562,.T.);
#56222=EDGE_CURVE('',#42594,#42690,#6563,.T.);
#56223=EDGE_CURVE('',#42691,#42692,#6564,.T.);
#56224=EDGE_CURVE('',#42693,#42691,#34771,.T.);
#56225=EDGE_CURVE('',#42694,#42693,#6565,.T.);
#56226=EDGE_CURVE('',#42596,#42694,#6566,.T.);
#56227=EDGE_CURVE('',#42692,#42595,#6567,.T.);
#56228=EDGE_CURVE('',#42695,#42552,#6568,.T.);
#56229=EDGE_CURVE('',#42696,#42695,#34772,.T.);
#56230=EDGE_CURVE('',#42539,#42696,#6569,.T.);
#56231=EDGE_CURVE('',#42697,#42560,#6570,.T.);
#56232=EDGE_CURVE('',#42698,#42697,#34773,.T.);
#56233=EDGE_CURVE('',#42547,#42698,#6571,.T.);
#56234=EDGE_CURVE('',#42699,#42615,#24325,.T.);
#56235=EDGE_CURVE('',#42700,#42699,#34774,.T.);
#56236=EDGE_CURVE('',#42617,#42700,#24326,.T.);
#56237=EDGE_CURVE('',#42622,#42701,#24327,.T.);
#56238=EDGE_CURVE('',#42702,#42621,#24328,.T.);
#56239=EDGE_CURVE('',#42701,#42702,#34775,.T.);
#56240=EDGE_CURVE('',#42626,#42703,#24329,.T.);
#56241=EDGE_CURVE('',#42704,#42625,#24330,.T.);
#56242=EDGE_CURVE('',#42703,#42704,#34776,.T.);
#56243=EDGE_CURVE('',#42630,#42705,#24331,.T.);
#56244=EDGE_CURVE('',#42706,#42629,#24332,.T.);
#56245=EDGE_CURVE('',#42705,#42706,#34777,.T.);
#56246=EDGE_CURVE('',#42707,#42631,#24333,.T.);
#56247=EDGE_CURVE('',#42708,#42707,#34778,.T.);
#56248=EDGE_CURVE('',#42633,#42708,#24334,.T.);
#56249=EDGE_CURVE('',#42709,#42636,#24335,.T.);
#56250=EDGE_CURVE('',#42459,#42709,#34779,.T.);
#56251=EDGE_CURVE('',#42640,#42710,#24336,.T.);
#56252=EDGE_CURVE('',#42711,#42639,#24337,.T.);
#56253=EDGE_CURVE('',#42710,#42711,#34780,.T.);
#56254=EDGE_CURVE('',#42712,#42641,#24338,.T.);
#56255=EDGE_CURVE('',#42713,#42712,#34781,.T.);
#56256=EDGE_CURVE('',#42643,#42713,#24339,.T.);
#56257=EDGE_CURVE('',#42648,#42714,#24340,.T.);
#56258=EDGE_CURVE('',#42715,#42647,#24341,.T.);
#56259=EDGE_CURVE('',#42714,#42715,#34782,.T.);
#56260=EDGE_CURVE('',#42650,#42716,#24342,.T.);
#56261=EDGE_CURVE('',#42716,#42464,#34783,.T.);
#56262=EDGE_CURVE('',#42717,#42651,#24343,.T.);
#56263=EDGE_CURVE('',#42718,#42717,#34784,.T.);
#56264=EDGE_CURVE('',#42653,#42718,#24344,.T.);
#56265=EDGE_CURVE('',#42658,#42719,#24345,.T.);
#56266=EDGE_CURVE('',#42720,#42657,#24346,.T.);
#56267=EDGE_CURVE('',#42719,#42720,#34785,.T.);
#56268=EDGE_CURVE('',#42721,#42659,#24347,.T.);
#56269=EDGE_CURVE('',#42722,#42721,#34786,.T.);
#56270=EDGE_CURVE('',#42661,#42722,#24348,.T.);
#56271=EDGE_CURVE('',#42666,#42723,#24349,.T.);
#56272=EDGE_CURVE('',#42724,#42665,#24350,.T.);
#56273=EDGE_CURVE('',#42723,#42724,#34787,.T.);
#56274=EDGE_CURVE('',#42725,#42667,#24351,.T.);
#56275=EDGE_CURVE('',#42726,#42725,#34788,.T.);
#56276=EDGE_CURVE('',#42668,#42726,#24352,.T.);
#56277=EDGE_CURVE('',#42670,#42727,#24353,.T.);
#56278=EDGE_CURVE('',#42728,#42669,#24354,.T.);
#56279=EDGE_CURVE('',#42727,#42728,#34789,.T.);
#56280=EDGE_CURVE('',#42672,#42729,#24355,.T.);
#56281=EDGE_CURVE('',#42730,#42671,#24356,.T.);
#56282=EDGE_CURVE('',#42729,#42730,#34790,.T.);
#56283=EDGE_CURVE('',#42731,#42673,#24357,.T.);
#56284=EDGE_CURVE('',#42732,#42731,#34791,.T.);
#56285=EDGE_CURVE('',#42674,#42732,#24358,.T.);
#56286=EDGE_CURVE('',#42676,#42733,#24359,.T.);
#56287=EDGE_CURVE('',#42734,#42675,#24360,.T.);
#56288=EDGE_CURVE('',#42733,#42734,#34792,.T.);
#56289=EDGE_CURVE('',#42735,#42677,#24361,.T.);
#56290=EDGE_CURVE('',#42736,#42735,#34793,.T.);
#56291=EDGE_CURVE('',#42678,#42736,#24362,.T.);
#56292=EDGE_CURVE('',#42681,#42737,#24363,.T.);
#56293=EDGE_CURVE('',#42738,#42680,#24364,.T.);
#56294=EDGE_CURVE('',#42737,#42738,#34794,.T.);
#56295=EDGE_CURVE('',#42739,#42682,#24365,.T.);
#56296=EDGE_CURVE('',#42740,#42739,#34795,.T.);
#56297=EDGE_CURVE('',#42683,#42740,#24366,.T.);
#56298=EDGE_CURVE('',#42685,#42741,#24367,.T.);
#56299=EDGE_CURVE('',#42742,#42684,#24368,.T.);
#56300=EDGE_CURVE('',#42741,#42742,#34796,.T.);
#56301=EDGE_CURVE('',#42687,#42743,#24369,.T.);
#56302=EDGE_CURVE('',#42744,#42686,#24370,.T.);
#56303=EDGE_CURVE('',#42743,#42744,#34797,.T.);
#56304=EDGE_CURVE('',#42745,#42688,#24371,.T.);
#56305=EDGE_CURVE('',#42746,#42745,#34798,.T.);
#56306=EDGE_CURVE('',#42689,#42746,#24372,.T.);
#56307=EDGE_CURVE('',#42747,#42691,#24373,.T.);
#56308=EDGE_CURVE('',#42748,#42747,#34799,.T.);
#56309=EDGE_CURVE('',#42693,#42748,#24374,.T.);
#56310=EDGE_CURVE('',#42696,#42749,#24375,.T.);
#56311=EDGE_CURVE('',#42750,#42695,#24376,.T.);
#56312=EDGE_CURVE('',#42749,#42750,#34800,.T.);
#56313=EDGE_CURVE('',#42698,#42751,#24377,.T.);
#56314=EDGE_CURVE('',#42752,#42697,#24378,.T.);
#56315=EDGE_CURVE('',#42751,#42752,#34801,.T.);
#56316=EDGE_CURVE('',#42753,#42699,#6572,.T.);
#56317=EDGE_CURVE('',#42754,#42753,#6573,.T.);
#56318=EDGE_CURVE('',#42755,#42754,#34802,.T.);
#56319=EDGE_CURVE('',#42756,#42755,#6574,.T.);
#56320=EDGE_CURVE('',#42700,#42756,#6575,.T.);
#56321=EDGE_CURVE('',#42757,#42758,#6576,.T.);
#56322=EDGE_CURVE('',#42701,#42757,#6577,.T.);
#56323=EDGE_CURVE('',#42759,#42702,#6578,.T.);
#56324=EDGE_CURVE('',#42760,#42759,#6579,.T.);
#56325=EDGE_CURVE('',#42758,#42760,#34803,.T.);
#56326=EDGE_CURVE('',#42761,#42762,#6580,.T.);
#56327=EDGE_CURVE('',#42703,#42761,#6581,.T.);
#56328=EDGE_CURVE('',#42763,#42704,#6582,.T.);
#56329=EDGE_CURVE('',#42764,#42763,#6583,.T.);
#56330=EDGE_CURVE('',#42762,#42764,#34804,.T.);
#56331=EDGE_CURVE('',#42765,#42766,#6584,.T.);
#56332=EDGE_CURVE('',#42705,#42765,#6585,.T.);
#56333=EDGE_CURVE('',#42767,#42706,#6586,.T.);
#56334=EDGE_CURVE('',#42768,#42767,#6587,.T.);
#56335=EDGE_CURVE('',#42766,#42768,#34805,.T.);
#56336=EDGE_CURVE('',#42769,#42707,#6588,.T.);
#56337=EDGE_CURVE('',#42770,#42769,#6589,.T.);
#56338=EDGE_CURVE('',#42771,#42770,#34806,.T.);
#56339=EDGE_CURVE('',#42772,#42771,#6590,.T.);
#56340=EDGE_CURVE('',#42708,#42772,#6591,.T.);
#56341=EDGE_CURVE('',#42460,#42773,#6592,.T.);
#56342=EDGE_CURVE('',#42774,#42709,#6593,.T.);
#56343=EDGE_CURVE('',#42775,#42774,#6594,.T.);
#56344=EDGE_CURVE('',#42773,#42775,#34807,.T.);
#56345=EDGE_CURVE('',#42776,#42777,#6595,.T.);
#56346=EDGE_CURVE('',#42710,#42776,#6596,.T.);
#56347=EDGE_CURVE('',#42778,#42711,#6597,.T.);
#56348=EDGE_CURVE('',#42779,#42778,#6598,.T.);
#56349=EDGE_CURVE('',#42777,#42779,#34808,.T.);
#56350=EDGE_CURVE('',#42780,#42712,#6599,.T.);
#56351=EDGE_CURVE('',#42781,#42780,#6600,.T.);
#56352=EDGE_CURVE('',#42782,#42781,#34809,.T.);
#56353=EDGE_CURVE('',#42783,#42782,#6601,.T.);
#56354=EDGE_CURVE('',#42713,#42783,#6602,.T.);
#56355=EDGE_CURVE('',#42784,#42785,#6603,.T.);
#56356=EDGE_CURVE('',#42714,#42784,#6604,.T.);
#56357=EDGE_CURVE('',#42786,#42715,#6605,.T.);
#56358=EDGE_CURVE('',#42787,#42786,#6606,.T.);
#56359=EDGE_CURVE('',#42785,#42787,#34810,.T.);
#56360=EDGE_CURVE('',#42788,#42789,#6607,.T.);
#56361=EDGE_CURVE('',#42716,#42788,#6608,.T.);
#56362=EDGE_CURVE('',#42790,#42463,#6609,.T.);
#56363=EDGE_CURVE('',#42789,#42790,#34811,.T.);
#56364=EDGE_CURVE('',#42791,#42717,#6610,.T.);
#56365=EDGE_CURVE('',#42792,#42791,#6611,.T.);
#56366=EDGE_CURVE('',#42793,#42792,#34812,.T.);
#56367=EDGE_CURVE('',#42794,#42793,#6612,.T.);
#56368=EDGE_CURVE('',#42718,#42794,#6613,.T.);
#56369=EDGE_CURVE('',#42795,#42796,#6614,.T.);
#56370=EDGE_CURVE('',#42719,#42795,#6615,.T.);
#56371=EDGE_CURVE('',#42797,#42720,#6616,.T.);
#56372=EDGE_CURVE('',#42798,#42797,#6617,.T.);
#56373=EDGE_CURVE('',#42796,#42798,#34813,.T.);
#56374=EDGE_CURVE('',#42799,#42721,#6618,.T.);
#56375=EDGE_CURVE('',#42800,#42799,#6619,.T.);
#56376=EDGE_CURVE('',#42801,#42800,#34814,.T.);
#56377=EDGE_CURVE('',#42802,#42801,#6620,.T.);
#56378=EDGE_CURVE('',#42722,#42802,#6621,.T.);
#56379=EDGE_CURVE('',#42803,#42804,#6622,.T.);
#56380=EDGE_CURVE('',#42723,#42803,#6623,.T.);
#56381=EDGE_CURVE('',#42805,#42724,#6624,.T.);
#56382=EDGE_CURVE('',#42806,#42805,#6625,.T.);
#56383=EDGE_CURVE('',#42804,#42806,#34815,.T.);
#56384=EDGE_CURVE('',#42471,#42725,#6626,.T.);
#56385=EDGE_CURVE('',#42557,#42470,#34816,.T.);
#56386=EDGE_CURVE('',#42726,#42556,#6627,.T.);
#56387=EDGE_CURVE('',#42727,#42468,#6628,.T.);
#56388=EDGE_CURVE('',#42479,#42728,#6629,.T.);
#56389=EDGE_CURVE('',#42469,#42478,#34817,.T.);
#56390=EDGE_CURVE('',#42729,#42476,#6630,.T.);
#56391=EDGE_CURVE('',#42495,#42730,#6631,.T.);
#56392=EDGE_CURVE('',#42477,#42494,#34818,.T.);
#56393=EDGE_CURVE('',#42487,#42731,#6632,.T.);
#56394=EDGE_CURVE('',#42493,#42486,#34819,.T.);
#56395=EDGE_CURVE('',#42732,#42492,#6633,.T.);
#56396=EDGE_CURVE('',#42733,#42484,#6634,.T.);
#56397=EDGE_CURVE('',#42510,#42734,#6635,.T.);
#56398=EDGE_CURVE('',#42485,#42509,#34820,.T.);
#56399=EDGE_CURVE('',#42502,#42735,#6636,.T.);
#56400=EDGE_CURVE('',#42508,#42501,#34821,.T.);
#56401=EDGE_CURVE('',#42736,#42507,#6637,.T.);
#56402=EDGE_CURVE('',#42737,#42499,#6638,.T.);
#56403=EDGE_CURVE('',#42807,#42738,#6639,.T.);
#56404=EDGE_CURVE('',#42808,#42807,#6640,.T.);
#56405=EDGE_CURVE('',#42500,#42808,#34822,.T.);
#56406=EDGE_CURVE('',#42520,#42739,#6641,.T.);
#56407=EDGE_CURVE('',#42534,#42519,#34823,.T.);
#56408=EDGE_CURVE('',#42740,#42533,#6642,.T.);
#56409=EDGE_CURVE('',#42741,#42517,#6643,.T.);
#56410=EDGE_CURVE('',#42527,#42742,#6644,.T.);
#56411=EDGE_CURVE('',#42518,#42526,#34824,.T.);
#56412=EDGE_CURVE('',#42743,#42524,#6645,.T.);
#56413=EDGE_CURVE('',#42543,#42744,#6646,.T.);
#56414=EDGE_CURVE('',#42525,#42542,#34825,.T.);
#56415=EDGE_CURVE('',#42536,#42745,#6647,.T.);
#56416=EDGE_CURVE('',#42809,#42535,#34826,.T.);
#56417=EDGE_CURVE('',#42810,#42809,#6648,.T.);
#56418=EDGE_CURVE('',#42746,#42810,#6649,.T.);
#56419=EDGE_CURVE('',#42811,#42747,#6650,.T.);
#56420=EDGE_CURVE('',#42812,#42811,#6651,.T.);
#56421=EDGE_CURVE('',#42813,#42812,#34827,.T.);
#56422=EDGE_CURVE('',#42814,#42813,#6652,.T.);
#56423=EDGE_CURVE('',#42748,#42814,#6653,.T.);
#56424=EDGE_CURVE('',#42749,#42540,#6654,.T.);
#56425=EDGE_CURVE('',#42551,#42750,#6655,.T.);
#56426=EDGE_CURVE('',#42541,#42550,#34828,.T.);
#56427=EDGE_CURVE('',#42751,#42548,#6656,.T.);
#56428=EDGE_CURVE('',#42559,#42752,#6657,.T.);
#56429=EDGE_CURVE('',#42549,#42558,#34829,.T.);
#56430=EDGE_CURVE('',#42598,#42815,#6658,.T.);
#56431=EDGE_CURVE('',#42816,#42597,#6659,.T.);
#56432=EDGE_CURVE('',#42817,#42816,#6660,.T.);
#56433=EDGE_CURVE('',#42818,#42817,#34830,.T.);
#56434=EDGE_CURVE('',#42815,#42818,#6661,.T.);
#56435=EDGE_CURVE('',#42818,#42819,#24379,.T.);
#56436=EDGE_CURVE('',#42820,#42817,#24380,.T.);
#56437=EDGE_CURVE('',#42819,#42820,#34831,.T.);
#56438=EDGE_CURVE('',#42821,#42822,#6662,.T.);
#56439=EDGE_CURVE('',#42819,#42821,#6663,.T.);
#56440=EDGE_CURVE('',#42823,#42820,#6664,.T.);
#56441=EDGE_CURVE('',#42824,#42823,#6665,.T.);
#56442=EDGE_CURVE('',#42822,#42824,#34832,.T.);
#56443=EDGE_CURVE('',#42565,#42754,#34833,.T.);
#56444=EDGE_CURVE('',#42758,#42564,#34834,.T.);
#56445=EDGE_CURVE('',#42762,#42760,#34835,.T.);
#56446=EDGE_CURVE('',#42766,#42764,#34836,.T.);
#56447=EDGE_CURVE('',#42777,#42768,#34837,.T.);
#56448=EDGE_CURVE('',#42771,#42779,#34838,.T.);
#56449=EDGE_CURVE('',#42773,#42770,#34839,.T.);
#56450=EDGE_CURVE('',#42822,#42775,#34840,.T.);
#56451=EDGE_CURVE('',#42813,#42824,#34841,.T.);
#56452=EDGE_CURVE('',#42809,#42812,#34842,.T.);
#56453=EDGE_CURVE('',#42782,#42808,#34843,.T.);
#56454=EDGE_CURVE('',#42785,#42781,#34844,.T.);
#56455=EDGE_CURVE('',#42789,#42787,#34845,.T.);
#56456=EDGE_CURVE('',#42793,#42790,#34846,.T.);
#56457=EDGE_CURVE('',#42796,#42792,#34847,.T.);
#56458=EDGE_CURVE('',#42801,#42798,#34848,.T.);
#56459=EDGE_CURVE('',#42804,#42800,#34849,.T.);
#56460=EDGE_CURVE('',#42755,#42806,#34850,.T.);
#56461=EDGE_CURVE('',#42816,#42823,#24381,.T.);
#56462=EDGE_CURVE('',#42694,#42814,#24382,.T.);
#56463=EDGE_CURVE('',#42635,#42774,#24383,.T.);
#56464=EDGE_CURVE('',#42815,#42821,#24384,.T.);
#56465=EDGE_CURVE('',#42692,#42811,#24385,.T.);
#56466=EDGE_CURVE('',#42690,#42810,#24386,.T.);
#56467=EDGE_CURVE('',#42679,#42807,#24387,.T.);
#56468=EDGE_CURVE('',#42644,#42783,#24388,.T.);
#56469=EDGE_CURVE('',#42664,#42805,#24389,.T.);
#56470=EDGE_CURVE('',#42618,#42756,#24390,.T.);
#56471=EDGE_CURVE('',#42656,#42797,#24391,.T.);
#56472=EDGE_CURVE('',#42662,#42802,#24392,.T.);
#56473=EDGE_CURVE('',#42660,#42799,#24393,.T.);
#56474=EDGE_CURVE('',#42663,#42803,#24394,.T.);
#56475=EDGE_CURVE('',#42654,#42794,#24395,.T.);
#56476=EDGE_CURVE('',#42652,#42791,#24396,.T.);
#56477=EDGE_CURVE('',#42655,#42795,#24397,.T.);
#56478=EDGE_CURVE('',#42646,#42786,#24398,.T.);
#56479=EDGE_CURVE('',#42649,#42788,#24399,.T.);
#56480=EDGE_CURVE('',#42642,#42780,#24400,.T.);
#56481=EDGE_CURVE('',#42645,#42784,#24401,.T.);
#56482=EDGE_CURVE('',#42638,#42778,#24402,.T.);
#56483=EDGE_CURVE('',#42634,#42772,#24403,.T.);
#56484=EDGE_CURVE('',#42628,#42767,#24404,.T.);
#56485=EDGE_CURVE('',#42637,#42776,#24405,.T.);
#56486=EDGE_CURVE('',#42632,#42769,#24406,.T.);
#56487=EDGE_CURVE('',#42624,#42763,#24407,.T.);
#56488=EDGE_CURVE('',#42627,#42765,#24408,.T.);
#56489=EDGE_CURVE('',#42620,#42759,#24409,.T.);
#56490=EDGE_CURVE('',#42623,#42761,#24410,.T.);
#56491=EDGE_CURVE('',#42571,#42563,#24411,.T.);
#56492=EDGE_CURVE('',#42619,#42757,#24412,.T.);
#56493=EDGE_CURVE('',#42616,#42753,#24413,.T.);
#56494=EDGE_CURVE('',#42572,#42566,#24414,.T.);
#56495=EDGE_CURVE('',#42612,#42614,#24415,.T.);
#56496=EDGE_CURVE('',#42611,#42613,#24416,.T.);
#82321=ORIENTED_EDGE('',*,*,#55940,.F.);
#82322=ORIENTED_EDGE('',*,*,#55941,.T.);
#82323=ORIENTED_EDGE('',*,*,#55942,.F.);
#82324=ORIENTED_EDGE('',*,*,#55941,.F.);
#82325=ORIENTED_EDGE('',*,*,#55942,.T.);
#82326=ORIENTED_EDGE('',*,*,#55943,.T.);
#82327=ORIENTED_EDGE('',*,*,#55944,.F.);
#82328=ORIENTED_EDGE('',*,*,#55943,.F.);
#82329=ORIENTED_EDGE('',*,*,#55945,.T.);
#82330=ORIENTED_EDGE('',*,*,#55946,.T.);
#82331=ORIENTED_EDGE('',*,*,#55947,.T.);
#82332=ORIENTED_EDGE('',*,*,#55948,.F.);
#82333=ORIENTED_EDGE('',*,*,#55949,.T.);
#82334=ORIENTED_EDGE('',*,*,#55950,.T.);
#82335=ORIENTED_EDGE('',*,*,#55951,.T.);
#82336=ORIENTED_EDGE('',*,*,#55952,.T.);
#82337=ORIENTED_EDGE('',*,*,#55953,.T.);
#82338=ORIENTED_EDGE('',*,*,#55954,.T.);
#82339=ORIENTED_EDGE('',*,*,#55955,.T.);
#82340=ORIENTED_EDGE('',*,*,#55956,.T.);
#82341=ORIENTED_EDGE('',*,*,#55957,.T.);
#82342=ORIENTED_EDGE('',*,*,#55958,.T.);
#82343=ORIENTED_EDGE('',*,*,#55959,.F.);
#82344=ORIENTED_EDGE('',*,*,#55960,.T.);
#82345=ORIENTED_EDGE('',*,*,#55961,.T.);
#82346=ORIENTED_EDGE('',*,*,#55962,.T.);
#82347=ORIENTED_EDGE('',*,*,#55963,.T.);
#82348=ORIENTED_EDGE('',*,*,#55964,.T.);
#82349=ORIENTED_EDGE('',*,*,#55965,.T.);
#82350=ORIENTED_EDGE('',*,*,#55966,.T.);
#82351=ORIENTED_EDGE('',*,*,#55967,.F.);
#82352=ORIENTED_EDGE('',*,*,#55968,.T.);
#82353=ORIENTED_EDGE('',*,*,#55969,.T.);
#82354=ORIENTED_EDGE('',*,*,#55970,.T.);
#82355=ORIENTED_EDGE('',*,*,#55971,.T.);
#82356=ORIENTED_EDGE('',*,*,#55972,.T.);
#82357=ORIENTED_EDGE('',*,*,#55973,.T.);
#82358=ORIENTED_EDGE('',*,*,#55974,.T.);
#82359=ORIENTED_EDGE('',*,*,#55975,.F.);
#82360=ORIENTED_EDGE('',*,*,#55976,.T.);
#82361=ORIENTED_EDGE('',*,*,#55977,.T.);
#82362=ORIENTED_EDGE('',*,*,#55978,.T.);
#82363=ORIENTED_EDGE('',*,*,#55979,.T.);
#82364=ORIENTED_EDGE('',*,*,#55980,.T.);
#82365=ORIENTED_EDGE('',*,*,#55981,.T.);
#82366=ORIENTED_EDGE('',*,*,#55982,.T.);
#82367=ORIENTED_EDGE('',*,*,#55983,.F.);
#82368=ORIENTED_EDGE('',*,*,#55984,.T.);
#82369=ORIENTED_EDGE('',*,*,#55985,.T.);
#82370=ORIENTED_EDGE('',*,*,#55986,.T.);
#82371=ORIENTED_EDGE('',*,*,#55987,.T.);
#82372=ORIENTED_EDGE('',*,*,#55988,.T.);
#82373=ORIENTED_EDGE('',*,*,#55989,.T.);
#82374=ORIENTED_EDGE('',*,*,#55990,.F.);
#82375=ORIENTED_EDGE('',*,*,#55991,.T.);
#82376=ORIENTED_EDGE('',*,*,#55992,.T.);
#82377=ORIENTED_EDGE('',*,*,#55993,.T.);
#82378=ORIENTED_EDGE('',*,*,#55994,.T.);
#82379=ORIENTED_EDGE('',*,*,#55995,.T.);
#82380=ORIENTED_EDGE('',*,*,#55996,.T.);
#82381=ORIENTED_EDGE('',*,*,#55997,.T.);
#82382=ORIENTED_EDGE('',*,*,#55998,.F.);
#82383=ORIENTED_EDGE('',*,*,#55999,.T.);
#82384=ORIENTED_EDGE('',*,*,#56000,.T.);
#82385=ORIENTED_EDGE('',*,*,#56001,.T.);
#82386=ORIENTED_EDGE('',*,*,#56002,.T.);
#82387=ORIENTED_EDGE('',*,*,#56003,.T.);
#82388=ORIENTED_EDGE('',*,*,#56004,.T.);
#82389=ORIENTED_EDGE('',*,*,#56005,.T.);
#82390=ORIENTED_EDGE('',*,*,#56006,.T.);
#82391=ORIENTED_EDGE('',*,*,#56007,.T.);
#82392=ORIENTED_EDGE('',*,*,#56008,.F.);
#82393=ORIENTED_EDGE('',*,*,#56009,.T.);
#82394=ORIENTED_EDGE('',*,*,#56010,.T.);
#82395=ORIENTED_EDGE('',*,*,#56011,.T.);
#82396=ORIENTED_EDGE('',*,*,#56012,.T.);
#82397=ORIENTED_EDGE('',*,*,#56013,.T.);
#82398=ORIENTED_EDGE('',*,*,#56014,.T.);
#82399=ORIENTED_EDGE('',*,*,#56015,.F.);
#82400=ORIENTED_EDGE('',*,*,#56016,.T.);
#82401=ORIENTED_EDGE('',*,*,#56017,.T.);
#82402=ORIENTED_EDGE('',*,*,#56018,.T.);
#82403=ORIENTED_EDGE('',*,*,#56019,.T.);
#82404=ORIENTED_EDGE('',*,*,#56020,.T.);
#82405=ORIENTED_EDGE('',*,*,#56021,.T.);
#82406=ORIENTED_EDGE('',*,*,#56022,.T.);
#82407=ORIENTED_EDGE('',*,*,#56023,.T.);
#82408=ORIENTED_EDGE('',*,*,#56024,.F.);
#82409=ORIENTED_EDGE('',*,*,#56025,.T.);
#82410=ORIENTED_EDGE('',*,*,#56026,.T.);
#82411=ORIENTED_EDGE('',*,*,#56027,.T.);
#82412=ORIENTED_EDGE('',*,*,#56028,.T.);
#82413=ORIENTED_EDGE('',*,*,#56029,.T.);
#82414=ORIENTED_EDGE('',*,*,#56030,.T.);
#82415=ORIENTED_EDGE('',*,*,#56031,.F.);
#82416=ORIENTED_EDGE('',*,*,#56032,.T.);
#82417=ORIENTED_EDGE('',*,*,#56033,.T.);
#82418=ORIENTED_EDGE('',*,*,#56034,.T.);
#82419=ORIENTED_EDGE('',*,*,#56035,.T.);
#82420=ORIENTED_EDGE('',*,*,#56036,.T.);
#82421=ORIENTED_EDGE('',*,*,#56037,.T.);
#82422=ORIENTED_EDGE('',*,*,#56038,.T.);
#82423=ORIENTED_EDGE('',*,*,#56039,.F.);
#82424=ORIENTED_EDGE('',*,*,#56040,.T.);
#82425=ORIENTED_EDGE('',*,*,#56041,.T.);
#82426=ORIENTED_EDGE('',*,*,#56042,.T.);
#82427=ORIENTED_EDGE('',*,*,#56043,.T.);
#82428=ORIENTED_EDGE('',*,*,#56044,.T.);
#82429=ORIENTED_EDGE('',*,*,#56045,.T.);
#82430=ORIENTED_EDGE('',*,*,#56046,.T.);
#82431=ORIENTED_EDGE('',*,*,#56047,.F.);
#82432=ORIENTED_EDGE('',*,*,#56048,.T.);
#82433=ORIENTED_EDGE('',*,*,#56049,.T.);
#82434=ORIENTED_EDGE('',*,*,#56050,.F.);
#82435=ORIENTED_EDGE('',*,*,#56051,.F.);
#82436=ORIENTED_EDGE('',*,*,#56052,.F.);
#82437=ORIENTED_EDGE('',*,*,#56053,.F.);
#82438=ORIENTED_EDGE('',*,*,#56054,.F.);
#82439=ORIENTED_EDGE('',*,*,#56055,.T.);
#82440=ORIENTED_EDGE('',*,*,#56056,.F.);
#82441=ORIENTED_EDGE('',*,*,#56049,.F.);
#82442=ORIENTED_EDGE('',*,*,#56057,.F.);
#82443=ORIENTED_EDGE('',*,*,#56058,.T.);
#82444=ORIENTED_EDGE('',*,*,#56059,.F.);
#82445=ORIENTED_EDGE('',*,*,#56060,.F.);
#82446=ORIENTED_EDGE('',*,*,#56055,.F.);
#82447=ORIENTED_EDGE('',*,*,#56061,.F.);
#82448=ORIENTED_EDGE('',*,*,#56062,.F.);
#82449=ORIENTED_EDGE('',*,*,#56063,.T.);
#82450=ORIENTED_EDGE('',*,*,#56064,.T.);
#82451=ORIENTED_EDGE('',*,*,#56065,.F.);
#82452=ORIENTED_EDGE('',*,*,#56066,.T.);
#82453=ORIENTED_EDGE('',*,*,#56067,.F.);
#82454=ORIENTED_EDGE('',*,*,#56068,.F.);
#82455=ORIENTED_EDGE('',*,*,#56069,.F.);
#82456=ORIENTED_EDGE('',*,*,#56070,.F.);
#82457=ORIENTED_EDGE('',*,*,#56071,.F.);
#82458=ORIENTED_EDGE('',*,*,#56072,.F.);
#82459=ORIENTED_EDGE('',*,*,#56073,.F.);
#82460=ORIENTED_EDGE('',*,*,#56074,.F.);
#82461=ORIENTED_EDGE('',*,*,#56075,.F.);
#82462=ORIENTED_EDGE('',*,*,#56076,.F.);
#82463=ORIENTED_EDGE('',*,*,#56077,.F.);
#82464=ORIENTED_EDGE('',*,*,#56078,.F.);
#82465=ORIENTED_EDGE('',*,*,#56079,.F.);
#82466=ORIENTED_EDGE('',*,*,#56080,.F.);
#82467=ORIENTED_EDGE('',*,*,#56081,.F.);
#82468=ORIENTED_EDGE('',*,*,#56082,.F.);
#82469=ORIENTED_EDGE('',*,*,#56083,.F.);
#82470=ORIENTED_EDGE('',*,*,#56084,.F.);
#82471=ORIENTED_EDGE('',*,*,#55992,.F.);
#82472=ORIENTED_EDGE('',*,*,#56085,.F.);
#82473=ORIENTED_EDGE('',*,*,#56000,.F.);
#82474=ORIENTED_EDGE('',*,*,#56086,.F.);
#82475=ORIENTED_EDGE('',*,*,#55969,.F.);
#82476=ORIENTED_EDGE('',*,*,#56087,.F.);
#82477=ORIENTED_EDGE('',*,*,#55977,.F.);
#82478=ORIENTED_EDGE('',*,*,#56088,.F.);
#82479=ORIENTED_EDGE('',*,*,#55961,.F.);
#82480=ORIENTED_EDGE('',*,*,#56089,.F.);
#82481=ORIENTED_EDGE('',*,*,#55953,.F.);
#82482=ORIENTED_EDGE('',*,*,#56090,.F.);
#82483=ORIENTED_EDGE('',*,*,#56041,.F.);
#82484=ORIENTED_EDGE('',*,*,#56091,.F.);
#82485=ORIENTED_EDGE('',*,*,#56033,.F.);
#82486=ORIENTED_EDGE('',*,*,#56092,.F.);
#82487=ORIENTED_EDGE('',*,*,#56025,.F.);
#82488=ORIENTED_EDGE('',*,*,#56093,.F.);
#82489=ORIENTED_EDGE('',*,*,#56009,.F.);
#82490=ORIENTED_EDGE('',*,*,#56094,.F.);
#82491=ORIENTED_EDGE('',*,*,#56002,.F.);
#82492=ORIENTED_EDGE('',*,*,#56095,.F.);
#82493=ORIENTED_EDGE('',*,*,#56018,.F.);
#82494=ORIENTED_EDGE('',*,*,#56096,.F.);
#82495=ORIENTED_EDGE('',*,*,#56097,.F.);
#82496=ORIENTED_EDGE('',*,*,#56098,.F.);
#82497=ORIENTED_EDGE('',*,*,#56099,.F.);
#82498=ORIENTED_EDGE('',*,*,#56100,.F.);
#82499=ORIENTED_EDGE('',*,*,#56101,.F.);
#82500=ORIENTED_EDGE('',*,*,#56102,.F.);
#82501=ORIENTED_EDGE('',*,*,#56103,.F.);
#82502=ORIENTED_EDGE('',*,*,#56104,.F.);
#82503=ORIENTED_EDGE('',*,*,#56105,.F.);
#82504=ORIENTED_EDGE('',*,*,#56106,.F.);
#82505=ORIENTED_EDGE('',*,*,#56107,.F.);
#82506=ORIENTED_EDGE('',*,*,#56108,.F.);
#82507=ORIENTED_EDGE('',*,*,#56109,.F.);
#82508=ORIENTED_EDGE('',*,*,#56110,.F.);
#82509=ORIENTED_EDGE('',*,*,#56111,.F.);
#82510=ORIENTED_EDGE('',*,*,#56112,.F.);
#82511=ORIENTED_EDGE('',*,*,#56113,.F.);
#82512=ORIENTED_EDGE('',*,*,#56058,.F.);
#82513=ORIENTED_EDGE('',*,*,#56114,.F.);
#82514=ORIENTED_EDGE('',*,*,#56063,.F.);
#82515=ORIENTED_EDGE('',*,*,#56115,.F.);
#82516=ORIENTED_EDGE('',*,*,#56116,.F.);
#82517=ORIENTED_EDGE('',*,*,#55944,.T.);
#82518=ORIENTED_EDGE('',*,*,#56065,.T.);
#82519=ORIENTED_EDGE('',*,*,#56117,.T.);
#82520=ORIENTED_EDGE('',*,*,#56118,.T.);
#82521=ORIENTED_EDGE('',*,*,#56119,.T.);
#82522=ORIENTED_EDGE('',*,*,#56120,.F.);
#82523=ORIENTED_EDGE('',*,*,#56121,.F.);
#82524=ORIENTED_EDGE('',*,*,#56122,.F.);
#82525=ORIENTED_EDGE('',*,*,#56123,.F.);
#82526=ORIENTED_EDGE('',*,*,#56068,.T.);
#82527=ORIENTED_EDGE('',*,*,#56124,.F.);
#82528=ORIENTED_EDGE('',*,*,#56125,.F.);
#82529=ORIENTED_EDGE('',*,*,#56112,.T.);
#82530=ORIENTED_EDGE('',*,*,#56126,.F.);
#82531=ORIENTED_EDGE('',*,*,#56127,.F.);
#82532=ORIENTED_EDGE('',*,*,#56128,.F.);
#82533=ORIENTED_EDGE('',*,*,#56129,.F.);
#82534=ORIENTED_EDGE('',*,*,#56130,.F.);
#82535=ORIENTED_EDGE('',*,*,#56110,.T.);
#82536=ORIENTED_EDGE('',*,*,#56131,.F.);
#82537=ORIENTED_EDGE('',*,*,#56132,.F.);
#82538=ORIENTED_EDGE('',*,*,#56133,.F.);
#82539=ORIENTED_EDGE('',*,*,#56134,.F.);
#82540=ORIENTED_EDGE('',*,*,#56135,.F.);
#82541=ORIENTED_EDGE('',*,*,#56108,.T.);
#82542=ORIENTED_EDGE('',*,*,#56136,.F.);
#82543=ORIENTED_EDGE('',*,*,#56137,.F.);
#82544=ORIENTED_EDGE('',*,*,#56138,.F.);
#82545=ORIENTED_EDGE('',*,*,#56139,.F.);
#82546=ORIENTED_EDGE('',*,*,#56140,.F.);
#82547=ORIENTED_EDGE('',*,*,#56141,.F.);
#82548=ORIENTED_EDGE('',*,*,#56142,.F.);
#82549=ORIENTED_EDGE('',*,*,#56143,.F.);
#82550=ORIENTED_EDGE('',*,*,#56104,.T.);
#82551=ORIENTED_EDGE('',*,*,#56144,.F.);
#82552=ORIENTED_EDGE('',*,*,#56145,.F.);
#82553=ORIENTED_EDGE('',*,*,#56102,.T.);
#82554=ORIENTED_EDGE('',*,*,#56146,.F.);
#82555=ORIENTED_EDGE('',*,*,#56147,.F.);
#82556=ORIENTED_EDGE('',*,*,#56148,.F.);
#82557=ORIENTED_EDGE('',*,*,#55945,.F.);
#82558=ORIENTED_EDGE('',*,*,#56149,.F.);
#82559=ORIENTED_EDGE('',*,*,#56106,.T.);
#82560=ORIENTED_EDGE('',*,*,#56150,.F.);
#82561=ORIENTED_EDGE('',*,*,#56151,.F.);
#82562=ORIENTED_EDGE('',*,*,#56152,.F.);
#82563=ORIENTED_EDGE('',*,*,#56153,.F.);
#82564=ORIENTED_EDGE('',*,*,#56154,.F.);
#82565=ORIENTED_EDGE('',*,*,#56155,.F.);
#82566=ORIENTED_EDGE('',*,*,#56156,.F.);
#82567=ORIENTED_EDGE('',*,*,#56157,.F.);
#82568=ORIENTED_EDGE('',*,*,#56082,.T.);
#82569=ORIENTED_EDGE('',*,*,#56158,.F.);
#82570=ORIENTED_EDGE('',*,*,#56159,.F.);
#82571=ORIENTED_EDGE('',*,*,#56080,.T.);
#82572=ORIENTED_EDGE('',*,*,#56160,.F.);
#82573=ORIENTED_EDGE('',*,*,#56161,.F.);
#82574=ORIENTED_EDGE('',*,*,#56162,.F.);
#82575=ORIENTED_EDGE('',*,*,#56163,.F.);
#82576=ORIENTED_EDGE('',*,*,#56164,.F.);
#82577=ORIENTED_EDGE('',*,*,#56078,.T.);
#82578=ORIENTED_EDGE('',*,*,#56165,.F.);
#82579=ORIENTED_EDGE('',*,*,#55949,.F.);
#82580=ORIENTED_EDGE('',*,*,#56166,.F.);
#82581=ORIENTED_EDGE('',*,*,#56167,.F.);
#82582=ORIENTED_EDGE('',*,*,#56168,.F.);
#82583=ORIENTED_EDGE('',*,*,#56169,.F.);
#82584=ORIENTED_EDGE('',*,*,#56170,.F.);
#82585=ORIENTED_EDGE('',*,*,#56171,.F.);
#82586=ORIENTED_EDGE('',*,*,#56076,.T.);
#82587=ORIENTED_EDGE('',*,*,#56172,.F.);
#82588=ORIENTED_EDGE('',*,*,#56173,.F.);
#82589=ORIENTED_EDGE('',*,*,#56074,.T.);
#82590=ORIENTED_EDGE('',*,*,#56174,.F.);
#82591=ORIENTED_EDGE('',*,*,#56175,.F.);
#82592=ORIENTED_EDGE('',*,*,#56176,.F.);
#82593=ORIENTED_EDGE('',*,*,#56177,.F.);
#82594=ORIENTED_EDGE('',*,*,#56178,.F.);
#82595=ORIENTED_EDGE('',*,*,#56179,.F.);
#82596=ORIENTED_EDGE('',*,*,#56180,.F.);
#82597=ORIENTED_EDGE('',*,*,#56181,.F.);
#82598=ORIENTED_EDGE('',*,*,#56072,.T.);
#82599=ORIENTED_EDGE('',*,*,#56182,.F.);
#82600=ORIENTED_EDGE('',*,*,#56183,.F.);
#82601=ORIENTED_EDGE('',*,*,#56070,.T.);
#82602=ORIENTED_EDGE('',*,*,#56184,.F.);
#82603=ORIENTED_EDGE('',*,*,#56185,.F.);
#82604=ORIENTED_EDGE('',*,*,#56186,.F.);
#82605=ORIENTED_EDGE('',*,*,#56187,.F.);
#82606=ORIENTED_EDGE('',*,*,#56188,.F.);
#82607=ORIENTED_EDGE('',*,*,#56189,.F.);
#82608=ORIENTED_EDGE('',*,*,#56190,.F.);
#82609=ORIENTED_EDGE('',*,*,#56042,.F.);
#82610=ORIENTED_EDGE('',*,*,#56090,.T.);
#82611=ORIENTED_EDGE('',*,*,#55960,.F.);
#82612=ORIENTED_EDGE('',*,*,#55954,.F.);
#82613=ORIENTED_EDGE('',*,*,#56089,.T.);
#82614=ORIENTED_EDGE('',*,*,#55968,.F.);
#82615=ORIENTED_EDGE('',*,*,#56191,.F.);
#82616=ORIENTED_EDGE('',*,*,#56192,.F.);
#82617=ORIENTED_EDGE('',*,*,#56193,.F.);
#82618=ORIENTED_EDGE('',*,*,#55962,.F.);
#82619=ORIENTED_EDGE('',*,*,#56088,.T.);
#82620=ORIENTED_EDGE('',*,*,#55984,.F.);
#82621=ORIENTED_EDGE('',*,*,#56194,.F.);
#82622=ORIENTED_EDGE('',*,*,#56195,.F.);
#82623=ORIENTED_EDGE('',*,*,#56196,.F.);
#82624=ORIENTED_EDGE('',*,*,#56197,.F.);
#82625=ORIENTED_EDGE('',*,*,#56198,.F.);
#82626=ORIENTED_EDGE('',*,*,#56199,.F.);
#82627=ORIENTED_EDGE('',*,*,#55978,.F.);
#82628=ORIENTED_EDGE('',*,*,#56087,.T.);
#82629=ORIENTED_EDGE('',*,*,#55976,.F.);
#82630=ORIENTED_EDGE('',*,*,#55970,.F.);
#82631=ORIENTED_EDGE('',*,*,#56086,.T.);
#82632=ORIENTED_EDGE('',*,*,#55999,.F.);
#82633=ORIENTED_EDGE('',*,*,#56200,.F.);
#82634=ORIENTED_EDGE('',*,*,#56201,.F.);
#82635=ORIENTED_EDGE('',*,*,#56202,.F.);
#82636=ORIENTED_EDGE('',*,*,#56203,.F.);
#82637=ORIENTED_EDGE('',*,*,#56204,.F.);
#82638=ORIENTED_EDGE('',*,*,#56205,.F.);
#82639=ORIENTED_EDGE('',*,*,#55993,.F.);
#82640=ORIENTED_EDGE('',*,*,#56085,.T.);
#82641=ORIENTED_EDGE('',*,*,#55991,.F.);
#82642=ORIENTED_EDGE('',*,*,#55985,.F.);
#82643=ORIENTED_EDGE('',*,*,#56084,.T.);
#82644=ORIENTED_EDGE('',*,*,#56206,.F.);
#82645=ORIENTED_EDGE('',*,*,#56207,.F.);
#82646=ORIENTED_EDGE('',*,*,#56208,.F.);
#82647=ORIENTED_EDGE('',*,*,#56209,.F.);
#82648=ORIENTED_EDGE('',*,*,#56210,.F.);
#82649=ORIENTED_EDGE('',*,*,#56211,.F.);
#82650=ORIENTED_EDGE('',*,*,#56212,.F.);
#82651=ORIENTED_EDGE('',*,*,#56019,.F.);
#82652=ORIENTED_EDGE('',*,*,#56095,.T.);
#82653=ORIENTED_EDGE('',*,*,#56001,.F.);
#82654=ORIENTED_EDGE('',*,*,#56003,.F.);
#82655=ORIENTED_EDGE('',*,*,#56094,.T.);
#82656=ORIENTED_EDGE('',*,*,#56016,.F.);
#82657=ORIENTED_EDGE('',*,*,#56213,.F.);
#82658=ORIENTED_EDGE('',*,*,#56214,.F.);
#82659=ORIENTED_EDGE('',*,*,#56215,.F.);
#82660=ORIENTED_EDGE('',*,*,#56010,.F.);
#82661=ORIENTED_EDGE('',*,*,#56093,.T.);
#82662=ORIENTED_EDGE('',*,*,#56032,.F.);
#82663=ORIENTED_EDGE('',*,*,#56216,.F.);
#82664=ORIENTED_EDGE('',*,*,#56217,.F.);
#82665=ORIENTED_EDGE('',*,*,#56218,.F.);
#82666=ORIENTED_EDGE('',*,*,#56219,.F.);
#82667=ORIENTED_EDGE('',*,*,#56220,.F.);
#82668=ORIENTED_EDGE('',*,*,#56221,.F.);
#82669=ORIENTED_EDGE('',*,*,#56222,.F.);
#82670=ORIENTED_EDGE('',*,*,#56096,.T.);
#82671=ORIENTED_EDGE('',*,*,#56017,.F.);
#82672=ORIENTED_EDGE('',*,*,#56223,.F.);
#82673=ORIENTED_EDGE('',*,*,#56224,.F.);
#82674=ORIENTED_EDGE('',*,*,#56225,.F.);
#82675=ORIENTED_EDGE('',*,*,#56226,.F.);
#82676=ORIENTED_EDGE('',*,*,#56098,.T.);
#82677=ORIENTED_EDGE('',*,*,#56227,.F.);
#82678=ORIENTED_EDGE('',*,*,#56026,.F.);
#82679=ORIENTED_EDGE('',*,*,#56092,.T.);
#82680=ORIENTED_EDGE('',*,*,#56040,.F.);
#82681=ORIENTED_EDGE('',*,*,#56228,.F.);
#82682=ORIENTED_EDGE('',*,*,#56229,.F.);
#82683=ORIENTED_EDGE('',*,*,#56230,.F.);
#82684=ORIENTED_EDGE('',*,*,#56034,.F.);
#82685=ORIENTED_EDGE('',*,*,#56091,.T.);
#82686=ORIENTED_EDGE('',*,*,#56048,.F.);
#82687=ORIENTED_EDGE('',*,*,#56231,.F.);
#82688=ORIENTED_EDGE('',*,*,#56232,.F.);
#82689=ORIENTED_EDGE('',*,*,#56233,.F.);
#82690=ORIENTED_EDGE('',*,*,#56234,.F.);
#82691=ORIENTED_EDGE('',*,*,#56235,.F.);
#82692=ORIENTED_EDGE('',*,*,#56236,.F.);
#82693=ORIENTED_EDGE('',*,*,#56121,.T.);
#82694=ORIENTED_EDGE('',*,*,#56237,.F.);
#82695=ORIENTED_EDGE('',*,*,#56128,.T.);
#82696=ORIENTED_EDGE('',*,*,#56238,.F.);
#82697=ORIENTED_EDGE('',*,*,#56239,.F.);
#82698=ORIENTED_EDGE('',*,*,#56240,.F.);
#82699=ORIENTED_EDGE('',*,*,#56133,.T.);
#82700=ORIENTED_EDGE('',*,*,#56241,.F.);
#82701=ORIENTED_EDGE('',*,*,#56242,.F.);
#82702=ORIENTED_EDGE('',*,*,#56243,.F.);
#82703=ORIENTED_EDGE('',*,*,#56138,.T.);
#82704=ORIENTED_EDGE('',*,*,#56244,.F.);
#82705=ORIENTED_EDGE('',*,*,#56245,.F.);
#82706=ORIENTED_EDGE('',*,*,#56246,.F.);
#82707=ORIENTED_EDGE('',*,*,#56247,.F.);
#82708=ORIENTED_EDGE('',*,*,#56248,.F.);
#82709=ORIENTED_EDGE('',*,*,#56141,.T.);
#82710=ORIENTED_EDGE('',*,*,#55946,.F.);
#82711=ORIENTED_EDGE('',*,*,#56148,.T.);
#82712=ORIENTED_EDGE('',*,*,#56249,.F.);
#82713=ORIENTED_EDGE('',*,*,#56250,.F.);
#82714=ORIENTED_EDGE('',*,*,#56251,.F.);
#82715=ORIENTED_EDGE('',*,*,#56152,.T.);
#82716=ORIENTED_EDGE('',*,*,#56252,.F.);
#82717=ORIENTED_EDGE('',*,*,#56253,.F.);
#82718=ORIENTED_EDGE('',*,*,#56254,.F.);
#82719=ORIENTED_EDGE('',*,*,#56255,.F.);
#82720=ORIENTED_EDGE('',*,*,#56256,.F.);
#82721=ORIENTED_EDGE('',*,*,#56155,.T.);
#82722=ORIENTED_EDGE('',*,*,#56257,.F.);
#82723=ORIENTED_EDGE('',*,*,#56162,.T.);
#82724=ORIENTED_EDGE('',*,*,#56258,.F.);
#82725=ORIENTED_EDGE('',*,*,#56259,.F.);
#82726=ORIENTED_EDGE('',*,*,#56260,.F.);
#82727=ORIENTED_EDGE('',*,*,#56166,.T.);
#82728=ORIENTED_EDGE('',*,*,#55952,.F.);
#82729=ORIENTED_EDGE('',*,*,#56261,.F.);
#82730=ORIENTED_EDGE('',*,*,#56262,.F.);
#82731=ORIENTED_EDGE('',*,*,#56263,.F.);
#82732=ORIENTED_EDGE('',*,*,#56264,.F.);
#82733=ORIENTED_EDGE('',*,*,#56169,.T.);
#82734=ORIENTED_EDGE('',*,*,#56265,.F.);
#82735=ORIENTED_EDGE('',*,*,#56176,.T.);
#82736=ORIENTED_EDGE('',*,*,#56266,.F.);
#82737=ORIENTED_EDGE('',*,*,#56267,.F.);
#82738=ORIENTED_EDGE('',*,*,#56268,.F.);
#82739=ORIENTED_EDGE('',*,*,#56269,.F.);
#82740=ORIENTED_EDGE('',*,*,#56270,.F.);
#82741=ORIENTED_EDGE('',*,*,#56179,.T.);
#82742=ORIENTED_EDGE('',*,*,#56271,.F.);
#82743=ORIENTED_EDGE('',*,*,#56186,.T.);
#82744=ORIENTED_EDGE('',*,*,#56272,.F.);
#82745=ORIENTED_EDGE('',*,*,#56273,.F.);
#82746=ORIENTED_EDGE('',*,*,#56274,.F.);
#82747=ORIENTED_EDGE('',*,*,#56275,.F.);
#82748=ORIENTED_EDGE('',*,*,#56276,.F.);
#82749=ORIENTED_EDGE('',*,*,#56189,.T.);
#82750=ORIENTED_EDGE('',*,*,#56277,.F.);
#82751=ORIENTED_EDGE('',*,*,#56192,.T.);
#82752=ORIENTED_EDGE('',*,*,#56278,.F.);
#82753=ORIENTED_EDGE('',*,*,#56279,.F.);
#82754=ORIENTED_EDGE('',*,*,#56280,.F.);
#82755=ORIENTED_EDGE('',*,*,#56195,.T.);
#82756=ORIENTED_EDGE('',*,*,#56281,.F.);
#82757=ORIENTED_EDGE('',*,*,#56282,.F.);
#82758=ORIENTED_EDGE('',*,*,#56283,.F.);
#82759=ORIENTED_EDGE('',*,*,#56284,.F.);
#82760=ORIENTED_EDGE('',*,*,#56285,.F.);
#82761=ORIENTED_EDGE('',*,*,#56198,.T.);
#82762=ORIENTED_EDGE('',*,*,#56286,.F.);
#82763=ORIENTED_EDGE('',*,*,#56201,.T.);
#82764=ORIENTED_EDGE('',*,*,#56287,.F.);
#82765=ORIENTED_EDGE('',*,*,#56288,.F.);
#82766=ORIENTED_EDGE('',*,*,#56289,.F.);
#82767=ORIENTED_EDGE('',*,*,#56290,.F.);
#82768=ORIENTED_EDGE('',*,*,#56291,.F.);
#82769=ORIENTED_EDGE('',*,*,#56204,.T.);
#82770=ORIENTED_EDGE('',*,*,#56292,.F.);
#82771=ORIENTED_EDGE('',*,*,#56208,.T.);
#82772=ORIENTED_EDGE('',*,*,#56293,.F.);
#82773=ORIENTED_EDGE('',*,*,#56294,.F.);
#82774=ORIENTED_EDGE('',*,*,#56295,.F.);
#82775=ORIENTED_EDGE('',*,*,#56296,.F.);
#82776=ORIENTED_EDGE('',*,*,#56297,.F.);
#82777=ORIENTED_EDGE('',*,*,#56211,.T.);
#82778=ORIENTED_EDGE('',*,*,#56298,.F.);
#82779=ORIENTED_EDGE('',*,*,#56214,.T.);
#82780=ORIENTED_EDGE('',*,*,#56299,.F.);
#82781=ORIENTED_EDGE('',*,*,#56300,.F.);
#82782=ORIENTED_EDGE('',*,*,#56301,.F.);
#82783=ORIENTED_EDGE('',*,*,#56217,.T.);
#82784=ORIENTED_EDGE('',*,*,#56302,.F.);
#82785=ORIENTED_EDGE('',*,*,#56303,.F.);
#82786=ORIENTED_EDGE('',*,*,#56304,.F.);
#82787=ORIENTED_EDGE('',*,*,#56305,.F.);
#82788=ORIENTED_EDGE('',*,*,#56306,.F.);
#82789=ORIENTED_EDGE('',*,*,#56220,.T.);
#82790=ORIENTED_EDGE('',*,*,#56307,.F.);
#82791=ORIENTED_EDGE('',*,*,#56308,.F.);
#82792=ORIENTED_EDGE('',*,*,#56309,.F.);
#82793=ORIENTED_EDGE('',*,*,#56224,.T.);
#82794=ORIENTED_EDGE('',*,*,#56310,.F.);
#82795=ORIENTED_EDGE('',*,*,#56229,.T.);
#82796=ORIENTED_EDGE('',*,*,#56311,.F.);
#82797=ORIENTED_EDGE('',*,*,#56312,.F.);
#82798=ORIENTED_EDGE('',*,*,#56313,.F.);
#82799=ORIENTED_EDGE('',*,*,#56232,.T.);
#82800=ORIENTED_EDGE('',*,*,#56314,.F.);
#82801=ORIENTED_EDGE('',*,*,#56315,.F.);
#82802=ORIENTED_EDGE('',*,*,#56316,.F.);
#82803=ORIENTED_EDGE('',*,*,#56317,.F.);
#82804=ORIENTED_EDGE('',*,*,#56318,.F.);
#82805=ORIENTED_EDGE('',*,*,#56319,.F.);
#82806=ORIENTED_EDGE('',*,*,#56320,.F.);
#82807=ORIENTED_EDGE('',*,*,#56235,.T.);
#82808=ORIENTED_EDGE('',*,*,#56321,.F.);
#82809=ORIENTED_EDGE('',*,*,#56322,.F.);
#82810=ORIENTED_EDGE('',*,*,#56239,.T.);
#82811=ORIENTED_EDGE('',*,*,#56323,.F.);
#82812=ORIENTED_EDGE('',*,*,#56324,.F.);
#82813=ORIENTED_EDGE('',*,*,#56325,.F.);
#82814=ORIENTED_EDGE('',*,*,#56326,.F.);
#82815=ORIENTED_EDGE('',*,*,#56327,.F.);
#82816=ORIENTED_EDGE('',*,*,#56242,.T.);
#82817=ORIENTED_EDGE('',*,*,#56328,.F.);
#82818=ORIENTED_EDGE('',*,*,#56329,.F.);
#82819=ORIENTED_EDGE('',*,*,#56330,.F.);
#82820=ORIENTED_EDGE('',*,*,#56331,.F.);
#82821=ORIENTED_EDGE('',*,*,#56332,.F.);
#82822=ORIENTED_EDGE('',*,*,#56245,.T.);
#82823=ORIENTED_EDGE('',*,*,#56333,.F.);
#82824=ORIENTED_EDGE('',*,*,#56334,.F.);
#82825=ORIENTED_EDGE('',*,*,#56335,.F.);
#82826=ORIENTED_EDGE('',*,*,#56336,.F.);
#82827=ORIENTED_EDGE('',*,*,#56337,.F.);
#82828=ORIENTED_EDGE('',*,*,#56338,.F.);
#82829=ORIENTED_EDGE('',*,*,#56339,.F.);
#82830=ORIENTED_EDGE('',*,*,#56340,.F.);
#82831=ORIENTED_EDGE('',*,*,#56247,.T.);
#82832=ORIENTED_EDGE('',*,*,#56341,.F.);
#82833=ORIENTED_EDGE('',*,*,#55947,.F.);
#82834=ORIENTED_EDGE('',*,*,#56250,.T.);
#82835=ORIENTED_EDGE('',*,*,#56342,.F.);
#82836=ORIENTED_EDGE('',*,*,#56343,.F.);
#82837=ORIENTED_EDGE('',*,*,#56344,.F.);
#82838=ORIENTED_EDGE('',*,*,#56345,.F.);
#82839=ORIENTED_EDGE('',*,*,#56346,.F.);
#82840=ORIENTED_EDGE('',*,*,#56253,.T.);
#82841=ORIENTED_EDGE('',*,*,#56347,.F.);
#82842=ORIENTED_EDGE('',*,*,#56348,.F.);
#82843=ORIENTED_EDGE('',*,*,#56349,.F.);
#82844=ORIENTED_EDGE('',*,*,#56350,.F.);
#82845=ORIENTED_EDGE('',*,*,#56351,.F.);
#82846=ORIENTED_EDGE('',*,*,#56352,.F.);
#82847=ORIENTED_EDGE('',*,*,#56353,.F.);
#82848=ORIENTED_EDGE('',*,*,#56354,.F.);
#82849=ORIENTED_EDGE('',*,*,#56255,.T.);
#82850=ORIENTED_EDGE('',*,*,#56355,.F.);
#82851=ORIENTED_EDGE('',*,*,#56356,.F.);
#82852=ORIENTED_EDGE('',*,*,#56259,.T.);
#82853=ORIENTED_EDGE('',*,*,#56357,.F.);
#82854=ORIENTED_EDGE('',*,*,#56358,.F.);
#82855=ORIENTED_EDGE('',*,*,#56359,.F.);
#82856=ORIENTED_EDGE('',*,*,#56360,.F.);
#82857=ORIENTED_EDGE('',*,*,#56361,.F.);
#82858=ORIENTED_EDGE('',*,*,#56261,.T.);
#82859=ORIENTED_EDGE('',*,*,#55951,.F.);
#82860=ORIENTED_EDGE('',*,*,#56362,.F.);
#82861=ORIENTED_EDGE('',*,*,#56363,.F.);
#82862=ORIENTED_EDGE('',*,*,#56364,.F.);
#82863=ORIENTED_EDGE('',*,*,#56365,.F.);
#82864=ORIENTED_EDGE('',*,*,#56366,.F.);
#82865=ORIENTED_EDGE('',*,*,#56367,.F.);
#82866=ORIENTED_EDGE('',*,*,#56368,.F.);
#82867=ORIENTED_EDGE('',*,*,#56263,.T.);
#82868=ORIENTED_EDGE('',*,*,#56369,.F.);
#82869=ORIENTED_EDGE('',*,*,#56370,.F.);
#82870=ORIENTED_EDGE('',*,*,#56267,.T.);
#82871=ORIENTED_EDGE('',*,*,#56371,.F.);
#82872=ORIENTED_EDGE('',*,*,#56372,.F.);
#82873=ORIENTED_EDGE('',*,*,#56373,.F.);
#82874=ORIENTED_EDGE('',*,*,#56374,.F.);
#82875=ORIENTED_EDGE('',*,*,#56375,.F.);
#82876=ORIENTED_EDGE('',*,*,#56376,.F.);
#82877=ORIENTED_EDGE('',*,*,#56377,.F.);
#82878=ORIENTED_EDGE('',*,*,#56378,.F.);
#82879=ORIENTED_EDGE('',*,*,#56269,.T.);
#82880=ORIENTED_EDGE('',*,*,#56379,.F.);
#82881=ORIENTED_EDGE('',*,*,#56380,.F.);
#82882=ORIENTED_EDGE('',*,*,#56273,.T.);
#82883=ORIENTED_EDGE('',*,*,#56381,.F.);
#82884=ORIENTED_EDGE('',*,*,#56382,.F.);
#82885=ORIENTED_EDGE('',*,*,#56383,.F.);
#82886=ORIENTED_EDGE('',*,*,#56384,.F.);
#82887=ORIENTED_EDGE('',*,*,#55958,.F.);
#82888=ORIENTED_EDGE('',*,*,#56385,.F.);
#82889=ORIENTED_EDGE('',*,*,#56044,.F.);
#82890=ORIENTED_EDGE('',*,*,#56386,.F.);
#82891=ORIENTED_EDGE('',*,*,#56275,.T.);
#82892=ORIENTED_EDGE('',*,*,#55956,.F.);
#82893=ORIENTED_EDGE('',*,*,#56387,.F.);
#82894=ORIENTED_EDGE('',*,*,#56279,.T.);
#82895=ORIENTED_EDGE('',*,*,#56388,.F.);
#82896=ORIENTED_EDGE('',*,*,#55966,.F.);
#82897=ORIENTED_EDGE('',*,*,#56389,.F.);
#82898=ORIENTED_EDGE('',*,*,#55964,.F.);
#82899=ORIENTED_EDGE('',*,*,#56390,.F.);
#82900=ORIENTED_EDGE('',*,*,#56282,.T.);
#82901=ORIENTED_EDGE('',*,*,#56391,.F.);
#82902=ORIENTED_EDGE('',*,*,#55982,.F.);
#82903=ORIENTED_EDGE('',*,*,#56392,.F.);
#82904=ORIENTED_EDGE('',*,*,#56393,.F.);
#82905=ORIENTED_EDGE('',*,*,#55974,.F.);
#82906=ORIENTED_EDGE('',*,*,#56394,.F.);
#82907=ORIENTED_EDGE('',*,*,#55980,.F.);
#82908=ORIENTED_EDGE('',*,*,#56395,.F.);
#82909=ORIENTED_EDGE('',*,*,#56284,.T.);
#82910=ORIENTED_EDGE('',*,*,#55972,.F.);
#82911=ORIENTED_EDGE('',*,*,#56396,.F.);
#82912=ORIENTED_EDGE('',*,*,#56288,.T.);
#82913=ORIENTED_EDGE('',*,*,#56397,.F.);
#82914=ORIENTED_EDGE('',*,*,#55997,.F.);
#82915=ORIENTED_EDGE('',*,*,#56398,.F.);
#82916=ORIENTED_EDGE('',*,*,#56399,.F.);
#82917=ORIENTED_EDGE('',*,*,#55989,.F.);
#82918=ORIENTED_EDGE('',*,*,#56400,.F.);
#82919=ORIENTED_EDGE('',*,*,#55995,.F.);
#82920=ORIENTED_EDGE('',*,*,#56401,.F.);
#82921=ORIENTED_EDGE('',*,*,#56290,.T.);
#82922=ORIENTED_EDGE('',*,*,#55987,.F.);
#82923=ORIENTED_EDGE('',*,*,#56402,.F.);
#82924=ORIENTED_EDGE('',*,*,#56294,.T.);
#82925=ORIENTED_EDGE('',*,*,#56403,.F.);
#82926=ORIENTED_EDGE('',*,*,#56404,.F.);
#82927=ORIENTED_EDGE('',*,*,#56405,.F.);
#82928=ORIENTED_EDGE('',*,*,#56406,.F.);
#82929=ORIENTED_EDGE('',*,*,#56007,.F.);
#82930=ORIENTED_EDGE('',*,*,#56407,.F.);
#82931=ORIENTED_EDGE('',*,*,#56021,.F.);
#82932=ORIENTED_EDGE('',*,*,#56408,.F.);
#82933=ORIENTED_EDGE('',*,*,#56296,.T.);
#82934=ORIENTED_EDGE('',*,*,#56005,.F.);
#82935=ORIENTED_EDGE('',*,*,#56409,.F.);
#82936=ORIENTED_EDGE('',*,*,#56300,.T.);
#82937=ORIENTED_EDGE('',*,*,#56410,.F.);
#82938=ORIENTED_EDGE('',*,*,#56014,.F.);
#82939=ORIENTED_EDGE('',*,*,#56411,.F.);
#82940=ORIENTED_EDGE('',*,*,#56012,.F.);
#82941=ORIENTED_EDGE('',*,*,#56412,.F.);
#82942=ORIENTED_EDGE('',*,*,#56303,.T.);
#82943=ORIENTED_EDGE('',*,*,#56413,.F.);
#82944=ORIENTED_EDGE('',*,*,#56030,.F.);
#82945=ORIENTED_EDGE('',*,*,#56414,.F.);
#82946=ORIENTED_EDGE('',*,*,#56415,.F.);
#82947=ORIENTED_EDGE('',*,*,#56023,.F.);
#82948=ORIENTED_EDGE('',*,*,#56416,.F.);
#82949=ORIENTED_EDGE('',*,*,#56417,.F.);
#82950=ORIENTED_EDGE('',*,*,#56418,.F.);
#82951=ORIENTED_EDGE('',*,*,#56305,.T.);
#82952=ORIENTED_EDGE('',*,*,#56419,.F.);
#82953=ORIENTED_EDGE('',*,*,#56420,.F.);
#82954=ORIENTED_EDGE('',*,*,#56421,.F.);
#82955=ORIENTED_EDGE('',*,*,#56422,.F.);
#82956=ORIENTED_EDGE('',*,*,#56423,.F.);
#82957=ORIENTED_EDGE('',*,*,#56308,.T.);
#82958=ORIENTED_EDGE('',*,*,#56028,.F.);
#82959=ORIENTED_EDGE('',*,*,#56424,.F.);
#82960=ORIENTED_EDGE('',*,*,#56312,.T.);
#82961=ORIENTED_EDGE('',*,*,#56425,.F.);
#82962=ORIENTED_EDGE('',*,*,#56038,.F.);
#82963=ORIENTED_EDGE('',*,*,#56426,.F.);
#82964=ORIENTED_EDGE('',*,*,#56036,.F.);
#82965=ORIENTED_EDGE('',*,*,#56427,.F.);
#82966=ORIENTED_EDGE('',*,*,#56315,.T.);
#82967=ORIENTED_EDGE('',*,*,#56428,.F.);
#82968=ORIENTED_EDGE('',*,*,#56046,.F.);
#82969=ORIENTED_EDGE('',*,*,#56429,.F.);
#82970=ORIENTED_EDGE('',*,*,#56430,.F.);
#82971=ORIENTED_EDGE('',*,*,#56100,.T.);
#82972=ORIENTED_EDGE('',*,*,#56431,.F.);
#82973=ORIENTED_EDGE('',*,*,#56432,.F.);
#82974=ORIENTED_EDGE('',*,*,#56433,.F.);
#82975=ORIENTED_EDGE('',*,*,#56434,.F.);
#82976=ORIENTED_EDGE('',*,*,#56435,.F.);
#82977=ORIENTED_EDGE('',*,*,#56433,.T.);
#82978=ORIENTED_EDGE('',*,*,#56436,.F.);
#82979=ORIENTED_EDGE('',*,*,#56437,.F.);
#82980=ORIENTED_EDGE('',*,*,#56438,.F.);
#82981=ORIENTED_EDGE('',*,*,#56439,.F.);
#82982=ORIENTED_EDGE('',*,*,#56437,.T.);
#82983=ORIENTED_EDGE('',*,*,#56440,.F.);
#82984=ORIENTED_EDGE('',*,*,#56441,.F.);
#82985=ORIENTED_EDGE('',*,*,#56442,.F.);
#82986=ORIENTED_EDGE('',*,*,#56443,.F.);
#82987=ORIENTED_EDGE('',*,*,#56052,.T.);
#82988=ORIENTED_EDGE('',*,*,#56444,.F.);
#82989=ORIENTED_EDGE('',*,*,#56325,.T.);
#82990=ORIENTED_EDGE('',*,*,#56445,.F.);
#82991=ORIENTED_EDGE('',*,*,#56330,.T.);
#82992=ORIENTED_EDGE('',*,*,#56446,.F.);
#82993=ORIENTED_EDGE('',*,*,#56335,.T.);
#82994=ORIENTED_EDGE('',*,*,#56447,.F.);
#82995=ORIENTED_EDGE('',*,*,#56349,.T.);
#82996=ORIENTED_EDGE('',*,*,#56448,.F.);
#82997=ORIENTED_EDGE('',*,*,#56338,.T.);
#82998=ORIENTED_EDGE('',*,*,#56449,.F.);
#82999=ORIENTED_EDGE('',*,*,#56344,.T.);
#83000=ORIENTED_EDGE('',*,*,#56450,.F.);
#83001=ORIENTED_EDGE('',*,*,#56442,.T.);
#83002=ORIENTED_EDGE('',*,*,#56451,.F.);
#83003=ORIENTED_EDGE('',*,*,#56421,.T.);
#83004=ORIENTED_EDGE('',*,*,#56452,.F.);
#83005=ORIENTED_EDGE('',*,*,#56416,.T.);
#83006=ORIENTED_EDGE('',*,*,#56022,.F.);
#83007=ORIENTED_EDGE('',*,*,#56407,.T.);
#83008=ORIENTED_EDGE('',*,*,#56006,.F.);
#83009=ORIENTED_EDGE('',*,*,#56411,.T.);
#83010=ORIENTED_EDGE('',*,*,#56013,.F.);
#83011=ORIENTED_EDGE('',*,*,#56414,.T.);
#83012=ORIENTED_EDGE('',*,*,#56029,.F.);
#83013=ORIENTED_EDGE('',*,*,#56426,.T.);
#83014=ORIENTED_EDGE('',*,*,#56037,.F.);
#83015=ORIENTED_EDGE('',*,*,#56429,.T.);
#83016=ORIENTED_EDGE('',*,*,#56045,.F.);
#83017=ORIENTED_EDGE('',*,*,#56385,.T.);
#83018=ORIENTED_EDGE('',*,*,#55957,.F.);
#83019=ORIENTED_EDGE('',*,*,#56389,.T.);
#83020=ORIENTED_EDGE('',*,*,#55965,.F.);
#83021=ORIENTED_EDGE('',*,*,#56392,.T.);
#83022=ORIENTED_EDGE('',*,*,#55981,.F.);
#83023=ORIENTED_EDGE('',*,*,#56394,.T.);
#83024=ORIENTED_EDGE('',*,*,#55973,.F.);
#83025=ORIENTED_EDGE('',*,*,#56398,.T.);
#83026=ORIENTED_EDGE('',*,*,#55996,.F.);
#83027=ORIENTED_EDGE('',*,*,#56400,.T.);
#83028=ORIENTED_EDGE('',*,*,#55988,.F.);
#83029=ORIENTED_EDGE('',*,*,#56405,.T.);
#83030=ORIENTED_EDGE('',*,*,#56453,.F.);
#83031=ORIENTED_EDGE('',*,*,#56352,.T.);
#83032=ORIENTED_EDGE('',*,*,#56454,.F.);
#83033=ORIENTED_EDGE('',*,*,#56359,.T.);
#83034=ORIENTED_EDGE('',*,*,#56455,.F.);
#83035=ORIENTED_EDGE('',*,*,#56363,.T.);
#83036=ORIENTED_EDGE('',*,*,#56456,.F.);
#83037=ORIENTED_EDGE('',*,*,#56366,.T.);
#83038=ORIENTED_EDGE('',*,*,#56457,.F.);
#83039=ORIENTED_EDGE('',*,*,#56373,.T.);
#83040=ORIENTED_EDGE('',*,*,#56458,.F.);
#83041=ORIENTED_EDGE('',*,*,#56376,.T.);
#83042=ORIENTED_EDGE('',*,*,#56459,.F.);
#83043=ORIENTED_EDGE('',*,*,#56383,.T.);
#83044=ORIENTED_EDGE('',*,*,#56460,.F.);
#83045=ORIENTED_EDGE('',*,*,#56318,.T.);
#83046=ORIENTED_EDGE('',*,*,#55940,.T.);
#83047=ORIENTED_EDGE('',*,*,#56432,.T.);
#83048=ORIENTED_EDGE('',*,*,#56461,.T.);
#83049=ORIENTED_EDGE('',*,*,#56440,.T.);
#83050=ORIENTED_EDGE('',*,*,#56436,.T.);
#83051=ORIENTED_EDGE('',*,*,#56225,.T.);
#83052=ORIENTED_EDGE('',*,*,#56309,.T.);
#83053=ORIENTED_EDGE('',*,*,#56423,.T.);
#83054=ORIENTED_EDGE('',*,*,#56462,.F.);
#83055=ORIENTED_EDGE('',*,*,#56431,.T.);
#83056=ORIENTED_EDGE('',*,*,#56099,.T.);
#83057=ORIENTED_EDGE('',*,*,#56226,.T.);
#83058=ORIENTED_EDGE('',*,*,#56462,.T.);
#83059=ORIENTED_EDGE('',*,*,#56422,.T.);
#83060=ORIENTED_EDGE('',*,*,#56451,.T.);
#83061=ORIENTED_EDGE('',*,*,#56441,.T.);
#83062=ORIENTED_EDGE('',*,*,#56461,.F.);
#83063=ORIENTED_EDGE('',*,*,#56147,.T.);
#83064=ORIENTED_EDGE('',*,*,#56463,.T.);
#83065=ORIENTED_EDGE('',*,*,#56342,.T.);
#83066=ORIENTED_EDGE('',*,*,#56249,.T.);
#83067=ORIENTED_EDGE('',*,*,#56434,.T.);
#83068=ORIENTED_EDGE('',*,*,#56435,.T.);
#83069=ORIENTED_EDGE('',*,*,#56439,.T.);
#83070=ORIENTED_EDGE('',*,*,#56464,.F.);
#83071=ORIENTED_EDGE('',*,*,#56146,.T.);
#83072=ORIENTED_EDGE('',*,*,#56101,.T.);
#83073=ORIENTED_EDGE('',*,*,#56430,.T.);
#83074=ORIENTED_EDGE('',*,*,#56464,.T.);
#83075=ORIENTED_EDGE('',*,*,#56438,.T.);
#83076=ORIENTED_EDGE('',*,*,#56450,.T.);
#83077=ORIENTED_EDGE('',*,*,#56343,.T.);
#83078=ORIENTED_EDGE('',*,*,#56463,.F.);
#83079=ORIENTED_EDGE('',*,*,#56231,.T.);
#83080=ORIENTED_EDGE('',*,*,#56047,.T.);
#83081=ORIENTED_EDGE('',*,*,#56428,.T.);
#83082=ORIENTED_EDGE('',*,*,#56314,.T.);
#83083=ORIENTED_EDGE('',*,*,#56190,.T.);
#83084=ORIENTED_EDGE('',*,*,#56276,.T.);
#83085=ORIENTED_EDGE('',*,*,#56386,.T.);
#83086=ORIENTED_EDGE('',*,*,#56043,.F.);
#83087=ORIENTED_EDGE('',*,*,#56228,.T.);
#83088=ORIENTED_EDGE('',*,*,#56039,.T.);
#83089=ORIENTED_EDGE('',*,*,#56425,.T.);
#83090=ORIENTED_EDGE('',*,*,#56311,.T.);
#83091=ORIENTED_EDGE('',*,*,#56233,.T.);
#83092=ORIENTED_EDGE('',*,*,#56313,.T.);
#83093=ORIENTED_EDGE('',*,*,#56427,.T.);
#83094=ORIENTED_EDGE('',*,*,#56035,.F.);
#83095=ORIENTED_EDGE('',*,*,#56216,.T.);
#83096=ORIENTED_EDGE('',*,*,#56031,.T.);
#83097=ORIENTED_EDGE('',*,*,#56413,.T.);
#83098=ORIENTED_EDGE('',*,*,#56302,.T.);
#83099=ORIENTED_EDGE('',*,*,#56230,.T.);
#83100=ORIENTED_EDGE('',*,*,#56310,.T.);
#83101=ORIENTED_EDGE('',*,*,#56424,.T.);
#83102=ORIENTED_EDGE('',*,*,#56027,.F.);
#83103=ORIENTED_EDGE('',*,*,#56223,.T.);
#83104=ORIENTED_EDGE('',*,*,#56465,.T.);
#83105=ORIENTED_EDGE('',*,*,#56419,.T.);
#83106=ORIENTED_EDGE('',*,*,#56307,.T.);
#83107=ORIENTED_EDGE('',*,*,#56221,.T.);
#83108=ORIENTED_EDGE('',*,*,#56306,.T.);
#83109=ORIENTED_EDGE('',*,*,#56418,.T.);
#83110=ORIENTED_EDGE('',*,*,#56466,.F.);
#83111=ORIENTED_EDGE('',*,*,#56227,.T.);
#83112=ORIENTED_EDGE('',*,*,#56097,.T.);
#83113=ORIENTED_EDGE('',*,*,#56222,.T.);
#83114=ORIENTED_EDGE('',*,*,#56466,.T.);
#83115=ORIENTED_EDGE('',*,*,#56417,.T.);
#83116=ORIENTED_EDGE('',*,*,#56452,.T.);
#83117=ORIENTED_EDGE('',*,*,#56420,.T.);
#83118=ORIENTED_EDGE('',*,*,#56465,.F.);
#83119=ORIENTED_EDGE('',*,*,#56219,.T.);
#83120=ORIENTED_EDGE('',*,*,#56024,.T.);
#83121=ORIENTED_EDGE('',*,*,#56415,.T.);
#83122=ORIENTED_EDGE('',*,*,#56304,.T.);
#83123=ORIENTED_EDGE('',*,*,#56212,.T.);
#83124=ORIENTED_EDGE('',*,*,#56297,.T.);
#83125=ORIENTED_EDGE('',*,*,#56408,.T.);
#83126=ORIENTED_EDGE('',*,*,#56020,.F.);
#83127=ORIENTED_EDGE('',*,*,#56213,.T.);
#83128=ORIENTED_EDGE('',*,*,#56015,.T.);
#83129=ORIENTED_EDGE('',*,*,#56410,.T.);
#83130=ORIENTED_EDGE('',*,*,#56299,.T.);
#83131=ORIENTED_EDGE('',*,*,#56218,.T.);
#83132=ORIENTED_EDGE('',*,*,#56301,.T.);
#83133=ORIENTED_EDGE('',*,*,#56412,.T.);
#83134=ORIENTED_EDGE('',*,*,#56011,.F.);
#83135=ORIENTED_EDGE('',*,*,#56210,.T.);
#83136=ORIENTED_EDGE('',*,*,#56008,.T.);
#83137=ORIENTED_EDGE('',*,*,#56406,.T.);
#83138=ORIENTED_EDGE('',*,*,#56295,.T.);
#83139=ORIENTED_EDGE('',*,*,#56215,.T.);
#83140=ORIENTED_EDGE('',*,*,#56298,.T.);
#83141=ORIENTED_EDGE('',*,*,#56409,.T.);
#83142=ORIENTED_EDGE('',*,*,#56004,.F.);
#83143=ORIENTED_EDGE('',*,*,#56207,.T.);
#83144=ORIENTED_EDGE('',*,*,#56467,.T.);
#83145=ORIENTED_EDGE('',*,*,#56403,.T.);
#83146=ORIENTED_EDGE('',*,*,#56293,.T.);
#83147=ORIENTED_EDGE('',*,*,#56156,.T.);
#83148=ORIENTED_EDGE('',*,*,#56256,.T.);
#83149=ORIENTED_EDGE('',*,*,#56354,.T.);
#83150=ORIENTED_EDGE('',*,*,#56468,.F.);
#83151=ORIENTED_EDGE('',*,*,#56206,.T.);
#83152=ORIENTED_EDGE('',*,*,#56083,.T.);
#83153=ORIENTED_EDGE('',*,*,#56157,.T.);
#83154=ORIENTED_EDGE('',*,*,#56468,.T.);
#83155=ORIENTED_EDGE('',*,*,#56353,.T.);
#83156=ORIENTED_EDGE('',*,*,#56453,.T.);
#83157=ORIENTED_EDGE('',*,*,#56404,.T.);
#83158=ORIENTED_EDGE('',*,*,#56467,.F.);
#83159=ORIENTED_EDGE('',*,*,#56200,.T.);
#83160=ORIENTED_EDGE('',*,*,#55998,.T.);
#83161=ORIENTED_EDGE('',*,*,#56397,.T.);
#83162=ORIENTED_EDGE('',*,*,#56287,.T.);
#83163=ORIENTED_EDGE('',*,*,#56205,.T.);
#83164=ORIENTED_EDGE('',*,*,#56291,.T.);
#83165=ORIENTED_EDGE('',*,*,#56401,.T.);
#83166=ORIENTED_EDGE('',*,*,#55994,.F.);
#83167=ORIENTED_EDGE('',*,*,#56203,.T.);
#83168=ORIENTED_EDGE('',*,*,#55990,.T.);
#83169=ORIENTED_EDGE('',*,*,#56399,.T.);
#83170=ORIENTED_EDGE('',*,*,#56289,.T.);
#83171=ORIENTED_EDGE('',*,*,#56209,.T.);
#83172=ORIENTED_EDGE('',*,*,#56292,.T.);
#83173=ORIENTED_EDGE('',*,*,#56402,.T.);
#83174=ORIENTED_EDGE('',*,*,#55986,.F.);
#83175=ORIENTED_EDGE('',*,*,#56194,.T.);
#83176=ORIENTED_EDGE('',*,*,#55983,.T.);
#83177=ORIENTED_EDGE('',*,*,#56391,.T.);
#83178=ORIENTED_EDGE('',*,*,#56281,.T.);
#83179=ORIENTED_EDGE('',*,*,#56199,.T.);
#83180=ORIENTED_EDGE('',*,*,#56285,.T.);
#83181=ORIENTED_EDGE('',*,*,#56395,.T.);
#83182=ORIENTED_EDGE('',*,*,#55979,.F.);
#83183=ORIENTED_EDGE('',*,*,#56197,.T.);
#83184=ORIENTED_EDGE('',*,*,#55975,.T.);
#83185=ORIENTED_EDGE('',*,*,#56393,.T.);
#83186=ORIENTED_EDGE('',*,*,#56283,.T.);
#83187=ORIENTED_EDGE('',*,*,#56202,.T.);
#83188=ORIENTED_EDGE('',*,*,#56286,.T.);
#83189=ORIENTED_EDGE('',*,*,#56396,.T.);
#83190=ORIENTED_EDGE('',*,*,#55971,.F.);
#83191=ORIENTED_EDGE('',*,*,#56191,.T.);
#83192=ORIENTED_EDGE('',*,*,#55967,.T.);
#83193=ORIENTED_EDGE('',*,*,#56388,.T.);
#83194=ORIENTED_EDGE('',*,*,#56278,.T.);
#83195=ORIENTED_EDGE('',*,*,#56196,.T.);
#83196=ORIENTED_EDGE('',*,*,#56280,.T.);
#83197=ORIENTED_EDGE('',*,*,#56390,.T.);
#83198=ORIENTED_EDGE('',*,*,#55963,.F.);
#83199=ORIENTED_EDGE('',*,*,#56188,.T.);
#83200=ORIENTED_EDGE('',*,*,#55959,.T.);
#83201=ORIENTED_EDGE('',*,*,#56384,.T.);
#83202=ORIENTED_EDGE('',*,*,#56274,.T.);
#83203=ORIENTED_EDGE('',*,*,#56193,.T.);
#83204=ORIENTED_EDGE('',*,*,#56277,.T.);
#83205=ORIENTED_EDGE('',*,*,#56387,.T.);
#83206=ORIENTED_EDGE('',*,*,#55955,.F.);
#83207=ORIENTED_EDGE('',*,*,#56185,.T.);
#83208=ORIENTED_EDGE('',*,*,#56469,.T.);
#83209=ORIENTED_EDGE('',*,*,#56381,.T.);
#83210=ORIENTED_EDGE('',*,*,#56272,.T.);
#83211=ORIENTED_EDGE('',*,*,#56122,.T.);
#83212=ORIENTED_EDGE('',*,*,#56236,.T.);
#83213=ORIENTED_EDGE('',*,*,#56320,.T.);
#83214=ORIENTED_EDGE('',*,*,#56470,.F.);
#83215=ORIENTED_EDGE('',*,*,#56184,.T.);
#83216=ORIENTED_EDGE('',*,*,#56069,.T.);
#83217=ORIENTED_EDGE('',*,*,#56123,.T.);
#83218=ORIENTED_EDGE('',*,*,#56470,.T.);
#83219=ORIENTED_EDGE('',*,*,#56319,.T.);
#83220=ORIENTED_EDGE('',*,*,#56460,.T.);
#83221=ORIENTED_EDGE('',*,*,#56382,.T.);
#83222=ORIENTED_EDGE('',*,*,#56469,.F.);
#83223=ORIENTED_EDGE('',*,*,#56175,.T.);
#83224=ORIENTED_EDGE('',*,*,#56471,.T.);
#83225=ORIENTED_EDGE('',*,*,#56371,.T.);
#83226=ORIENTED_EDGE('',*,*,#56266,.T.);
#83227=ORIENTED_EDGE('',*,*,#56180,.T.);
#83228=ORIENTED_EDGE('',*,*,#56270,.T.);
#83229=ORIENTED_EDGE('',*,*,#56378,.T.);
#83230=ORIENTED_EDGE('',*,*,#56472,.F.);
#83231=ORIENTED_EDGE('',*,*,#56174,.T.);
#83232=ORIENTED_EDGE('',*,*,#56073,.T.);
#83233=ORIENTED_EDGE('',*,*,#56181,.T.);
#83234=ORIENTED_EDGE('',*,*,#56472,.T.);
#83235=ORIENTED_EDGE('',*,*,#56377,.T.);
#83236=ORIENTED_EDGE('',*,*,#56458,.T.);
#83237=ORIENTED_EDGE('',*,*,#56372,.T.);
#83238=ORIENTED_EDGE('',*,*,#56471,.F.);
#83239=ORIENTED_EDGE('',*,*,#56178,.T.);
#83240=ORIENTED_EDGE('',*,*,#56473,.T.);
#83241=ORIENTED_EDGE('',*,*,#56374,.T.);
#83242=ORIENTED_EDGE('',*,*,#56268,.T.);
#83243=ORIENTED_EDGE('',*,*,#56187,.T.);
#83244=ORIENTED_EDGE('',*,*,#56271,.T.);
#83245=ORIENTED_EDGE('',*,*,#56380,.T.);
#83246=ORIENTED_EDGE('',*,*,#56474,.F.);
#83247=ORIENTED_EDGE('',*,*,#56182,.T.);
#83248=ORIENTED_EDGE('',*,*,#56071,.T.);
#83249=ORIENTED_EDGE('',*,*,#56183,.T.);
#83250=ORIENTED_EDGE('',*,*,#56474,.T.);
#83251=ORIENTED_EDGE('',*,*,#56379,.T.);
#83252=ORIENTED_EDGE('',*,*,#56459,.T.);
#83253=ORIENTED_EDGE('',*,*,#56375,.T.);
#83254=ORIENTED_EDGE('',*,*,#56473,.F.);
#83255=ORIENTED_EDGE('',*,*,#56170,.T.);
#83256=ORIENTED_EDGE('',*,*,#56264,.T.);
#83257=ORIENTED_EDGE('',*,*,#56368,.T.);
#83258=ORIENTED_EDGE('',*,*,#56475,.F.);
#83259=ORIENTED_EDGE('',*,*,#56165,.T.);
#83260=ORIENTED_EDGE('',*,*,#56077,.T.);
#83261=ORIENTED_EDGE('',*,*,#56171,.T.);
#83262=ORIENTED_EDGE('',*,*,#56475,.T.);
#83263=ORIENTED_EDGE('',*,*,#56367,.T.);
#83264=ORIENTED_EDGE('',*,*,#56456,.T.);
#83265=ORIENTED_EDGE('',*,*,#56362,.T.);
#83266=ORIENTED_EDGE('',*,*,#55950,.F.);
#83267=ORIENTED_EDGE('',*,*,#56168,.T.);
#83268=ORIENTED_EDGE('',*,*,#56476,.T.);
#83269=ORIENTED_EDGE('',*,*,#56364,.T.);
#83270=ORIENTED_EDGE('',*,*,#56262,.T.);
#83271=ORIENTED_EDGE('',*,*,#56177,.T.);
#83272=ORIENTED_EDGE('',*,*,#56265,.T.);
#83273=ORIENTED_EDGE('',*,*,#56370,.T.);
#83274=ORIENTED_EDGE('',*,*,#56477,.F.);
#83275=ORIENTED_EDGE('',*,*,#56172,.T.);
#83276=ORIENTED_EDGE('',*,*,#56075,.T.);
#83277=ORIENTED_EDGE('',*,*,#56173,.T.);
#83278=ORIENTED_EDGE('',*,*,#56477,.T.);
#83279=ORIENTED_EDGE('',*,*,#56369,.T.);
#83280=ORIENTED_EDGE('',*,*,#56457,.T.);
#83281=ORIENTED_EDGE('',*,*,#56365,.T.);
#83282=ORIENTED_EDGE('',*,*,#56476,.F.);
#83283=ORIENTED_EDGE('',*,*,#56161,.T.);
#83284=ORIENTED_EDGE('',*,*,#56478,.T.);
#83285=ORIENTED_EDGE('',*,*,#56357,.T.);
#83286=ORIENTED_EDGE('',*,*,#56258,.T.);
#83287=ORIENTED_EDGE('',*,*,#56167,.T.);
#83288=ORIENTED_EDGE('',*,*,#56260,.T.);
#83289=ORIENTED_EDGE('',*,*,#56361,.T.);
#83290=ORIENTED_EDGE('',*,*,#56479,.F.);
#83291=ORIENTED_EDGE('',*,*,#56160,.T.);
#83292=ORIENTED_EDGE('',*,*,#56079,.T.);
#83293=ORIENTED_EDGE('',*,*,#56164,.T.);
#83294=ORIENTED_EDGE('',*,*,#56479,.T.);
#83295=ORIENTED_EDGE('',*,*,#56360,.T.);
#83296=ORIENTED_EDGE('',*,*,#56455,.T.);
#83297=ORIENTED_EDGE('',*,*,#56358,.T.);
#83298=ORIENTED_EDGE('',*,*,#56478,.F.);
#83299=ORIENTED_EDGE('',*,*,#56154,.T.);
#83300=ORIENTED_EDGE('',*,*,#56480,.T.);
#83301=ORIENTED_EDGE('',*,*,#56350,.T.);
#83302=ORIENTED_EDGE('',*,*,#56254,.T.);
#83303=ORIENTED_EDGE('',*,*,#56163,.T.);
#83304=ORIENTED_EDGE('',*,*,#56257,.T.);
#83305=ORIENTED_EDGE('',*,*,#56356,.T.);
#83306=ORIENTED_EDGE('',*,*,#56481,.F.);
#83307=ORIENTED_EDGE('',*,*,#56158,.T.);
#83308=ORIENTED_EDGE('',*,*,#56081,.T.);
#83309=ORIENTED_EDGE('',*,*,#56159,.T.);
#83310=ORIENTED_EDGE('',*,*,#56481,.T.);
#83311=ORIENTED_EDGE('',*,*,#56355,.T.);
#83312=ORIENTED_EDGE('',*,*,#56454,.T.);
#83313=ORIENTED_EDGE('',*,*,#56351,.T.);
#83314=ORIENTED_EDGE('',*,*,#56480,.F.);
#83315=ORIENTED_EDGE('',*,*,#56151,.T.);
#83316=ORIENTED_EDGE('',*,*,#56482,.T.);
#83317=ORIENTED_EDGE('',*,*,#56347,.T.);
#83318=ORIENTED_EDGE('',*,*,#56252,.T.);
#83319=ORIENTED_EDGE('',*,*,#56142,.T.);
#83320=ORIENTED_EDGE('',*,*,#56248,.T.);
#83321=ORIENTED_EDGE('',*,*,#56340,.T.);
#83322=ORIENTED_EDGE('',*,*,#56483,.F.);
#83323=ORIENTED_EDGE('',*,*,#56150,.T.);
#83324=ORIENTED_EDGE('',*,*,#56105,.T.);
#83325=ORIENTED_EDGE('',*,*,#56143,.T.);
#83326=ORIENTED_EDGE('',*,*,#56483,.T.);
#83327=ORIENTED_EDGE('',*,*,#56339,.T.);
#83328=ORIENTED_EDGE('',*,*,#56448,.T.);
#83329=ORIENTED_EDGE('',*,*,#56348,.T.);
#83330=ORIENTED_EDGE('',*,*,#56482,.F.);
#83331=ORIENTED_EDGE('',*,*,#56137,.T.);
#83332=ORIENTED_EDGE('',*,*,#56484,.T.);
#83333=ORIENTED_EDGE('',*,*,#56333,.T.);
#83334=ORIENTED_EDGE('',*,*,#56244,.T.);
#83335=ORIENTED_EDGE('',*,*,#56153,.T.);
#83336=ORIENTED_EDGE('',*,*,#56251,.T.);
#83337=ORIENTED_EDGE('',*,*,#56346,.T.);
#83338=ORIENTED_EDGE('',*,*,#56485,.F.);
#83339=ORIENTED_EDGE('',*,*,#56136,.T.);
#83340=ORIENTED_EDGE('',*,*,#56107,.T.);
#83341=ORIENTED_EDGE('',*,*,#56149,.T.);
#83342=ORIENTED_EDGE('',*,*,#56485,.T.);
#83343=ORIENTED_EDGE('',*,*,#56345,.T.);
#83344=ORIENTED_EDGE('',*,*,#56447,.T.);
#83345=ORIENTED_EDGE('',*,*,#56334,.T.);
#83346=ORIENTED_EDGE('',*,*,#56484,.F.);
#83347=ORIENTED_EDGE('',*,*,#56140,.T.);
#83348=ORIENTED_EDGE('',*,*,#56486,.T.);
#83349=ORIENTED_EDGE('',*,*,#56336,.T.);
#83350=ORIENTED_EDGE('',*,*,#56246,.T.);
#83351=ORIENTED_EDGE('',*,*,#56144,.T.);
#83352=ORIENTED_EDGE('',*,*,#56103,.T.);
#83353=ORIENTED_EDGE('',*,*,#56145,.T.);
#83354=ORIENTED_EDGE('',*,*,#55948,.T.);
#83355=ORIENTED_EDGE('',*,*,#56341,.T.);
#83356=ORIENTED_EDGE('',*,*,#56449,.T.);
#83357=ORIENTED_EDGE('',*,*,#56337,.T.);
#83358=ORIENTED_EDGE('',*,*,#56486,.F.);
#83359=ORIENTED_EDGE('',*,*,#56132,.T.);
#83360=ORIENTED_EDGE('',*,*,#56487,.T.);
#83361=ORIENTED_EDGE('',*,*,#56328,.T.);
#83362=ORIENTED_EDGE('',*,*,#56241,.T.);
#83363=ORIENTED_EDGE('',*,*,#56139,.T.);
#83364=ORIENTED_EDGE('',*,*,#56243,.T.);
#83365=ORIENTED_EDGE('',*,*,#56332,.T.);
#83366=ORIENTED_EDGE('',*,*,#56488,.F.);
#83367=ORIENTED_EDGE('',*,*,#56131,.T.);
#83368=ORIENTED_EDGE('',*,*,#56109,.T.);
#83369=ORIENTED_EDGE('',*,*,#56135,.T.);
#83370=ORIENTED_EDGE('',*,*,#56488,.T.);
#83371=ORIENTED_EDGE('',*,*,#56331,.T.);
#83372=ORIENTED_EDGE('',*,*,#56446,.T.);
#83373=ORIENTED_EDGE('',*,*,#56329,.T.);
#83374=ORIENTED_EDGE('',*,*,#56487,.F.);
#83375=ORIENTED_EDGE('',*,*,#56127,.T.);
#83376=ORIENTED_EDGE('',*,*,#56489,.T.);
#83377=ORIENTED_EDGE('',*,*,#56323,.T.);
#83378=ORIENTED_EDGE('',*,*,#56238,.T.);
#83379=ORIENTED_EDGE('',*,*,#56134,.T.);
#83380=ORIENTED_EDGE('',*,*,#56240,.T.);
#83381=ORIENTED_EDGE('',*,*,#56327,.T.);
#83382=ORIENTED_EDGE('',*,*,#56490,.F.);
#83383=ORIENTED_EDGE('',*,*,#56126,.T.);
#83384=ORIENTED_EDGE('',*,*,#56111,.T.);
#83385=ORIENTED_EDGE('',*,*,#56130,.T.);
#83386=ORIENTED_EDGE('',*,*,#56490,.T.);
#83387=ORIENTED_EDGE('',*,*,#56326,.T.);
#83388=ORIENTED_EDGE('',*,*,#56445,.T.);
#83389=ORIENTED_EDGE('',*,*,#56324,.T.);
#83390=ORIENTED_EDGE('',*,*,#56489,.F.);
#83391=ORIENTED_EDGE('',*,*,#56060,.T.);
#83392=ORIENTED_EDGE('',*,*,#56491,.T.);
#83393=ORIENTED_EDGE('',*,*,#56050,.T.);
#83394=ORIENTED_EDGE('',*,*,#56056,.T.);
#83395=ORIENTED_EDGE('',*,*,#56129,.T.);
#83396=ORIENTED_EDGE('',*,*,#56237,.T.);
#83397=ORIENTED_EDGE('',*,*,#56322,.T.);
#83398=ORIENTED_EDGE('',*,*,#56492,.F.);
#83399=ORIENTED_EDGE('',*,*,#56059,.T.);
#83400=ORIENTED_EDGE('',*,*,#56113,.T.);
#83401=ORIENTED_EDGE('',*,*,#56125,.T.);
#83402=ORIENTED_EDGE('',*,*,#56492,.T.);
#83403=ORIENTED_EDGE('',*,*,#56321,.T.);
#83404=ORIENTED_EDGE('',*,*,#56444,.T.);
#83405=ORIENTED_EDGE('',*,*,#56051,.T.);
#83406=ORIENTED_EDGE('',*,*,#56491,.F.);
#83407=ORIENTED_EDGE('',*,*,#56120,.T.);
#83408=ORIENTED_EDGE('',*,*,#56493,.T.);
#83409=ORIENTED_EDGE('',*,*,#56316,.T.);
#83410=ORIENTED_EDGE('',*,*,#56234,.T.);
#83411=ORIENTED_EDGE('',*,*,#56061,.T.);
#83412=ORIENTED_EDGE('',*,*,#56057,.T.);
#83413=ORIENTED_EDGE('',*,*,#56054,.T.);
#83414=ORIENTED_EDGE('',*,*,#56494,.F.);
#83415=ORIENTED_EDGE('',*,*,#56124,.T.);
#83416=ORIENTED_EDGE('',*,*,#56067,.T.);
#83417=ORIENTED_EDGE('',*,*,#56062,.T.);
#83418=ORIENTED_EDGE('',*,*,#56494,.T.);
#83419=ORIENTED_EDGE('',*,*,#56053,.T.);
#83420=ORIENTED_EDGE('',*,*,#56443,.T.);
#83421=ORIENTED_EDGE('',*,*,#56317,.T.);
#83422=ORIENTED_EDGE('',*,*,#56493,.F.);
#83423=ORIENTED_EDGE('',*,*,#56116,.T.);
#83424=ORIENTED_EDGE('',*,*,#56495,.T.);
#83425=ORIENTED_EDGE('',*,*,#56118,.F.);
#83426=ORIENTED_EDGE('',*,*,#56496,.F.);
#83427=ORIENTED_EDGE('',*,*,#56114,.T.);
#83428=ORIENTED_EDGE('',*,*,#56496,.T.);
#83429=ORIENTED_EDGE('',*,*,#56117,.F.);
#83430=ORIENTED_EDGE('',*,*,#56064,.F.);
#83431=ORIENTED_EDGE('',*,*,#56115,.T.);
#83432=ORIENTED_EDGE('',*,*,#56066,.F.);
#83433=ORIENTED_EDGE('',*,*,#56119,.F.);
#83434=ORIENTED_EDGE('',*,*,#56495,.F.);
#87639=CYLINDRICAL_SURFACE('',#103552,25.2);
#87640=CYLINDRICAL_SURFACE('',#103554,25.611264);
#87641=CYLINDRICAL_SURFACE('',#103555,25.611264);
#87642=CYLINDRICAL_SURFACE('',#103556,3.36814799999999);
#87643=CYLINDRICAL_SURFACE('',#103559,3.36814799999999);
#87644=CYLINDRICAL_SURFACE('',#103562,3.36814799999999);
#87645=CYLINDRICAL_SURFACE('',#103565,3.36814799999999);
#87646=CYLINDRICAL_SURFACE('',#103568,3.36814799999999);
#87647=CYLINDRICAL_SURFACE('',#103571,3.36814799999999);
#87648=CYLINDRICAL_SURFACE('',#103574,3.36814799999999);
#87649=CYLINDRICAL_SURFACE('',#103577,3.36814799999999);
#87650=CYLINDRICAL_SURFACE('',#103580,3.36814799999999);
#87651=CYLINDRICAL_SURFACE('',#103583,3.36814799999999);
#87652=CYLINDRICAL_SURFACE('',#103586,3.36814799999999);
#87653=CYLINDRICAL_SURFACE('',#103589,3.36814799999999);
#87654=CYLINDRICAL_SURFACE('',#103595,54.361863151615);
#87655=CYLINDRICAL_SURFACE('',#103599,8.82);
#87656=CYLINDRICAL_SURFACE('',#103707,54.361863151615);
#87657=CYLINDRICAL_SURFACE('',#103709,54.361863151615);
#87658=CYLINDRICAL_SURFACE('',#103711,54.361863151615);
#87659=CYLINDRICAL_SURFACE('',#103713,54.361863151615);
#87660=CYLINDRICAL_SURFACE('',#103715,54.361863151615);
#87661=CYLINDRICAL_SURFACE('',#103717,54.361863151615);
#87662=CYLINDRICAL_SURFACE('',#103719,54.361863151615);
#87663=CYLINDRICAL_SURFACE('',#103721,54.361863151615);
#87664=CYLINDRICAL_SURFACE('',#103723,54.361863151615);
#87665=CYLINDRICAL_SURFACE('',#103725,54.361863151615);
#87666=CYLINDRICAL_SURFACE('',#103727,54.361863151615);
#87667=CYLINDRICAL_SURFACE('',#103729,54.361863151615);
#87668=CYLINDRICAL_SURFACE('',#103731,54.361863151615);
#87669=CYLINDRICAL_SURFACE('',#103733,54.361863151615);
#87670=CYLINDRICAL_SURFACE('',#103735,54.361863151615);
#87671=CYLINDRICAL_SURFACE('',#103737,54.361863151615);
#87672=CYLINDRICAL_SURFACE('',#103739,54.361863151615);
#87673=CYLINDRICAL_SURFACE('',#103741,54.361863151615);
#87674=CYLINDRICAL_SURFACE('',#103743,54.361863151615);
#87675=CYLINDRICAL_SURFACE('',#103745,54.361863151615);
#87676=CYLINDRICAL_SURFACE('',#103747,54.361863151615);
#87677=CYLINDRICAL_SURFACE('',#103749,54.361863151615);
#87678=CYLINDRICAL_SURFACE('',#103751,54.361863151615);
#87679=CYLINDRICAL_SURFACE('',#103753,54.361863151615);
#87680=CYLINDRICAL_SURFACE('',#103755,54.361863151615);
#87681=CYLINDRICAL_SURFACE('',#103757,54.361863151615);
#87682=CYLINDRICAL_SURFACE('',#103759,54.361863151615);
#87683=CYLINDRICAL_SURFACE('',#103761,54.361863151615);
#87684=CYLINDRICAL_SURFACE('',#103821,54.361863151615);
#87685=CYLINDRICAL_SURFACE('',#103844,25.611264);
#87686=CYLINDRICAL_SURFACE('',#103845,25.611264);
#87687=CYLINDRICAL_SURFACE('',#103846,3.36814799999999);
#87688=CYLINDRICAL_SURFACE('',#103847,25.611264);
#87689=CYLINDRICAL_SURFACE('',#103848,25.611264);
#87690=CYLINDRICAL_SURFACE('',#103849,3.36814799999999);
#87691=CYLINDRICAL_SURFACE('',#103850,25.611264);
#87692=CYLINDRICAL_SURFACE('',#103851,25.611264);
#87693=CYLINDRICAL_SURFACE('',#103852,25.611264);
#87694=CYLINDRICAL_SURFACE('',#103853,25.611264);
#87695=CYLINDRICAL_SURFACE('',#103854,25.611264);
#87696=CYLINDRICAL_SURFACE('',#103855,25.611264);
#87697=CYLINDRICAL_SURFACE('',#103856,25.611264);
#87698=CYLINDRICAL_SURFACE('',#103857,25.611264);
#87699=CYLINDRICAL_SURFACE('',#103858,3.36814799999999);
#87700=CYLINDRICAL_SURFACE('',#103859,25.611264);
#87701=CYLINDRICAL_SURFACE('',#103860,25.611264);
#87702=CYLINDRICAL_SURFACE('',#103861,25.611264);
#87703=CYLINDRICAL_SURFACE('',#103862,25.611264);
#87704=CYLINDRICAL_SURFACE('',#103863,25.611264);
#87705=CYLINDRICAL_SURFACE('',#103864,25.611264);
#87706=CYLINDRICAL_SURFACE('',#103865,25.611264);
#87707=CYLINDRICAL_SURFACE('',#103866,25.611264);
#87708=CYLINDRICAL_SURFACE('',#103867,3.36814799999999);
#87709=CYLINDRICAL_SURFACE('',#103868,25.611264);
#87710=CYLINDRICAL_SURFACE('',#103869,25.611264);
#87711=CYLINDRICAL_SURFACE('',#103870,25.611264);
#87712=CYLINDRICAL_SURFACE('',#103871,25.611264);
#87713=CYLINDRICAL_SURFACE('',#103872,25.611264);
#87714=CYLINDRICAL_SURFACE('',#103873,25.611264);
#87715=CYLINDRICAL_SURFACE('',#103874,25.611264);
#87716=CYLINDRICAL_SURFACE('',#103875,25.611264);
#87717=CYLINDRICAL_SURFACE('',#103876,25.611264);
#87718=CYLINDRICAL_SURFACE('',#103877,25.611264);
#87719=CYLINDRICAL_SURFACE('',#103878,25.611264);
#87720=CYLINDRICAL_SURFACE('',#103879,25.611264);
#87721=CYLINDRICAL_SURFACE('',#103880,25.611264);
#87722=CYLINDRICAL_SURFACE('',#103881,25.611264);
#87723=CYLINDRICAL_SURFACE('',#103882,3.36814799999999);
#87724=CYLINDRICAL_SURFACE('',#103883,25.611264);
#87725=CYLINDRICAL_SURFACE('',#103884,25.611264);
#87726=CYLINDRICAL_SURFACE('',#103885,3.36814799999999);
#87727=CYLINDRICAL_SURFACE('',#103886,25.611264);
#87728=CYLINDRICAL_SURFACE('',#103887,25.611264);
#87729=CYLINDRICAL_SURFACE('',#103888,3.36814799999999);
#87730=CYLINDRICAL_SURFACE('',#103889,25.611264);
#87731=CYLINDRICAL_SURFACE('',#103890,3.36814799999999);
#87732=CYLINDRICAL_SURFACE('',#103891,25.611264);
#87733=CYLINDRICAL_SURFACE('',#103892,25.611264);
#87734=CYLINDRICAL_SURFACE('',#103893,3.36814799999999);
#87735=CYLINDRICAL_SURFACE('',#103894,25.611264);
#87736=CYLINDRICAL_SURFACE('',#103895,25.611264);
#87737=CYLINDRICAL_SURFACE('',#103896,3.36814799999999);
#87738=CYLINDRICAL_SURFACE('',#103897,25.611264);
#87739=CYLINDRICAL_SURFACE('',#103898,25.611264);
#87740=CYLINDRICAL_SURFACE('',#103899,3.368148);
#87741=CYLINDRICAL_SURFACE('',#103900,25.611264);
#87742=CYLINDRICAL_SURFACE('',#103901,25.611264);
#87743=CYLINDRICAL_SURFACE('',#103902,3.368148);
#87744=CYLINDRICAL_SURFACE('',#103903,25.611264);
#87745=CYLINDRICAL_SURFACE('',#103904,25.611264);
#87746=CYLINDRICAL_SURFACE('',#103905,3.36814799999999);
#87747=CYLINDRICAL_SURFACE('',#103906,25.611264);
#87748=CYLINDRICAL_SURFACE('',#103907,3.36814799999999);
#87749=CYLINDRICAL_SURFACE('',#103908,25.611264);
#87750=CYLINDRICAL_SURFACE('',#103909,25.611264);
#87751=CYLINDRICAL_SURFACE('',#103910,3.36814799999999);
#87752=CYLINDRICAL_SURFACE('',#103911,25.611264);
#87753=CYLINDRICAL_SURFACE('',#103912,25.611264);
#87754=CYLINDRICAL_SURFACE('',#103913,3.36814799999999);
#87755=CYLINDRICAL_SURFACE('',#103914,25.611264);
#87756=CYLINDRICAL_SURFACE('',#103915,25.611264);
#87757=CYLINDRICAL_SURFACE('',#103916,3.36814799999999);
#87758=CYLINDRICAL_SURFACE('',#103917,25.611264);
#87759=CYLINDRICAL_SURFACE('',#103918,25.611264);
#87760=CYLINDRICAL_SURFACE('',#103919,3.36814799999999);
#93020=ADVANCED_FACE('',(#13741),#4055,.F.);
#93021=ADVANCED_FACE('',(#13742),#87639,.T.);
#93022=ADVANCED_FACE('',(#13743),#87640,.T.);
#93023=ADVANCED_FACE('',(#13744),#87641,.T.);
#93024=ADVANCED_FACE('',(#13745),#87642,.F.);
#93025=ADVANCED_FACE('',(#13746),#87643,.F.);
#93026=ADVANCED_FACE('',(#13747),#87644,.F.);
#93027=ADVANCED_FACE('',(#13748),#87645,.F.);
#93028=ADVANCED_FACE('',(#13749),#87646,.F.);
#93029=ADVANCED_FACE('',(#13750),#87647,.F.);
#93030=ADVANCED_FACE('',(#13751),#87648,.F.);
#93031=ADVANCED_FACE('',(#13752),#87649,.F.);
#93032=ADVANCED_FACE('',(#13753),#87650,.F.);
#93033=ADVANCED_FACE('',(#13754),#87651,.F.);
#93034=ADVANCED_FACE('',(#13755),#87652,.F.);
#93035=ADVANCED_FACE('',(#13756),#87653,.F.);
#93036=ADVANCED_FACE('',(#13757),#4056,.T.);
#93037=ADVANCED_FACE('',(#13758),#87654,.T.);
#93038=ADVANCED_FACE('',(#13759),#4057,.T.);
#93039=ADVANCED_FACE('',(#13760),#87655,.F.);
#93040=ADVANCED_FACE('',(#13761,#7627),#8535,.F.);
#93041=ADVANCED_FACE('',(#13762,#7628),#8536,.T.);
#93042=ADVANCED_FACE('',(#13763),#4058,.T.);
#93043=ADVANCED_FACE('',(#13764),#4059,.T.);
#93044=ADVANCED_FACE('',(#13765),#4060,.T.);
#93045=ADVANCED_FACE('',(#13766),#4061,.T.);
#93046=ADVANCED_FACE('',(#13767),#4062,.T.);
#93047=ADVANCED_FACE('',(#13768),#4063,.T.);
#93048=ADVANCED_FACE('',(#13769),#4064,.T.);
#93049=ADVANCED_FACE('',(#13770),#4065,.T.);
#93050=ADVANCED_FACE('',(#13771),#4066,.T.);
#93051=ADVANCED_FACE('',(#13772),#4067,.T.);
#93052=ADVANCED_FACE('',(#13773),#4068,.T.);
#93053=ADVANCED_FACE('',(#13774),#4069,.T.);
#93054=ADVANCED_FACE('',(#13775),#4070,.T.);
#93055=ADVANCED_FACE('',(#13776),#4071,.T.);
#93056=ADVANCED_FACE('',(#13777),#4072,.T.);
#93057=ADVANCED_FACE('',(#13778),#4073,.T.);
#93058=ADVANCED_FACE('',(#13779),#4074,.T.);
#93059=ADVANCED_FACE('',(#13780),#4075,.T.);
#93060=ADVANCED_FACE('',(#13781),#4076,.T.);
#93061=ADVANCED_FACE('',(#13782),#4077,.T.);
#93062=ADVANCED_FACE('',(#13783),#4078,.T.);
#93063=ADVANCED_FACE('',(#13784),#4079,.T.);
#93064=ADVANCED_FACE('',(#13785),#4080,.T.);
#93065=ADVANCED_FACE('',(#13786),#4081,.T.);
#93066=ADVANCED_FACE('',(#13787),#4082,.T.);
#93067=ADVANCED_FACE('',(#13788),#4083,.T.);
#93068=ADVANCED_FACE('',(#13789),#4084,.T.);
#93069=ADVANCED_FACE('',(#13790),#4085,.T.);
#93070=ADVANCED_FACE('',(#13791),#87656,.T.);
#93071=ADVANCED_FACE('',(#13792),#87657,.T.);
#93072=ADVANCED_FACE('',(#13793),#87658,.T.);
#93073=ADVANCED_FACE('',(#13794),#87659,.T.);
#93074=ADVANCED_FACE('',(#13795),#87660,.T.);
#93075=ADVANCED_FACE('',(#13796),#87661,.T.);
#93076=ADVANCED_FACE('',(#13797),#87662,.T.);
#93077=ADVANCED_FACE('',(#13798),#87663,.T.);
#93078=ADVANCED_FACE('',(#13799),#87664,.T.);
#93079=ADVANCED_FACE('',(#13800),#87665,.T.);
#93080=ADVANCED_FACE('',(#13801),#87666,.T.);
#93081=ADVANCED_FACE('',(#13802),#87667,.T.);
#93082=ADVANCED_FACE('',(#13803),#87668,.T.);
#93083=ADVANCED_FACE('',(#13804),#87669,.T.);
#93084=ADVANCED_FACE('',(#13805),#87670,.T.);
#93085=ADVANCED_FACE('',(#13806),#87671,.T.);
#93086=ADVANCED_FACE('',(#13807),#87672,.T.);
#93087=ADVANCED_FACE('',(#13808),#87673,.T.);
#93088=ADVANCED_FACE('',(#13809),#87674,.T.);
#93089=ADVANCED_FACE('',(#13810),#87675,.T.);
#93090=ADVANCED_FACE('',(#13811),#87676,.T.);
#93091=ADVANCED_FACE('',(#13812),#87677,.T.);
#93092=ADVANCED_FACE('',(#13813),#87678,.T.);
#93093=ADVANCED_FACE('',(#13814),#87679,.T.);
#93094=ADVANCED_FACE('',(#13815),#87680,.T.);
#93095=ADVANCED_FACE('',(#13816),#87681,.T.);
#93096=ADVANCED_FACE('',(#13817),#87682,.T.);
#93097=ADVANCED_FACE('',(#13818),#87683,.T.);
#93098=ADVANCED_FACE('',(#13819),#4086,.T.);
#93099=ADVANCED_FACE('',(#13820),#4087,.T.);
#93100=ADVANCED_FACE('',(#13821),#4088,.T.);
#93101=ADVANCED_FACE('',(#13822),#4089,.T.);
#93102=ADVANCED_FACE('',(#13823),#4090,.T.);
#93103=ADVANCED_FACE('',(#13824),#4091,.T.);
#93104=ADVANCED_FACE('',(#13825),#4092,.T.);
#93105=ADVANCED_FACE('',(#13826),#4093,.T.);
#93106=ADVANCED_FACE('',(#13827),#4094,.T.);
#93107=ADVANCED_FACE('',(#13828),#4095,.T.);
#93108=ADVANCED_FACE('',(#13829),#4096,.T.);
#93109=ADVANCED_FACE('',(#13830),#4097,.T.);
#93110=ADVANCED_FACE('',(#13831),#4098,.T.);
#93111=ADVANCED_FACE('',(#13832),#4099,.T.);
#93112=ADVANCED_FACE('',(#13833),#4100,.T.);
#93113=ADVANCED_FACE('',(#13834),#4101,.T.);
#93114=ADVANCED_FACE('',(#13835),#4102,.T.);
#93115=ADVANCED_FACE('',(#13836),#4103,.T.);
#93116=ADVANCED_FACE('',(#13837),#4104,.T.);
#93117=ADVANCED_FACE('',(#13838),#4105,.T.);
#93118=ADVANCED_FACE('',(#13839),#4106,.T.);
#93119=ADVANCED_FACE('',(#13840),#4107,.T.);
#93120=ADVANCED_FACE('',(#13841),#4108,.T.);
#93121=ADVANCED_FACE('',(#13842),#4109,.T.);
#93122=ADVANCED_FACE('',(#13843),#4110,.T.);
#93123=ADVANCED_FACE('',(#13844),#4111,.T.);
#93124=ADVANCED_FACE('',(#13845),#4112,.T.);
#93125=ADVANCED_FACE('',(#13846),#4113,.T.);
#93126=ADVANCED_FACE('',(#13847),#4114,.T.);
#93127=ADVANCED_FACE('',(#13848),#87684,.T.);
#93128=ADVANCED_FACE('',(#13849),#4115,.T.);
#93129=ADVANCED_FACE('',(#13850,#7629),#8537,.F.);
#93130=ADVANCED_FACE('',(#13851),#87685,.T.);
#93131=ADVANCED_FACE('',(#13852),#87686,.T.);
#93132=ADVANCED_FACE('',(#13853),#87687,.F.);
#93133=ADVANCED_FACE('',(#13854),#87688,.T.);
#93134=ADVANCED_FACE('',(#13855),#87689,.T.);
#93135=ADVANCED_FACE('',(#13856),#87690,.F.);
#93136=ADVANCED_FACE('',(#13857),#87691,.T.);
#93137=ADVANCED_FACE('',(#13858),#87692,.T.);
#93138=ADVANCED_FACE('',(#13859),#87693,.T.);
#93139=ADVANCED_FACE('',(#13860),#87694,.T.);
#93140=ADVANCED_FACE('',(#13861),#87695,.T.);
#93141=ADVANCED_FACE('',(#13862),#87696,.T.);
#93142=ADVANCED_FACE('',(#13863),#87697,.T.);
#93143=ADVANCED_FACE('',(#13864),#87698,.T.);
#93144=ADVANCED_FACE('',(#13865),#87699,.F.);
#93145=ADVANCED_FACE('',(#13866),#87700,.T.);
#93146=ADVANCED_FACE('',(#13867),#87701,.T.);
#93147=ADVANCED_FACE('',(#13868),#87702,.T.);
#93148=ADVANCED_FACE('',(#13869),#87703,.T.);
#93149=ADVANCED_FACE('',(#13870),#87704,.T.);
#93150=ADVANCED_FACE('',(#13871),#87705,.T.);
#93151=ADVANCED_FACE('',(#13872),#87706,.T.);
#93152=ADVANCED_FACE('',(#13873),#87707,.T.);
#93153=ADVANCED_FACE('',(#13874),#87708,.F.);
#93154=ADVANCED_FACE('',(#13875),#87709,.T.);
#93155=ADVANCED_FACE('',(#13876),#87710,.T.);
#93156=ADVANCED_FACE('',(#13877),#87711,.T.);
#93157=ADVANCED_FACE('',(#13878),#87712,.T.);
#93158=ADVANCED_FACE('',(#13879),#87713,.T.);
#93159=ADVANCED_FACE('',(#13880),#87714,.T.);
#93160=ADVANCED_FACE('',(#13881),#87715,.T.);
#93161=ADVANCED_FACE('',(#13882),#87716,.T.);
#93162=ADVANCED_FACE('',(#13883),#87717,.T.);
#93163=ADVANCED_FACE('',(#13884),#87718,.T.);
#93164=ADVANCED_FACE('',(#13885),#87719,.T.);
#93165=ADVANCED_FACE('',(#13886),#87720,.T.);
#93166=ADVANCED_FACE('',(#13887),#87721,.T.);
#93167=ADVANCED_FACE('',(#13888),#87722,.T.);
#93168=ADVANCED_FACE('',(#13889),#87723,.F.);
#93169=ADVANCED_FACE('',(#13890),#87724,.T.);
#93170=ADVANCED_FACE('',(#13891),#87725,.T.);
#93171=ADVANCED_FACE('',(#13892),#87726,.F.);
#93172=ADVANCED_FACE('',(#13893),#87727,.T.);
#93173=ADVANCED_FACE('',(#13894),#87728,.T.);
#93174=ADVANCED_FACE('',(#13895),#87729,.F.);
#93175=ADVANCED_FACE('',(#13896),#87730,.T.);
#93176=ADVANCED_FACE('',(#13897),#87731,.F.);
#93177=ADVANCED_FACE('',(#13898),#87732,.T.);
#93178=ADVANCED_FACE('',(#13899),#87733,.T.);
#93179=ADVANCED_FACE('',(#13900),#87734,.F.);
#93180=ADVANCED_FACE('',(#13901),#87735,.T.);
#93181=ADVANCED_FACE('',(#13902),#87736,.T.);
#93182=ADVANCED_FACE('',(#13903),#87737,.F.);
#93183=ADVANCED_FACE('',(#13904),#87738,.T.);
#93184=ADVANCED_FACE('',(#13905),#87739,.T.);
#93185=ADVANCED_FACE('',(#13906),#87740,.F.);
#93186=ADVANCED_FACE('',(#13907),#87741,.T.);
#93187=ADVANCED_FACE('',(#13908),#87742,.T.);
#93188=ADVANCED_FACE('',(#13909),#87743,.F.);
#93189=ADVANCED_FACE('',(#13910),#87744,.T.);
#93190=ADVANCED_FACE('',(#13911),#87745,.T.);
#93191=ADVANCED_FACE('',(#13912),#87746,.F.);
#93192=ADVANCED_FACE('',(#13913),#87747,.T.);
#93193=ADVANCED_FACE('',(#13914),#87748,.F.);
#93194=ADVANCED_FACE('',(#13915),#87749,.T.);
#93195=ADVANCED_FACE('',(#13916),#87750,.T.);
#93196=ADVANCED_FACE('',(#13917),#87751,.F.);
#93197=ADVANCED_FACE('',(#13918),#87752,.T.);
#93198=ADVANCED_FACE('',(#13919),#87753,.T.);
#93199=ADVANCED_FACE('',(#13920),#87754,.F.);
#93200=ADVANCED_FACE('',(#13921),#87755,.T.);
#93201=ADVANCED_FACE('',(#13922),#87756,.T.);
#93202=ADVANCED_FACE('',(#13923),#87757,.F.);
#93203=ADVANCED_FACE('',(#13924),#87758,.T.);
#93204=ADVANCED_FACE('',(#13925),#87759,.T.);
#93205=ADVANCED_FACE('',(#13926),#87760,.F.);
#93206=ADVANCED_FACE('',(#13927),#8538,.T.);
#93207=ADVANCED_FACE('',(#13928),#8539,.T.);
#93208=ADVANCED_FACE('',(#13929),#8540,.T.);
#93731=CLOSED_SHELL('',(#93020,#93021,#93022,#93023,#93024,#93025,#93026,
#93027,#93028,#93029,#93030,#93031,#93032,#93033,#93034,#93035,#93036,#93037,
#93038,#93039,#93040,#93041,#93042,#93043,#93044,#93045,#93046,#93047,#93048,
#93049,#93050,#93051,#93052,#93053,#93054,#93055,#93056,#93057,#93058,#93059,
#93060,#93061,#93062,#93063,#93064,#93065,#93066,#93067,#93068,#93069,#93070,
#93071,#93072,#93073,#93074,#93075,#93076,#93077,#93078,#93079,#93080,#93081,
#93082,#93083,#93084,#93085,#93086,#93087,#93088,#93089,#93090,#93091,#93092,
#93093,#93094,#93095,#93096,#93097,#93098,#93099,#93100,#93101,#93102,#93103,
#93104,#93105,#93106,#93107,#93108,#93109,#93110,#93111,#93112,#93113,#93114,
#93115,#93116,#93117,#93118,#93119,#93120,#93121,#93122,#93123,#93124,#93125,
#93126,#93127,#93128,#93129,#93130,#93131,#93132,#93133,#93134,#93135,#93136,
#93137,#93138,#93139,#93140,#93141,#93142,#93143,#93144,#93145,#93146,#93147,
#93148,#93149,#93150,#93151,#93152,#93153,#93154,#93155,#93156,#93157,#93158,
#93159,#93160,#93161,#93162,#93163,#93164,#93165,#93166,#93167,#93168,#93169,
#93170,#93171,#93172,#93173,#93174,#93175,#93176,#93177,#93178,#93179,#93180,
#93181,#93182,#93183,#93184,#93185,#93186,#93187,#93188,#93189,#93190,#93191,
#93192,#93193,#93194,#93195,#93196,#93197,#93198,#93199,#93200,#93201,#93202,
#93203,#93204,#93205,#93206,#93207,#93208));
#103547=AXIS2_PLACEMENT_3D('',#272463,#127837,#127838);
#103548=AXIS2_PLACEMENT_3D('',#272464,#127839,#127840);
#103549=AXIS2_PLACEMENT_3D('',#272466,#127841,#127842);
#103550=AXIS2_PLACEMENT_3D('',#272468,#127843,#127844);
#103551=AXIS2_PLACEMENT_3D('',#272469,#127845,#127846);
#103552=AXIS2_PLACEMENT_3D('',#272470,#127847,#127848);
#103553=AXIS2_PLACEMENT_3D('',#272473,#127850,#127851);
#103554=AXIS2_PLACEMENT_3D('',#272474,#127852,#127853);
#103555=AXIS2_PLACEMENT_3D('',#272495,#127856,#127857);
#103556=AXIS2_PLACEMENT_3D('',#272516,#127860,#127861);
#103557=AXIS2_PLACEMENT_3D('',#272519,#127862,#127863);
#103558=AXIS2_PLACEMENT_3D('',#272539,#127865,#127866);
#103559=AXIS2_PLACEMENT_3D('',#272559,#127868,#127869);
#103560=AXIS2_PLACEMENT_3D('',#272562,#127870,#127871);
#103561=AXIS2_PLACEMENT_3D('',#272582,#127873,#127874);
#103562=AXIS2_PLACEMENT_3D('',#272602,#127876,#127877);
#103563=AXIS2_PLACEMENT_3D('',#272605,#127878,#127879);
#103564=AXIS2_PLACEMENT_3D('',#272625,#127881,#127882);
#103565=AXIS2_PLACEMENT_3D('',#272645,#127884,#127885);
#103566=AXIS2_PLACEMENT_3D('',#272648,#127886,#127887);
#103567=AXIS2_PLACEMENT_3D('',#272668,#127889,#127890);
#103568=AXIS2_PLACEMENT_3D('',#272688,#127892,#127893);
#103569=AXIS2_PLACEMENT_3D('',#272705,#127895,#127896);
#103570=AXIS2_PLACEMENT_3D('',#272726,#127898,#127899);
#103571=AXIS2_PLACEMENT_3D('',#272727,#127900,#127901);
#103572=AXIS2_PLACEMENT_3D('',#272744,#127903,#127904);
#103573=AXIS2_PLACEMENT_3D('',#272765,#127906,#127907);
#103574=AXIS2_PLACEMENT_3D('',#272766,#127908,#127909);
#103575=AXIS2_PLACEMENT_3D('',#272776,#127910,#127911);
#103576=AXIS2_PLACEMENT_3D('',#272796,#127913,#127914);
#103577=AXIS2_PLACEMENT_3D('',#272805,#127916,#127917);
#103578=AXIS2_PLACEMENT_3D('',#272808,#127918,#127919);
#103579=AXIS2_PLACEMENT_3D('',#272828,#127921,#127922);
#103580=AXIS2_PLACEMENT_3D('',#272848,#127924,#127925);
#103581=AXIS2_PLACEMENT_3D('',#272858,#127926,#127927);
#103582=AXIS2_PLACEMENT_3D('',#272878,#127929,#127930);
#103583=AXIS2_PLACEMENT_3D('',#272887,#127932,#127933);
#103584=AXIS2_PLACEMENT_3D('',#272890,#127934,#127935);
#103585=AXIS2_PLACEMENT_3D('',#272910,#127937,#127938);
#103586=AXIS2_PLACEMENT_3D('',#272930,#127940,#127941);
#103587=AXIS2_PLACEMENT_3D('',#272933,#127942,#127943);
#103588=AXIS2_PLACEMENT_3D('',#272953,#127945,#127946);
#103589=AXIS2_PLACEMENT_3D('',#272973,#127948,#127949);
#103590=AXIS2_PLACEMENT_3D('',#272976,#127950,#127951);
#103591=AXIS2_PLACEMENT_3D('',#272996,#127953,#127954);
#103592=AXIS2_PLACEMENT_3D('',#273016,#127956,#127957);
#103593=AXIS2_PLACEMENT_3D('',#273019,#127958,#127959);
#103594=AXIS2_PLACEMENT_3D('',#273039,#127960,#127961);
#103595=AXIS2_PLACEMENT_3D('',#273053,#127962,#127963);
#103596=AXIS2_PLACEMENT_3D('',#273056,#127964,#127965);
#103597=AXIS2_PLACEMENT_3D('',#273059,#127968,#127969);
#103598=AXIS2_PLACEMENT_3D('',#273062,#127970,#127971);
#103599=AXIS2_PLACEMENT_3D('',#273095,#127972,#127973);
#103600=AXIS2_PLACEMENT_3D('',#273098,#127974,#127975);
#103601=AXIS2_PLACEMENT_3D('',#273102,#127977,#127978);
#103602=AXIS2_PLACEMENT_3D('',#273104,#127980,#127981);
#103603=AXIS2_PLACEMENT_3D('',#273106,#127982,#127983);
#103604=AXIS2_PLACEMENT_3D('',#273108,#127984,#127985);
#103605=AXIS2_PLACEMENT_3D('',#273110,#127986,#127987);
#103606=AXIS2_PLACEMENT_3D('',#273112,#127988,#127989);
#103607=AXIS2_PLACEMENT_3D('',#273114,#127990,#127991);
#103608=AXIS2_PLACEMENT_3D('',#273116,#127992,#127993);
#103609=AXIS2_PLACEMENT_3D('',#273118,#127994,#127995);
#103610=AXIS2_PLACEMENT_3D('',#273120,#127996,#127997);
#103611=AXIS2_PLACEMENT_3D('',#273122,#127998,#127999);
#103612=AXIS2_PLACEMENT_3D('',#273124,#128000,#128001);
#103613=AXIS2_PLACEMENT_3D('',#273126,#128002,#128003);
#103614=AXIS2_PLACEMENT_3D('',#273128,#128004,#128005);
#103615=AXIS2_PLACEMENT_3D('',#273130,#128006,#128007);
#103616=AXIS2_PLACEMENT_3D('',#273132,#128008,#128009);
#103617=AXIS2_PLACEMENT_3D('',#273134,#128010,#128011);
#103618=AXIS2_PLACEMENT_3D('',#273136,#128012,#128013);
#103619=AXIS2_PLACEMENT_3D('',#273138,#128014,#128015);
#103620=AXIS2_PLACEMENT_3D('',#273139,#128016,#128017);
#103621=AXIS2_PLACEMENT_3D('',#273140,#128018,#128019);
#103622=AXIS2_PLACEMENT_3D('',#273141,#128020,#128021);
#103623=AXIS2_PLACEMENT_3D('',#273142,#128022,#128023);
#103624=AXIS2_PLACEMENT_3D('',#273143,#128024,#128025);
#103625=AXIS2_PLACEMENT_3D('',#273144,#128026,#128027);
#103626=AXIS2_PLACEMENT_3D('',#273145,#128028,#128029);
#103627=AXIS2_PLACEMENT_3D('',#273146,#128030,#128031);
#103628=AXIS2_PLACEMENT_3D('',#273147,#128032,#128033);
#103629=AXIS2_PLACEMENT_3D('',#273148,#128034,#128035);
#103630=AXIS2_PLACEMENT_3D('',#273149,#128036,#128037);
#103631=AXIS2_PLACEMENT_3D('',#273150,#128038,#128039);
#103632=AXIS2_PLACEMENT_3D('',#273152,#128040,#128041);
#103633=AXIS2_PLACEMENT_3D('',#273154,#128042,#128043);
#103634=AXIS2_PLACEMENT_3D('',#273156,#128044,#128045);
#103635=AXIS2_PLACEMENT_3D('',#273158,#128046,#128047);
#103636=AXIS2_PLACEMENT_3D('',#273160,#128048,#128049);
#103637=AXIS2_PLACEMENT_3D('',#273162,#128050,#128051);
#103638=AXIS2_PLACEMENT_3D('',#273164,#128052,#128053);
#103639=AXIS2_PLACEMENT_3D('',#273166,#128054,#128055);
#103640=AXIS2_PLACEMENT_3D('',#273168,#128056,#128057);
#103641=AXIS2_PLACEMENT_3D('',#273170,#128058,#128059);
#103642=AXIS2_PLACEMENT_3D('',#273172,#128060,#128061);
#103643=AXIS2_PLACEMENT_3D('',#273174,#128062,#128063);
#103644=AXIS2_PLACEMENT_3D('',#273176,#128064,#128065);
#103645=AXIS2_PLACEMENT_3D('',#273178,#128066,#128067);
#103646=AXIS2_PLACEMENT_3D('',#273180,#128068,#128069);
#103647=AXIS2_PLACEMENT_3D('',#273182,#128070,#128071);
#103648=AXIS2_PLACEMENT_3D('',#273184,#128072,#128073);
#103649=AXIS2_PLACEMENT_3D('',#273185,#128074,#128075);
#103650=AXIS2_PLACEMENT_3D('',#273191,#128079,#128080);
#103651=AXIS2_PLACEMENT_3D('',#273197,#128084,#128085);
#103652=AXIS2_PLACEMENT_3D('',#273209,#128086,#128087);
#103653=AXIS2_PLACEMENT_3D('',#273233,#128088,#128089);
#103654=AXIS2_PLACEMENT_3D('',#273262,#128090,#128091);
#103655=AXIS2_PLACEMENT_3D('',#273269,#128092,#128093);
#103656=AXIS2_PLACEMENT_3D('',#273298,#128094,#128095);
#103657=AXIS2_PLACEMENT_3D('',#273305,#128096,#128097);
#103658=AXIS2_PLACEMENT_3D('',#273334,#128098,#128099);
#103659=AXIS2_PLACEMENT_3D('',#273341,#128100,#128101);
#103660=AXIS2_PLACEMENT_3D('',#273353,#128102,#128103);
#103661=AXIS2_PLACEMENT_3D('',#273377,#128104,#128105);
#103662=AXIS2_PLACEMENT_3D('',#273404,#128106,#128107);
#103663=AXIS2_PLACEMENT_3D('',#273405,#128108,#128109);
#103664=AXIS2_PLACEMENT_3D('',#273434,#128110,#128111);
#103665=AXIS2_PLACEMENT_3D('',#273441,#128112,#128113);
#103666=AXIS2_PLACEMENT_3D('',#273453,#128114,#128115);
#103667=AXIS2_PLACEMENT_3D('',#273477,#128116,#128117);
#103668=AXIS2_PLACEMENT_3D('',#273506,#128118,#128119);
#103669=AXIS2_PLACEMENT_3D('',#273513,#128120,#128121);
#103670=AXIS2_PLACEMENT_3D('',#273532,#128122,#128123);
#103671=AXIS2_PLACEMENT_3D('',#273539,#128124,#128125);
#103672=AXIS2_PLACEMENT_3D('',#273551,#128126,#128127);
#103673=AXIS2_PLACEMENT_3D('',#273575,#128128,#128129);
#103674=AXIS2_PLACEMENT_3D('',#273604,#128130,#128131);
#103675=AXIS2_PLACEMENT_3D('',#273611,#128132,#128133);
#103676=AXIS2_PLACEMENT_3D('',#273623,#128134,#128135);
#103677=AXIS2_PLACEMENT_3D('',#273647,#128136,#128137);
#103678=AXIS2_PLACEMENT_3D('',#273676,#128138,#128139);
#103679=AXIS2_PLACEMENT_3D('',#273683,#128140,#128141);
#103680=AXIS2_PLACEMENT_3D('',#273694,#128142,#128143);
#103681=AXIS2_PLACEMENT_3D('',#273701,#128144,#128145);
#103682=AXIS2_PLACEMENT_3D('',#273712,#128146,#128147);
#103683=AXIS2_PLACEMENT_3D('',#273719,#128148,#128149);
#103684=AXIS2_PLACEMENT_3D('',#273730,#128150,#128151);
#103685=AXIS2_PLACEMENT_3D('',#273737,#128152,#128153);
#103686=AXIS2_PLACEMENT_3D('',#273748,#128154,#128155);
#103687=AXIS2_PLACEMENT_3D('',#273755,#128156,#128157);
#103688=AXIS2_PLACEMENT_3D('',#273766,#128158,#128159);
#103689=AXIS2_PLACEMENT_3D('',#273773,#128160,#128161);
#103690=AXIS2_PLACEMENT_3D('',#273784,#128162,#128163);
#103691=AXIS2_PLACEMENT_3D('',#273791,#128164,#128165);
#103692=AXIS2_PLACEMENT_3D('',#273809,#128166,#128167);
#103693=AXIS2_PLACEMENT_3D('',#273816,#128168,#128169);
#103694=AXIS2_PLACEMENT_3D('',#273827,#128170,#128171);
#103695=AXIS2_PLACEMENT_3D('',#273834,#128172,#128173);
#103696=AXIS2_PLACEMENT_3D('',#273845,#128174,#128175);
#103697=AXIS2_PLACEMENT_3D('',#273852,#128176,#128177);
#103698=AXIS2_PLACEMENT_3D('',#273863,#128178,#128179);
#103699=AXIS2_PLACEMENT_3D('',#273870,#128180,#128181);
#103700=AXIS2_PLACEMENT_3D('',#273881,#128182,#128183);
#103701=AXIS2_PLACEMENT_3D('',#273899,#128184,#128185);
#103702=AXIS2_PLACEMENT_3D('',#273911,#128186,#128187);
#103703=AXIS2_PLACEMENT_3D('',#273935,#128188,#128189);
#103704=AXIS2_PLACEMENT_3D('',#273946,#128190,#128191);
#103705=AXIS2_PLACEMENT_3D('',#273953,#128192,#128193);
#103706=AXIS2_PLACEMENT_3D('',#273964,#128194,#128195);
#103707=AXIS2_PLACEMENT_3D('',#273971,#128196,#128197);
#103708=AXIS2_PLACEMENT_3D('',#273975,#128199,#128200);
#103709=AXIS2_PLACEMENT_3D('',#273977,#128202,#128203);
#103710=AXIS2_PLACEMENT_3D('',#273982,#128206,#128207);
#103711=AXIS2_PLACEMENT_3D('',#273983,#128208,#128209);
#103712=AXIS2_PLACEMENT_3D('',#273988,#128212,#128213);
#103713=AXIS2_PLACEMENT_3D('',#273989,#128214,#128215);
#103714=AXIS2_PLACEMENT_3D('',#273994,#128218,#128219);
#103715=AXIS2_PLACEMENT_3D('',#273995,#128220,#128221);
#103716=AXIS2_PLACEMENT_3D('',#273999,#128223,#128224);
#103717=AXIS2_PLACEMENT_3D('',#274001,#128226,#128227);
#103718=AXIS2_PLACEMENT_3D('',#274004,#128229,#128230);
#103719=AXIS2_PLACEMENT_3D('',#274005,#128231,#128232);
#103720=AXIS2_PLACEMENT_3D('',#274010,#128235,#128236);
#103721=AXIS2_PLACEMENT_3D('',#274011,#128237,#128238);
#103722=AXIS2_PLACEMENT_3D('',#274015,#128240,#128241);
#103723=AXIS2_PLACEMENT_3D('',#274017,#128243,#128244);
#103724=AXIS2_PLACEMENT_3D('',#274022,#128247,#128248);
#103725=AXIS2_PLACEMENT_3D('',#274023,#128249,#128250);
#103726=AXIS2_PLACEMENT_3D('',#274026,#128252,#128253);
#103727=AXIS2_PLACEMENT_3D('',#274027,#128254,#128255);
#103728=AXIS2_PLACEMENT_3D('',#274031,#128257,#128258);
#103729=AXIS2_PLACEMENT_3D('',#274033,#128260,#128261);
#103730=AXIS2_PLACEMENT_3D('',#274038,#128264,#128265);
#103731=AXIS2_PLACEMENT_3D('',#274039,#128266,#128267);
#103732=AXIS2_PLACEMENT_3D('',#274043,#128269,#128270);
#103733=AXIS2_PLACEMENT_3D('',#274045,#128272,#128273);
#103734=AXIS2_PLACEMENT_3D('',#274050,#128276,#128277);
#103735=AXIS2_PLACEMENT_3D('',#274051,#128278,#128279);
#103736=AXIS2_PLACEMENT_3D('',#274055,#128281,#128282);
#103737=AXIS2_PLACEMENT_3D('',#274057,#128284,#128285);
#103738=AXIS2_PLACEMENT_3D('',#274062,#128288,#128289);
#103739=AXIS2_PLACEMENT_3D('',#274063,#128290,#128291);
#103740=AXIS2_PLACEMENT_3D('',#274068,#128294,#128295);
#103741=AXIS2_PLACEMENT_3D('',#274069,#128296,#128297);
#103742=AXIS2_PLACEMENT_3D('',#274073,#128299,#128300);
#103743=AXIS2_PLACEMENT_3D('',#274075,#128302,#128303);
#103744=AXIS2_PLACEMENT_3D('',#274080,#128306,#128307);
#103745=AXIS2_PLACEMENT_3D('',#274081,#128308,#128309);
#103746=AXIS2_PLACEMENT_3D('',#274085,#128311,#128312);
#103747=AXIS2_PLACEMENT_3D('',#274087,#128314,#128315);
#103748=AXIS2_PLACEMENT_3D('',#274092,#128318,#128319);
#103749=AXIS2_PLACEMENT_3D('',#274093,#128320,#128321);
#103750=AXIS2_PLACEMENT_3D('',#274097,#128323,#128324);
#103751=AXIS2_PLACEMENT_3D('',#274099,#128326,#128327);
#103752=AXIS2_PLACEMENT_3D('',#274104,#128330,#128331);
#103753=AXIS2_PLACEMENT_3D('',#274105,#128332,#128333);
#103754=AXIS2_PLACEMENT_3D('',#274110,#128336,#128337);
#103755=AXIS2_PLACEMENT_3D('',#274111,#128338,#128339);
#103756=AXIS2_PLACEMENT_3D('',#274115,#128341,#128342);
#103757=AXIS2_PLACEMENT_3D('',#274117,#128344,#128345);
#103758=AXIS2_PLACEMENT_3D('',#274121,#128347,#128348);
#103759=AXIS2_PLACEMENT_3D('',#274123,#128350,#128351);
#103760=AXIS2_PLACEMENT_3D('',#274128,#128354,#128355);
#103761=AXIS2_PLACEMENT_3D('',#274129,#128356,#128357);
#103762=AXIS2_PLACEMENT_3D('',#274134,#128360,#128361);
#103763=AXIS2_PLACEMENT_3D('',#274135,#128362,#128363);
#103764=AXIS2_PLACEMENT_3D('',#274155,#128364,#128365);
#103765=AXIS2_PLACEMENT_3D('',#274169,#128366,#128367);
#103766=AXIS2_PLACEMENT_3D('',#274202,#128368,#128369);
#103767=AXIS2_PLACEMENT_3D('',#274203,#128370,#128371);
#103768=AXIS2_PLACEMENT_3D('',#274236,#128372,#128373);
#103769=AXIS2_PLACEMENT_3D('',#274237,#128374,#128375);
#103770=AXIS2_PLACEMENT_3D('',#274270,#128376,#128377);
#103771=AXIS2_PLACEMENT_3D('',#274271,#128378,#128379);
#103772=AXIS2_PLACEMENT_3D('',#274291,#128380,#128381);
#103773=AXIS2_PLACEMENT_3D('',#274305,#128382,#128383);
#103774=AXIS2_PLACEMENT_3D('',#274329,#128384,#128385);
#103775=AXIS2_PLACEMENT_3D('',#274330,#128386,#128387);
#103776=AXIS2_PLACEMENT_3D('',#274363,#128388,#128389);
#103777=AXIS2_PLACEMENT_3D('',#274364,#128390,#128391);
#103778=AXIS2_PLACEMENT_3D('',#274384,#128392,#128393);
#103779=AXIS2_PLACEMENT_3D('',#274398,#128394,#128395);
#103780=AXIS2_PLACEMENT_3D('',#274431,#128396,#128397);
#103781=AXIS2_PLACEMENT_3D('',#274432,#128398,#128399);
#103782=AXIS2_PLACEMENT_3D('',#274458,#128400,#128401);
#103783=AXIS2_PLACEMENT_3D('',#274459,#128402,#128403);
#103784=AXIS2_PLACEMENT_3D('',#274479,#128404,#128405);
#103785=AXIS2_PLACEMENT_3D('',#274493,#128406,#128407);
#103786=AXIS2_PLACEMENT_3D('',#274526,#128408,#128409);
#103787=AXIS2_PLACEMENT_3D('',#274527,#128410,#128411);
#103788=AXIS2_PLACEMENT_3D('',#274547,#128412,#128413);
#103789=AXIS2_PLACEMENT_3D('',#274561,#128414,#128415);
#103790=AXIS2_PLACEMENT_3D('',#274594,#128416,#128417);
#103791=AXIS2_PLACEMENT_3D('',#274595,#128418,#128419);
#103792=AXIS2_PLACEMENT_3D('',#274602,#128420,#128421);
#103793=AXIS2_PLACEMENT_3D('',#274611,#128422,#128423);
#103794=AXIS2_PLACEMENT_3D('',#274626,#128424,#128425);
#103795=AXIS2_PLACEMENT_3D('',#274627,#128426,#128427);
#103796=AXIS2_PLACEMENT_3D('',#274642,#128428,#128429);
#103797=AXIS2_PLACEMENT_3D('',#274643,#128430,#128431);
#103798=AXIS2_PLACEMENT_3D('',#274650,#128432,#128433);
#103799=AXIS2_PLACEMENT_3D('',#274659,#128434,#128435);
#103800=AXIS2_PLACEMENT_3D('',#274674,#128436,#128437);
#103801=AXIS2_PLACEMENT_3D('',#274675,#128438,#128439);
#103802=AXIS2_PLACEMENT_3D('',#274682,#128440,#128441);
#103803=AXIS2_PLACEMENT_3D('',#274691,#128442,#128443);
#103804=AXIS2_PLACEMENT_3D('',#274718,#128444,#128445);
#103805=AXIS2_PLACEMENT_3D('',#274719,#128446,#128447);
#103806=AXIS2_PLACEMENT_3D('',#274726,#128448,#128449);
#103807=AXIS2_PLACEMENT_3D('',#274735,#128450,#128451);
#103808=AXIS2_PLACEMENT_3D('',#274750,#128452,#128453);
#103809=AXIS2_PLACEMENT_3D('',#274751,#128454,#128455);
#103810=AXIS2_PLACEMENT_3D('',#274766,#128456,#128457);
#103811=AXIS2_PLACEMENT_3D('',#274767,#128458,#128459);
#103812=AXIS2_PLACEMENT_3D('',#274775,#128460,#128461);
#103813=AXIS2_PLACEMENT_3D('',#274789,#128462,#128463);
#103814=AXIS2_PLACEMENT_3D('',#274809,#128464,#128465);
#103815=AXIS2_PLACEMENT_3D('',#274823,#128466,#128467);
#103816=AXIS2_PLACEMENT_3D('',#274838,#128468,#128469);
#103817=AXIS2_PLACEMENT_3D('',#274839,#128470,#128471);
#103818=AXIS2_PLACEMENT_3D('',#274854,#128472,#128473);
#103819=AXIS2_PLACEMENT_3D('',#274855,#128474,#128475);
#103820=AXIS2_PLACEMENT_3D('',#274884,#128476,#128477);
#103821=AXIS2_PLACEMENT_3D('',#274891,#128478,#128479);
#103822=AXIS2_PLACEMENT_3D('',#274896,#128482,#128483);
#103823=AXIS2_PLACEMENT_3D('',#274897,#128484,#128485);
#103824=AXIS2_PLACEMENT_3D('',#274930,#128486,#128487);
#103825=AXIS2_PLACEMENT_3D('',#274931,#128488,#128489);
#103826=AXIS2_PLACEMENT_3D('',#274932,#128490,#128491);
#103827=AXIS2_PLACEMENT_3D('',#274933,#128492,#128493);
#103828=AXIS2_PLACEMENT_3D('',#274934,#128494,#128495);
#103829=AXIS2_PLACEMENT_3D('',#274935,#128496,#128497);
#103830=AXIS2_PLACEMENT_3D('',#274936,#128498,#128499);
#103831=AXIS2_PLACEMENT_3D('',#274937,#128500,#128501);
#103832=AXIS2_PLACEMENT_3D('',#274938,#128502,#128503);
#103833=AXIS2_PLACEMENT_3D('',#274939,#128504,#128505);
#103834=AXIS2_PLACEMENT_3D('',#274940,#128506,#128507);
#103835=AXIS2_PLACEMENT_3D('',#274941,#128508,#128509);
#103836=AXIS2_PLACEMENT_3D('',#274942,#128510,#128511);
#103837=AXIS2_PLACEMENT_3D('',#274943,#128512,#128513);
#103838=AXIS2_PLACEMENT_3D('',#274944,#128514,#128515);
#103839=AXIS2_PLACEMENT_3D('',#274945,#128516,#128517);
#103840=AXIS2_PLACEMENT_3D('',#274946,#128518,#128519);
#103841=AXIS2_PLACEMENT_3D('',#274947,#128520,#128521);
#103842=AXIS2_PLACEMENT_3D('',#274948,#128522,#128523);
#103843=AXIS2_PLACEMENT_3D('',#274949,#128524,#128525);
#103844=AXIS2_PLACEMENT_3D('',#274950,#128526,#128527);
#103845=AXIS2_PLACEMENT_3D('',#274952,#128529,#128530);
#103846=AXIS2_PLACEMENT_3D('',#274954,#128532,#128533);
#103847=AXIS2_PLACEMENT_3D('',#274955,#128534,#128535);
#103848=AXIS2_PLACEMENT_3D('',#274957,#128537,#128538);
#103849=AXIS2_PLACEMENT_3D('',#274959,#128540,#128541);
#103850=AXIS2_PLACEMENT_3D('',#274960,#128542,#128543);
#103851=AXIS2_PLACEMENT_3D('',#274961,#128544,#128545);
#103852=AXIS2_PLACEMENT_3D('',#274962,#128546,#128547);
#103853=AXIS2_PLACEMENT_3D('',#274963,#128548,#128549);
#103854=AXIS2_PLACEMENT_3D('',#274964,#128550,#128551);
#103855=AXIS2_PLACEMENT_3D('',#274965,#128552,#128553);
#103856=AXIS2_PLACEMENT_3D('',#274966,#128554,#128555);
#103857=AXIS2_PLACEMENT_3D('',#274968,#128557,#128558);
#103858=AXIS2_PLACEMENT_3D('',#274970,#128560,#128561);
#103859=AXIS2_PLACEMENT_3D('',#274971,#128562,#128563);
#103860=AXIS2_PLACEMENT_3D('',#274972,#128564,#128565);
#103861=AXIS2_PLACEMENT_3D('',#274973,#128566,#128567);
#103862=AXIS2_PLACEMENT_3D('',#274974,#128568,#128569);
#103863=AXIS2_PLACEMENT_3D('',#274975,#128570,#128571);
#103864=AXIS2_PLACEMENT_3D('',#274976,#128572,#128573);
#103865=AXIS2_PLACEMENT_3D('',#274977,#128574,#128575);
#103866=AXIS2_PLACEMENT_3D('',#274979,#128577,#128578);
#103867=AXIS2_PLACEMENT_3D('',#274981,#128580,#128581);
#103868=AXIS2_PLACEMENT_3D('',#274982,#128582,#128583);
#103869=AXIS2_PLACEMENT_3D('',#274983,#128584,#128585);
#103870=AXIS2_PLACEMENT_3D('',#274984,#128586,#128587);
#103871=AXIS2_PLACEMENT_3D('',#274985,#128588,#128589);
#103872=AXIS2_PLACEMENT_3D('',#274986,#128590,#128591);
#103873=AXIS2_PLACEMENT_3D('',#274987,#128592,#128593);
#103874=AXIS2_PLACEMENT_3D('',#274988,#128594,#128595);
#103875=AXIS2_PLACEMENT_3D('',#274989,#128596,#128597);
#103876=AXIS2_PLACEMENT_3D('',#274990,#128598,#128599);
#103877=AXIS2_PLACEMENT_3D('',#274991,#128600,#128601);
#103878=AXIS2_PLACEMENT_3D('',#274992,#128602,#128603);
#103879=AXIS2_PLACEMENT_3D('',#274993,#128604,#128605);
#103880=AXIS2_PLACEMENT_3D('',#274994,#128606,#128607);
#103881=AXIS2_PLACEMENT_3D('',#274996,#128609,#128610);
#103882=AXIS2_PLACEMENT_3D('',#274998,#128612,#128613);
#103883=AXIS2_PLACEMENT_3D('',#274999,#128614,#128615);
#103884=AXIS2_PLACEMENT_3D('',#275001,#128617,#128618);
#103885=AXIS2_PLACEMENT_3D('',#275003,#128620,#128621);
#103886=AXIS2_PLACEMENT_3D('',#275004,#128622,#128623);
#103887=AXIS2_PLACEMENT_3D('',#275006,#128625,#128626);
#103888=AXIS2_PLACEMENT_3D('',#275008,#128628,#128629);
#103889=AXIS2_PLACEMENT_3D('',#275009,#128630,#128631);
#103890=AXIS2_PLACEMENT_3D('',#275011,#128633,#128634);
#103891=AXIS2_PLACEMENT_3D('',#275012,#128635,#128636);
#103892=AXIS2_PLACEMENT_3D('',#275014,#128638,#128639);
#103893=AXIS2_PLACEMENT_3D('',#275016,#128641,#128642);
#103894=AXIS2_PLACEMENT_3D('',#275017,#128643,#128644);
#103895=AXIS2_PLACEMENT_3D('',#275019,#128646,#128647);
#103896=AXIS2_PLACEMENT_3D('',#275021,#128649,#128650);
#103897=AXIS2_PLACEMENT_3D('',#275022,#128651,#128652);
#103898=AXIS2_PLACEMENT_3D('',#275024,#128654,#128655);
#103899=AXIS2_PLACEMENT_3D('',#275026,#128657,#128658);
#103900=AXIS2_PLACEMENT_3D('',#275027,#128659,#128660);
#103901=AXIS2_PLACEMENT_3D('',#275029,#128662,#128663);
#103902=AXIS2_PLACEMENT_3D('',#275031,#128665,#128666);
#103903=AXIS2_PLACEMENT_3D('',#275032,#128667,#128668);
#103904=AXIS2_PLACEMENT_3D('',#275034,#128670,#128671);
#103905=AXIS2_PLACEMENT_3D('',#275036,#128673,#128674);
#103906=AXIS2_PLACEMENT_3D('',#275037,#128675,#128676);
#103907=AXIS2_PLACEMENT_3D('',#275039,#128678,#128679);
#103908=AXIS2_PLACEMENT_3D('',#275040,#128680,#128681);
#103909=AXIS2_PLACEMENT_3D('',#275042,#128683,#128684);
#103910=AXIS2_PLACEMENT_3D('',#275044,#128686,#128687);
#103911=AXIS2_PLACEMENT_3D('',#275045,#128688,#128689);
#103912=AXIS2_PLACEMENT_3D('',#275047,#128691,#128692);
#103913=AXIS2_PLACEMENT_3D('',#275049,#128694,#128695);
#103914=AXIS2_PLACEMENT_3D('',#275050,#128696,#128697);
#103915=AXIS2_PLACEMENT_3D('',#275052,#128699,#128700);
#103916=AXIS2_PLACEMENT_3D('',#275054,#128702,#128703);
#103917=AXIS2_PLACEMENT_3D('',#275055,#128704,#128705);
#103918=AXIS2_PLACEMENT_3D('',#275057,#128707,#128708);
#103919=AXIS2_PLACEMENT_3D('',#275059,#128710,#128711);
#103920=AXIS2_PLACEMENT_3D('',#275060,#128712,#128713);
#103921=AXIS2_PLACEMENT_3D('',#275063,#128716,#128717);
#103922=AXIS2_PLACEMENT_3D('',#275064,#128718,#128719);
#127837=DIRECTION('axis',(0.,0.,1.));
#127838=DIRECTION('refdir',(1.,0.,0.));
#127839=DIRECTION('center_axis',(1.,0.,0.));
#127840=DIRECTION('ref_axis',(0.,0.,-1.));
#127841=DIRECTION('center_axis',(1.,0.,0.));
#127842=DIRECTION('ref_axis',(0.,0.,-1.));
#127843=DIRECTION('center_axis',(0.,1.,8.58242907100461E-17));
#127844=DIRECTION('ref_axis',(0.,-8.58242907100461E-17,1.));
#127845=DIRECTION('center_axis',(-1.,0.,0.));
#127846=DIRECTION('ref_axis',(0.,0.,-1.));
#127847=DIRECTION('center_axis',(1.,0.,0.));
#127848=DIRECTION('ref_axis',(0.,0.,-1.));
#127849=DIRECTION('',(-1.,0.,0.));
#127850=DIRECTION('center_axis',(-1.,0.,0.));
#127851=DIRECTION('ref_axis',(0.,0.,1.));
#127852=DIRECTION('center_axis',(-1.,0.,0.));
#127853=DIRECTION('ref_axis',(0.,0.,1.));
#127854=DIRECTION('',(-1.,0.,0.));
#127855=DIRECTION('',(-1.,0.,0.));
#127856=DIRECTION('center_axis',(-1.,0.,0.));
#127857=DIRECTION('ref_axis',(0.,0.,1.));
#127858=DIRECTION('',(-1.,0.,0.));
#127859=DIRECTION('',(1.,0.,0.));
#127860=DIRECTION('center_axis',(-1.,0.,0.));
#127861=DIRECTION('ref_axis',(0.,0.,1.));
#127862=DIRECTION('center_axis',(1.,0.,0.));
#127863=DIRECTION('ref_axis',(0.,0.994521895368274,-0.104528463267644));
#127864=DIRECTION('',(-1.,0.,0.));
#127865=DIRECTION('center_axis',(-1.,0.,0.));
#127866=DIRECTION('ref_axis',(0.,0.,-1.));
#127867=DIRECTION('',(-1.,0.,0.));
#127868=DIRECTION('center_axis',(-1.,0.,0.));
#127869=DIRECTION('ref_axis',(0.,0.,1.));
#127870=DIRECTION('center_axis',(1.,0.,0.));
#127871=DIRECTION('ref_axis',(0.,0.951056516295157,-0.309016994374938));
#127872=DIRECTION('',(-1.,0.,0.));
#127873=DIRECTION('center_axis',(-1.,0.,0.));
#127874=DIRECTION('ref_axis',(0.,-2.06015112872333E-15,-1.));
#127875=DIRECTION('',(-1.,0.,0.));
#127876=DIRECTION('center_axis',(-1.,0.,0.));
#127877=DIRECTION('ref_axis',(0.,0.,1.));
#127878=DIRECTION('center_axis',(1.,0.,0.));
#127879=DIRECTION('ref_axis',(0.,0.743144825477399,-0.669130606358852));
#127880=DIRECTION('',(-1.,0.,0.));
#127881=DIRECTION('center_axis',(-1.,0.,0.));
#127882=DIRECTION('ref_axis',(0.,0.,-1.));
#127883=DIRECTION('',(-1.,0.,0.));
#127884=DIRECTION('center_axis',(-1.,0.,0.));
#127885=DIRECTION('ref_axis',(0.,0.,1.));
#127886=DIRECTION('center_axis',(1.,0.,0.));
#127887=DIRECTION('ref_axis',(0.,0.866025403784443,-0.499999999999993));
#127888=DIRECTION('',(-1.,0.,0.));
#127889=DIRECTION('center_axis',(-1.,0.,0.));
#127890=DIRECTION('ref_axis',(0.,0.,-1.));
#127891=DIRECTION('',(-1.,0.,0.));
#127892=DIRECTION('center_axis',(-1.,0.,0.));
#127893=DIRECTION('ref_axis',(0.,0.,1.));
#127894=DIRECTION('',(-1.,0.,0.));
#127895=DIRECTION('center_axis',(-1.,0.,0.));
#127896=DIRECTION('ref_axis',(0.,4.12030225744667E-15,-1.));
#127897=DIRECTION('',(-1.,0.,0.));
#127898=DIRECTION('center_axis',(1.,0.,0.));
#127899=DIRECTION('ref_axis',(0.,0.406736643075806,-0.913545457642598));
#127900=DIRECTION('center_axis',(-1.,0.,0.));
#127901=DIRECTION('ref_axis',(0.,0.,1.));
#127902=DIRECTION('',(-1.,0.,0.));
#127903=DIRECTION('center_axis',(-1.,0.,0.));
#127904=DIRECTION('ref_axis',(0.,0.,-1.));
#127905=DIRECTION('',(-1.,0.,0.));
#127906=DIRECTION('center_axis',(1.,0.,0.));
#127907=DIRECTION('ref_axis',(0.,0.58778525229248,-0.809016994374943));
#127908=DIRECTION('center_axis',(-1.,0.,0.));
#127909=DIRECTION('ref_axis',(0.,0.,1.));
#127910=DIRECTION('center_axis',(1.,0.,0.));
#127911=DIRECTION('ref_axis',(0.,0.587785252292463,0.809016994374955));
#127912=DIRECTION('',(-1.,0.,0.));
#127913=DIRECTION('center_axis',(-1.,0.,0.));
#127914=DIRECTION('ref_axis',(0.,0.,-1.));
#127915=DIRECTION('',(-1.,0.,0.));
#127916=DIRECTION('center_axis',(-1.,0.,0.));
#127917=DIRECTION('ref_axis',(0.,0.,1.));
#127918=DIRECTION('center_axis',(1.,0.,0.));
#127919=DIRECTION('ref_axis',(0.,0.743144825477386,0.669130606358867));
#127920=DIRECTION('',(-1.,0.,0.));
#127921=DIRECTION('center_axis',(-1.,0.,0.));
#127922=DIRECTION('ref_axis',(0.,0.,-1.));
#127923=DIRECTION('',(-1.,0.,0.));
#127924=DIRECTION('center_axis',(-1.,0.,0.));
#127925=DIRECTION('ref_axis',(0.,0.,1.));
#127926=DIRECTION('center_axis',(1.,0.,0.));
#127927=DIRECTION('ref_axis',(0.,0.406736643075789,0.913545457642606));
#127928=DIRECTION('',(-1.,0.,0.));
#127929=DIRECTION('center_axis',(-1.,0.,0.));
#127930=DIRECTION('ref_axis',(0.,0.,-1.));
#127931=DIRECTION('',(-1.,0.,0.));
#127932=DIRECTION('center_axis',(-1.,0.,0.));
#127933=DIRECTION('ref_axis',(0.,0.,1.));
#127934=DIRECTION('center_axis',(1.,0.,0.));
#127935=DIRECTION('ref_axis',(0.,0.866025403784433,0.50000000000001));
#127936=DIRECTION('',(-1.,0.,0.));
#127937=DIRECTION('center_axis',(-1.,0.,0.));
#127938=DIRECTION('ref_axis',(0.,0.,-1.));
#127939=DIRECTION('',(-1.,0.,0.));
#127940=DIRECTION('center_axis',(-1.,0.,0.));
#127941=DIRECTION('ref_axis',(0.,0.,1.));
#127942=DIRECTION('center_axis',(1.,0.,0.));
#127943=DIRECTION('ref_axis',(0.,0.951056516295151,0.309016994374957));
#127944=DIRECTION('',(-1.,0.,0.));
#127945=DIRECTION('center_axis',(-1.,0.,0.));
#127946=DIRECTION('ref_axis',(0.,0.,-1.));
#127947=DIRECTION('',(-1.,0.,0.));
#127948=DIRECTION('center_axis',(-1.,0.,0.));
#127949=DIRECTION('ref_axis',(0.,0.,1.));
#127950=DIRECTION('center_axis',(1.,0.,0.));
#127951=DIRECTION('ref_axis',(0.,0.994521895368272,0.104528463267663));
#127952=DIRECTION('',(-1.,0.,0.));
#127953=DIRECTION('center_axis',(-1.,0.,0.));
#127954=DIRECTION('ref_axis',(0.,3.60526447526583E-15,-1.));
#127955=DIRECTION('',(-1.,0.,0.));
#127956=DIRECTION('center_axis',(-1.,0.,0.));
#127957=DIRECTION('ref_axis',(0.,0.,1.));
#127958=DIRECTION('center_axis',(-1.,0.,0.));
#127959=DIRECTION('ref_axis',(0.,0.,1.));
#127960=DIRECTION('center_axis',(-1.,0.,0.));
#127961=DIRECTION('ref_axis',(0.,0.,1.));
#127962=DIRECTION('center_axis',(-1.,0.,0.));
#127963=DIRECTION('ref_axis',(0.,0.,1.));
#127964=DIRECTION('center_axis',(-1.,0.,0.));
#127965=DIRECTION('ref_axis',(0.,0.,1.));
#127966=DIRECTION('',(1.,0.,0.));
#127967=DIRECTION('',(-1.,0.,0.));
#127968=DIRECTION('center_axis',(-1.,0.,0.));
#127969=DIRECTION('ref_axis',(0.,0.,1.));
#127970=DIRECTION('center_axis',(-1.,0.,0.));
#127971=DIRECTION('ref_axis',(0.,0.,1.));
#127972=DIRECTION('center_axis',(-1.,0.,0.));
#127973=DIRECTION('ref_axis',(0.,-1.,-1.83697019872103E-16));
#127974=DIRECTION('center_axis',(1.,0.,0.));
#127975=DIRECTION('ref_axis',(0.,0.,1.));
#127976=DIRECTION('',(-1.,0.,0.));
#127977=DIRECTION('center_axis',(1.,0.,0.));
#127978=DIRECTION('ref_axis',(0.,0.,1.));
#127979=DIRECTION('',(1.,0.,0.));
#127980=DIRECTION('center_axis',(-1.,0.,0.));
#127981=DIRECTION('ref_axis',(0.,0.,1.));
#127982=DIRECTION('center_axis',(1.,0.,0.));
#127983=DIRECTION('ref_axis',(0.,-0.994521895368273,-0.104528463267657));
#127984=DIRECTION('center_axis',(-1.,0.,0.));
#127985=DIRECTION('ref_axis',(0.,0.,1.));
#127986=DIRECTION('center_axis',(1.,0.,0.));
#127987=DIRECTION('ref_axis',(0.,-0.951056516295153,-0.30901699437495));
#127988=DIRECTION('center_axis',(-1.,0.,0.));
#127989=DIRECTION('ref_axis',(0.,0.,1.));
#127990=DIRECTION('center_axis',(1.,0.,0.));
#127991=DIRECTION('ref_axis',(0.,-0.866025403784437,-0.500000000000003));
#127992=DIRECTION('center_axis',(-1.,0.,0.));
#127993=DIRECTION('ref_axis',(0.,0.,1.));
#127994=DIRECTION('center_axis',(1.,0.,0.));
#127995=DIRECTION('ref_axis',(0.,-0.74314482547739,-0.669130606358862));
#127996=DIRECTION('center_axis',(-1.,0.,0.));
#127997=DIRECTION('ref_axis',(0.,0.,1.));
#127998=DIRECTION('center_axis',(1.,0.,0.));
#127999=DIRECTION('ref_axis',(0.,-0.587785252292469,-0.80901699437495));
#128000=DIRECTION('center_axis',(-1.,0.,0.));
#128001=DIRECTION('ref_axis',(0.,0.,1.));
#128002=DIRECTION('center_axis',(1.,0.,0.));
#128003=DIRECTION('ref_axis',(0.,-0.406736643075793,-0.913545457642604));
#128004=DIRECTION('center_axis',(-1.,0.,0.));
#128005=DIRECTION('ref_axis',(0.,0.,1.));
#128006=DIRECTION('center_axis',(1.,0.,0.));
#128007=DIRECTION('ref_axis',(0.,-0.207911690817753,-0.978147600733807));
#128008=DIRECTION('center_axis',(-1.,0.,0.));
#128009=DIRECTION('ref_axis',(0.,0.,1.));
#128010=DIRECTION('center_axis',(1.,0.,0.));
#128011=DIRECTION('ref_axis',(0.,8.24060451489334E-15,-1.));
#128012=DIRECTION('center_axis',(-1.,0.,0.));
#128013=DIRECTION('ref_axis',(0.,0.,1.));
#128014=DIRECTION('center_axis',(1.,0.,0.));
#128015=DIRECTION('ref_axis',(0.,0.207911690817766,-0.978147600733804));
#128016=DIRECTION('center_axis',(-1.,0.,0.));
#128017=DIRECTION('ref_axis',(0.,0.,1.));
#128018=DIRECTION('center_axis',(-1.,0.,0.));
#128019=DIRECTION('ref_axis',(0.,0.,1.));
#128020=DIRECTION('center_axis',(-1.,0.,0.));
#128021=DIRECTION('ref_axis',(0.,0.,1.));
#128022=DIRECTION('center_axis',(-1.,0.,0.));
#128023=DIRECTION('ref_axis',(0.,0.,1.));
#128024=DIRECTION('center_axis',(-1.,0.,0.));
#128025=DIRECTION('ref_axis',(0.,0.,1.));
#128026=DIRECTION('center_axis',(-1.,0.,0.));
#128027=DIRECTION('ref_axis',(0.,0.,1.));
#128028=DIRECTION('center_axis',(-1.,0.,0.));
#128029=DIRECTION('ref_axis',(0.,0.,1.));
#128030=DIRECTION('center_axis',(-1.,0.,0.));
#128031=DIRECTION('ref_axis',(0.,0.,1.));
#128032=DIRECTION('center_axis',(-1.,0.,0.));
#128033=DIRECTION('ref_axis',(0.,0.,1.));
#128034=DIRECTION('center_axis',(-1.,0.,0.));
#128035=DIRECTION('ref_axis',(0.,0.,1.));
#128036=DIRECTION('center_axis',(-1.,0.,0.));
#128037=DIRECTION('ref_axis',(0.,0.,1.));
#128038=DIRECTION('center_axis',(-1.,0.,0.));
#128039=DIRECTION('ref_axis',(0.,0.,1.));
#128040=DIRECTION('center_axis',(-1.,0.,0.));
#128041=DIRECTION('ref_axis',(0.,0.,1.));
#128042=DIRECTION('center_axis',(1.,0.,0.));
#128043=DIRECTION('ref_axis',(0.,0.207911690817747,0.978147600733808));
#128044=DIRECTION('center_axis',(-1.,0.,0.));
#128045=DIRECTION('ref_axis',(0.,0.,1.));
#128046=DIRECTION('center_axis',(1.,0.,0.));
#128047=DIRECTION('ref_axis',(0.,0.,1.));
#128048=DIRECTION('center_axis',(-1.,0.,0.));
#128049=DIRECTION('ref_axis',(0.,0.,1.));
#128050=DIRECTION('center_axis',(1.,0.,0.));
#128051=DIRECTION('ref_axis',(0.,-0.20791169081776,0.978147600733806));
#128052=DIRECTION('center_axis',(-1.,0.,0.));
#128053=DIRECTION('ref_axis',(0.,0.,1.));
#128054=DIRECTION('center_axis',(1.,0.,0.));
#128055=DIRECTION('ref_axis',(0.,-0.406736643075801,0.9135454576426));
#128056=DIRECTION('center_axis',(-1.,0.,0.));
#128057=DIRECTION('ref_axis',(0.,0.,1.));
#128058=DIRECTION('center_axis',(1.,0.,0.));
#128059=DIRECTION('ref_axis',(0.,-0.587785252292474,0.809016994374947));
#128060=DIRECTION('center_axis',(-1.,0.,0.));
#128061=DIRECTION('ref_axis',(0.,0.,1.));
#128062=DIRECTION('center_axis',(1.,0.,0.));
#128063=DIRECTION('ref_axis',(0.,-0.743144825477395,0.669130606358857));
#128064=DIRECTION('center_axis',(-1.,0.,0.));
#128065=DIRECTION('ref_axis',(0.,0.,1.));
#128066=DIRECTION('center_axis',(1.,0.,0.));
#128067=DIRECTION('ref_axis',(0.,-0.866025403784439,0.499999999999999));
#128068=DIRECTION('center_axis',(-1.,0.,0.));
#128069=DIRECTION('ref_axis',(0.,0.,1.));
#128070=DIRECTION('center_axis',(1.,0.,0.));
#128071=DIRECTION('ref_axis',(0.,-0.951056516295155,0.309016994374944));
#128072=DIRECTION('center_axis',(-1.,0.,0.));
#128073=DIRECTION('ref_axis',(0.,0.,1.));
#128074=DIRECTION('center_axis',(1.,0.,0.));
#128075=DIRECTION('ref_axis',(0.,-0.994521895368274,0.104528463267651));
#128076=DIRECTION('',(0.,1.,0.));
#128077=DIRECTION('',(0.,-1.,0.));
#128078=DIRECTION('',(0.,0.,1.));
#128079=DIRECTION('center_axis',(-1.,0.,0.));
#128080=DIRECTION('ref_axis',(0.,0.,1.));
#128081=DIRECTION('',(0.,1.,0.));
#128082=DIRECTION('',(0.,0.,1.));
#128083=DIRECTION('',(0.,-1.,0.));
#128084=DIRECTION('center_axis',(-1.,0.,0.));
#128085=DIRECTION('ref_axis',(0.,0.,1.));
#128086=DIRECTION('center_axis',(-1.,0.,0.));
#128087=DIRECTION('ref_axis',(0.,0.,1.));
#128088=DIRECTION('center_axis',(-1.,0.,0.));
#128089=DIRECTION('ref_axis',(0.,0.,1.));
#128090=DIRECTION('center_axis',(-1.,0.,0.));
#128091=DIRECTION('ref_axis',(0.,0.,1.));
#128092=DIRECTION('center_axis',(-1.,0.,0.));
#128093=DIRECTION('ref_axis',(0.,0.,1.));
#128094=DIRECTION('center_axis',(-1.,0.,0.));
#128095=DIRECTION('ref_axis',(0.,0.,1.));
#128096=DIRECTION('center_axis',(-1.,0.,0.));
#128097=DIRECTION('ref_axis',(0.,0.,1.));
#128098=DIRECTION('center_axis',(-1.,0.,0.));
#128099=DIRECTION('ref_axis',(0.,0.,1.));
#128100=DIRECTION('center_axis',(-1.,0.,0.));
#128101=DIRECTION('ref_axis',(0.,0.,1.));
#128102=DIRECTION('center_axis',(-1.,0.,0.));
#128103=DIRECTION('ref_axis',(0.,0.,1.));
#128104=DIRECTION('center_axis',(-1.,0.,0.));
#128105=DIRECTION('ref_axis',(0.,0.,1.));
#128106=DIRECTION('center_axis',(-1.,0.,0.));
#128107=DIRECTION('ref_axis',(0.,0.,1.));
#128108=DIRECTION('center_axis',(-1.,0.,0.));
#128109=DIRECTION('ref_axis',(0.,0.,1.));
#128110=DIRECTION('center_axis',(-1.,0.,0.));
#128111=DIRECTION('ref_axis',(0.,0.,1.));
#128112=DIRECTION('center_axis',(-1.,0.,0.));
#128113=DIRECTION('ref_axis',(0.,0.,1.));
#128114=DIRECTION('center_axis',(-1.,0.,0.));
#128115=DIRECTION('ref_axis',(0.,0.,1.));
#128116=DIRECTION('center_axis',(-1.,0.,0.));
#128117=DIRECTION('ref_axis',(0.,0.,1.));
#128118=DIRECTION('center_axis',(-1.,0.,0.));
#128119=DIRECTION('ref_axis',(0.,0.,1.));
#128120=DIRECTION('center_axis',(-1.,0.,0.));
#128121=DIRECTION('ref_axis',(0.,0.,1.));
#128122=DIRECTION('center_axis',(-1.,0.,0.));
#128123=DIRECTION('ref_axis',(0.,0.,1.));
#128124=DIRECTION('center_axis',(-1.,0.,0.));
#128125=DIRECTION('ref_axis',(0.,0.,1.));
#128126=DIRECTION('center_axis',(-1.,0.,0.));
#128127=DIRECTION('ref_axis',(0.,0.,1.));
#128128=DIRECTION('center_axis',(-1.,0.,0.));
#128129=DIRECTION('ref_axis',(0.,0.,1.));
#128130=DIRECTION('center_axis',(-1.,0.,0.));
#128131=DIRECTION('ref_axis',(0.,0.,1.));
#128132=DIRECTION('center_axis',(-1.,0.,0.));
#128133=DIRECTION('ref_axis',(0.,0.,1.));
#128134=DIRECTION('center_axis',(-1.,0.,0.));
#128135=DIRECTION('ref_axis',(0.,0.,1.));
#128136=DIRECTION('center_axis',(-1.,0.,0.));
#128137=DIRECTION('ref_axis',(0.,0.,1.));
#128138=DIRECTION('center_axis',(-1.,0.,0.));
#128139=DIRECTION('ref_axis',(0.,0.,1.));
#128140=DIRECTION('center_axis',(-1.,0.,0.));
#128141=DIRECTION('ref_axis',(0.,9.62924104759778E-15,-1.));
#128142=DIRECTION('center_axis',(-1.,0.,0.));
#128143=DIRECTION('ref_axis',(0.,0.,1.));
#128144=DIRECTION('center_axis',(-1.,0.,0.));
#128145=DIRECTION('ref_axis',(0.,0.,1.));
#128146=DIRECTION('center_axis',(-1.,0.,0.));
#128147=DIRECTION('ref_axis',(0.,0.,1.));
#128148=DIRECTION('center_axis',(-1.,0.,0.));
#128149=DIRECTION('ref_axis',(0.,0.,1.));
#128150=DIRECTION('center_axis',(-1.,0.,0.));
#128151=DIRECTION('ref_axis',(0.,0.,1.));
#128152=DIRECTION('center_axis',(-1.,0.,0.));
#128153=DIRECTION('ref_axis',(0.,0.,1.));
#128154=DIRECTION('center_axis',(-1.,0.,0.));
#128155=DIRECTION('ref_axis',(0.,0.,1.));
#128156=DIRECTION('center_axis',(-1.,0.,0.));
#128157=DIRECTION('ref_axis',(0.,0.,1.));
#128158=DIRECTION('center_axis',(-1.,0.,0.));
#128159=DIRECTION('ref_axis',(0.,0.,1.));
#128160=DIRECTION('center_axis',(-1.,0.,0.));
#128161=DIRECTION('ref_axis',(0.,0.,1.));
#128162=DIRECTION('center_axis',(-1.,0.,0.));
#128163=DIRECTION('ref_axis',(0.,0.,1.));
#128164=DIRECTION('center_axis',(-1.,0.,0.));
#128165=DIRECTION('ref_axis',(0.,0.,1.));
#128166=DIRECTION('center_axis',(-1.,0.,0.));
#128167=DIRECTION('ref_axis',(0.,0.,1.));
#128168=DIRECTION('center_axis',(-1.,0.,0.));
#128169=DIRECTION('ref_axis',(0.,0.,1.));
#128170=DIRECTION('center_axis',(-1.,0.,0.));
#128171=DIRECTION('ref_axis',(0.,0.,1.));
#128172=DIRECTION('center_axis',(-1.,0.,0.));
#128173=DIRECTION('ref_axis',(0.,0.,1.));
#128174=DIRECTION('center_axis',(-1.,0.,0.));
#128175=DIRECTION('ref_axis',(0.,0.,1.));
#128176=DIRECTION('center_axis',(-1.,0.,0.));
#128177=DIRECTION('ref_axis',(0.,0.,1.));
#128178=DIRECTION('center_axis',(-1.,0.,0.));
#128179=DIRECTION('ref_axis',(0.,0.,1.));
#128180=DIRECTION('center_axis',(-1.,0.,0.));
#128181=DIRECTION('ref_axis',(0.,0.,1.));
#128182=DIRECTION('center_axis',(-1.,0.,0.));
#128183=DIRECTION('ref_axis',(0.,0.,1.));
#128184=DIRECTION('center_axis',(-1.,0.,0.));
#128185=DIRECTION('ref_axis',(0.,0.,1.));
#128186=DIRECTION('center_axis',(-1.,0.,0.));
#128187=DIRECTION('ref_axis',(0.,0.,1.));
#128188=DIRECTION('center_axis',(-1.,0.,0.));
#128189=DIRECTION('ref_axis',(0.,0.,1.));
#128190=DIRECTION('center_axis',(-1.,0.,0.));
#128191=DIRECTION('ref_axis',(0.,0.,1.));
#128192=DIRECTION('center_axis',(-1.,0.,0.));
#128193=DIRECTION('ref_axis',(0.,0.,1.));
#128194=DIRECTION('center_axis',(-1.,0.,0.));
#128195=DIRECTION('ref_axis',(0.,0.,1.));
#128196=DIRECTION('center_axis',(-1.,0.,0.));
#128197=DIRECTION('ref_axis',(0.,0.,1.));
#128198=DIRECTION('',(1.,0.,0.));
#128199=DIRECTION('center_axis',(-1.,0.,0.));
#128200=DIRECTION('ref_axis',(0.,0.,1.));
#128201=DIRECTION('',(-1.,0.,0.));
#128202=DIRECTION('center_axis',(-1.,0.,0.));
#128203=DIRECTION('ref_axis',(0.,0.,1.));
#128204=DIRECTION('',(-1.,0.,0.));
#128205=DIRECTION('',(1.,0.,0.));
#128206=DIRECTION('center_axis',(-1.,0.,0.));
#128207=DIRECTION('ref_axis',(0.,0.,1.));
#128208=DIRECTION('center_axis',(-1.,0.,0.));
#128209=DIRECTION('ref_axis',(0.,0.,1.));
#128210=DIRECTION('',(-1.,0.,0.));
#128211=DIRECTION('',(1.,0.,0.));
#128212=DIRECTION('center_axis',(-1.,0.,0.));
#128213=DIRECTION('ref_axis',(0.,0.,1.));
#128214=DIRECTION('center_axis',(-1.,0.,0.));
#128215=DIRECTION('ref_axis',(0.,0.,1.));
#128216=DIRECTION('',(-1.,0.,0.));
#128217=DIRECTION('',(1.,0.,0.));
#128218=DIRECTION('center_axis',(-1.,0.,0.));
#128219=DIRECTION('ref_axis',(0.,0.,1.));
#128220=DIRECTION('center_axis',(-1.,0.,0.));
#128221=DIRECTION('ref_axis',(0.,0.,1.));
#128222=DIRECTION('',(1.,0.,0.));
#128223=DIRECTION('center_axis',(-1.,0.,0.));
#128224=DIRECTION('ref_axis',(0.,0.,1.));
#128225=DIRECTION('',(-1.,0.,0.));
#128226=DIRECTION('center_axis',(-1.,0.,0.));
#128227=DIRECTION('ref_axis',(0.,0.,1.));
#128228=DIRECTION('',(1.,0.,0.));
#128229=DIRECTION('center_axis',(-1.,0.,0.));
#128230=DIRECTION('ref_axis',(0.,0.,1.));
#128231=DIRECTION('center_axis',(-1.,0.,0.));
#128232=DIRECTION('ref_axis',(0.,0.,1.));
#128233=DIRECTION('',(-1.,0.,0.));
#128234=DIRECTION('',(1.,0.,0.));
#128235=DIRECTION('center_axis',(-1.,0.,0.));
#128236=DIRECTION('ref_axis',(0.,0.,1.));
#128237=DIRECTION('center_axis',(-1.,0.,0.));
#128238=DIRECTION('ref_axis',(0.,0.,1.));
#128239=DIRECTION('',(1.,0.,0.));
#128240=DIRECTION('center_axis',(-1.,0.,0.));
#128241=DIRECTION('ref_axis',(0.,0.,1.));
#128242=DIRECTION('',(-1.,0.,0.));
#128243=DIRECTION('center_axis',(-1.,0.,0.));
#128244=DIRECTION('ref_axis',(0.,0.,1.));
#128245=DIRECTION('',(-1.,0.,0.));
#128246=DIRECTION('',(1.,0.,0.));
#128247=DIRECTION('center_axis',(-1.,0.,0.));
#128248=DIRECTION('ref_axis',(0.,0.,1.));
#128249=DIRECTION('center_axis',(-1.,0.,0.));
#128250=DIRECTION('ref_axis',(0.,0.,1.));
#128251=DIRECTION('',(-1.,0.,0.));
#128252=DIRECTION('center_axis',(-1.,0.,0.));
#128253=DIRECTION('ref_axis',(0.,0.,1.));
#128254=DIRECTION('center_axis',(-1.,0.,0.));
#128255=DIRECTION('ref_axis',(0.,0.,1.));
#128256=DIRECTION('',(1.,0.,0.));
#128257=DIRECTION('center_axis',(-1.,0.,0.));
#128258=DIRECTION('ref_axis',(0.,0.,1.));
#128259=DIRECTION('',(-1.,0.,0.));
#128260=DIRECTION('center_axis',(-1.,0.,0.));
#128261=DIRECTION('ref_axis',(0.,0.,1.));
#128262=DIRECTION('',(-1.,0.,0.));
#128263=DIRECTION('',(1.,0.,0.));
#128264=DIRECTION('center_axis',(-1.,0.,0.));
#128265=DIRECTION('ref_axis',(0.,0.,1.));
#128266=DIRECTION('center_axis',(-1.,0.,0.));
#128267=DIRECTION('ref_axis',(0.,0.,1.));
#128268=DIRECTION('',(1.,0.,0.));
#128269=DIRECTION('center_axis',(-1.,0.,0.));
#128270=DIRECTION('ref_axis',(0.,0.,1.));
#128271=DIRECTION('',(-1.,0.,0.));
#128272=DIRECTION('center_axis',(-1.,0.,0.));
#128273=DIRECTION('ref_axis',(0.,0.,1.));
#128274=DIRECTION('',(-1.,0.,0.));
#128275=DIRECTION('',(1.,0.,0.));
#128276=DIRECTION('center_axis',(-1.,0.,0.));
#128277=DIRECTION('ref_axis',(0.,0.,1.));
#128278=DIRECTION('center_axis',(-1.,0.,0.));
#128279=DIRECTION('ref_axis',(0.,9.64749793678664E-15,-1.));
#128280=DIRECTION('',(1.,0.,0.));
#128281=DIRECTION('center_axis',(-1.,0.,0.));
#128282=DIRECTION('ref_axis',(0.,0.,1.));
#128283=DIRECTION('',(-1.,0.,0.));
#128284=DIRECTION('center_axis',(-1.,0.,0.));
#128285=DIRECTION('ref_axis',(0.,0.,1.));
#128286=DIRECTION('',(-1.,0.,0.));
#128287=DIRECTION('',(1.,0.,0.));
#128288=DIRECTION('center_axis',(-1.,0.,0.));
#128289=DIRECTION('ref_axis',(0.,0.,1.));
#128290=DIRECTION('center_axis',(-1.,0.,0.));
#128291=DIRECTION('ref_axis',(0.,0.,1.));
#128292=DIRECTION('',(-1.,0.,0.));
#128293=DIRECTION('',(1.,0.,0.));
#128294=DIRECTION('center_axis',(-1.,0.,0.));
#128295=DIRECTION('ref_axis',(0.,0.,1.));
#128296=DIRECTION('center_axis',(-1.,0.,0.));
#128297=DIRECTION('ref_axis',(0.,0.,1.));
#128298=DIRECTION('',(1.,0.,0.));
#128299=DIRECTION('center_axis',(-1.,0.,0.));
#128300=DIRECTION('ref_axis',(0.,0.,1.));
#128301=DIRECTION('',(-1.,0.,0.));
#128302=DIRECTION('center_axis',(-1.,0.,0.));
#128303=DIRECTION('ref_axis',(0.,0.,1.));
#128304=DIRECTION('',(-1.,0.,0.));
#128305=DIRECTION('',(1.,0.,0.));
#128306=DIRECTION('center_axis',(-1.,0.,0.));
#128307=DIRECTION('ref_axis',(0.,0.,1.));
#128308=DIRECTION('center_axis',(-1.,0.,0.));
#128309=DIRECTION('ref_axis',(0.,0.,1.));
#128310=DIRECTION('',(1.,0.,0.));
#128311=DIRECTION('center_axis',(-1.,0.,0.));
#128312=DIRECTION('ref_axis',(0.,0.,1.));
#128313=DIRECTION('',(-1.,0.,0.));
#128314=DIRECTION('center_axis',(-1.,0.,0.));
#128315=DIRECTION('ref_axis',(0.,0.,1.));
#128316=DIRECTION('',(-1.,0.,0.));
#128317=DIRECTION('',(1.,0.,0.));
#128318=DIRECTION('center_axis',(-1.,0.,0.));
#128319=DIRECTION('ref_axis',(0.,0.,1.));
#128320=DIRECTION('center_axis',(-1.,0.,0.));
#128321=DIRECTION('ref_axis',(0.,0.,1.));
#128322=DIRECTION('',(1.,0.,0.));
#128323=DIRECTION('center_axis',(-1.,0.,0.));
#128324=DIRECTION('ref_axis',(0.,0.,1.));
#128325=DIRECTION('',(-1.,0.,0.));
#128326=DIRECTION('center_axis',(-1.,0.,0.));
#128327=DIRECTION('ref_axis',(0.,0.,1.));
#128328=DIRECTION('',(-1.,0.,0.));
#128329=DIRECTION('',(1.,0.,0.));
#128330=DIRECTION('center_axis',(-1.,0.,0.));
#128331=DIRECTION('ref_axis',(0.,0.,1.));
#128332=DIRECTION('center_axis',(-1.,0.,0.));
#128333=DIRECTION('ref_axis',(0.,0.,1.));
#128334=DIRECTION('',(-1.,0.,0.));
#128335=DIRECTION('',(1.,0.,0.));
#128336=DIRECTION('center_axis',(-1.,0.,0.));
#128337=DIRECTION('ref_axis',(0.,0.,1.));
#128338=DIRECTION('center_axis',(-1.,0.,0.));
#128339=DIRECTION('ref_axis',(0.,0.,1.));
#128340=DIRECTION('',(1.,0.,0.));
#128341=DIRECTION('center_axis',(-1.,0.,0.));
#128342=DIRECTION('ref_axis',(0.,0.,1.));
#128343=DIRECTION('',(-1.,0.,0.));
#128344=DIRECTION('center_axis',(-1.,0.,0.));
#128345=DIRECTION('ref_axis',(0.,0.,1.));
#128346=DIRECTION('',(1.,0.,0.));
#128347=DIRECTION('center_axis',(-1.,0.,0.));
#128348=DIRECTION('ref_axis',(0.,0.,1.));
#128349=DIRECTION('',(-1.,0.,0.));
#128350=DIRECTION('center_axis',(-1.,0.,0.));
#128351=DIRECTION('ref_axis',(0.,0.,1.));
#128352=DIRECTION('',(-1.,0.,0.));
#128353=DIRECTION('',(1.,0.,0.));
#128354=DIRECTION('center_axis',(-1.,0.,0.));
#128355=DIRECTION('ref_axis',(0.,0.,1.));
#128356=DIRECTION('center_axis',(-1.,0.,0.));
#128357=DIRECTION('ref_axis',(0.,0.,1.));
#128358=DIRECTION('',(-1.,0.,0.));
#128359=DIRECTION('',(1.,0.,0.));
#128360=DIRECTION('center_axis',(-1.,0.,0.));
#128361=DIRECTION('ref_axis',(0.,0.,1.));
#128362=DIRECTION('center_axis',(-1.,0.,0.));
#128363=DIRECTION('ref_axis',(0.,0.,1.));
#128364=DIRECTION('center_axis',(-1.,0.,0.));
#128365=DIRECTION('ref_axis',(0.,0.,1.));
#128366=DIRECTION('center_axis',(-1.,0.,0.));
#128367=DIRECTION('ref_axis',(0.,0.,1.));
#128368=DIRECTION('center_axis',(-1.,0.,0.));
#128369=DIRECTION('ref_axis',(0.,0.,1.));
#128370=DIRECTION('center_axis',(-1.,0.,0.));
#128371=DIRECTION('ref_axis',(0.,0.,1.));
#128372=DIRECTION('center_axis',(-1.,0.,0.));
#128373=DIRECTION('ref_axis',(0.,0.,1.));
#128374=DIRECTION('center_axis',(-1.,0.,0.));
#128375=DIRECTION('ref_axis',(0.,0.,1.));
#128376=DIRECTION('center_axis',(-1.,0.,0.));
#128377=DIRECTION('ref_axis',(0.,0.,1.));
#128378=DIRECTION('center_axis',(-1.,0.,0.));
#128379=DIRECTION('ref_axis',(0.,0.,1.));
#128380=DIRECTION('center_axis',(-1.,0.,0.));
#128381=DIRECTION('ref_axis',(0.,0.,1.));
#128382=DIRECTION('center_axis',(-1.,0.,0.));
#128383=DIRECTION('ref_axis',(0.,0.,1.));
#128384=DIRECTION('center_axis',(-1.,0.,0.));
#128385=DIRECTION('ref_axis',(0.,0.,1.));
#128386=DIRECTION('center_axis',(-1.,0.,0.));
#128387=DIRECTION('ref_axis',(0.,0.,1.));
#128388=DIRECTION('center_axis',(-1.,0.,0.));
#128389=DIRECTION('ref_axis',(0.,0.,1.));
#128390=DIRECTION('center_axis',(-1.,0.,0.));
#128391=DIRECTION('ref_axis',(0.,0.,1.));
#128392=DIRECTION('center_axis',(-1.,0.,0.));
#128393=DIRECTION('ref_axis',(0.,0.,1.));
#128394=DIRECTION('center_axis',(-1.,0.,0.));
#128395=DIRECTION('ref_axis',(0.,0.,1.));
#128396=DIRECTION('center_axis',(-1.,0.,0.));
#128397=DIRECTION('ref_axis',(0.,0.,1.));
#128398=DIRECTION('center_axis',(-1.,0.,0.));
#128399=DIRECTION('ref_axis',(0.,0.,1.));
#128400=DIRECTION('center_axis',(-1.,0.,0.));
#128401=DIRECTION('ref_axis',(0.,0.,1.));
#128402=DIRECTION('center_axis',(-1.,0.,0.));
#128403=DIRECTION('ref_axis',(0.,0.,1.));
#128404=DIRECTION('center_axis',(-1.,0.,0.));
#128405=DIRECTION('ref_axis',(0.,0.,1.));
#128406=DIRECTION('center_axis',(-1.,0.,0.));
#128407=DIRECTION('ref_axis',(0.,0.,1.));
#128408=DIRECTION('center_axis',(-1.,0.,0.));
#128409=DIRECTION('ref_axis',(0.,0.,1.));
#128410=DIRECTION('center_axis',(-1.,0.,0.));
#128411=DIRECTION('ref_axis',(0.,0.,1.));
#128412=DIRECTION('center_axis',(-1.,0.,0.));
#128413=DIRECTION('ref_axis',(0.,0.,1.));
#128414=DIRECTION('center_axis',(-1.,0.,0.));
#128415=DIRECTION('ref_axis',(0.,0.,1.));
#128416=DIRECTION('center_axis',(-1.,0.,0.));
#128417=DIRECTION('ref_axis',(0.,0.,1.));
#128418=DIRECTION('center_axis',(-1.,0.,0.));
#128419=DIRECTION('ref_axis',(0.,1.05802772004469E-14,-1.));
#128420=DIRECTION('center_axis',(-1.,0.,0.));
#128421=DIRECTION('ref_axis',(0.,0.,1.));
#128422=DIRECTION('center_axis',(-1.,0.,0.));
#128423=DIRECTION('ref_axis',(0.,0.,1.));
#128424=DIRECTION('center_axis',(-1.,0.,0.));
#128425=DIRECTION('ref_axis',(0.,0.,1.));
#128426=DIRECTION('center_axis',(-1.,0.,0.));
#128427=DIRECTION('ref_axis',(0.,0.,1.));
#128428=DIRECTION('center_axis',(-1.,0.,0.));
#128429=DIRECTION('ref_axis',(0.,0.,1.));
#128430=DIRECTION('center_axis',(-1.,0.,0.));
#128431=DIRECTION('ref_axis',(0.,0.,1.));
#128432=DIRECTION('center_axis',(-1.,0.,0.));
#128433=DIRECTION('ref_axis',(0.,0.,1.));
#128434=DIRECTION('center_axis',(-1.,0.,0.));
#128435=DIRECTION('ref_axis',(0.,0.,1.));
#128436=DIRECTION('center_axis',(-1.,0.,0.));
#128437=DIRECTION('ref_axis',(0.,0.,1.));
#128438=DIRECTION('center_axis',(-1.,0.,0.));
#128439=DIRECTION('ref_axis',(0.,0.,1.));
#128440=DIRECTION('center_axis',(-1.,0.,0.));
#128441=DIRECTION('ref_axis',(0.,0.,1.));
#128442=DIRECTION('center_axis',(-1.,0.,0.));
#128443=DIRECTION('ref_axis',(0.,0.,1.));
#128444=DIRECTION('center_axis',(-1.,0.,0.));
#128445=DIRECTION('ref_axis',(0.,0.,1.));
#128446=DIRECTION('center_axis',(-1.,0.,0.));
#128447=DIRECTION('ref_axis',(0.,0.,1.));
#128448=DIRECTION('center_axis',(-1.,0.,0.));
#128449=DIRECTION('ref_axis',(0.,0.,1.));
#128450=DIRECTION('center_axis',(-1.,0.,0.));
#128451=DIRECTION('ref_axis',(0.,0.,1.));
#128452=DIRECTION('center_axis',(-1.,0.,0.));
#128453=DIRECTION('ref_axis',(0.,0.,1.));
#128454=DIRECTION('center_axis',(-1.,0.,0.));
#128455=DIRECTION('ref_axis',(0.,0.,1.));
#128456=DIRECTION('center_axis',(-1.,0.,0.));
#128457=DIRECTION('ref_axis',(0.,0.,1.));
#128458=DIRECTION('center_axis',(-1.,0.,0.));
#128459=DIRECTION('ref_axis',(0.,0.,1.));
#128460=DIRECTION('center_axis',(-1.,0.,0.));
#128461=DIRECTION('ref_axis',(0.,0.,1.));
#128462=DIRECTION('center_axis',(-1.,0.,0.));
#128463=DIRECTION('ref_axis',(0.,0.,1.));
#128464=DIRECTION('center_axis',(-1.,0.,0.));
#128465=DIRECTION('ref_axis',(0.,0.,1.));
#128466=DIRECTION('center_axis',(-1.,0.,0.));
#128467=DIRECTION('ref_axis',(0.,0.,1.));
#128468=DIRECTION('center_axis',(-1.,0.,0.));
#128469=DIRECTION('ref_axis',(0.,0.,1.));
#128470=DIRECTION('center_axis',(-1.,0.,0.));
#128471=DIRECTION('ref_axis',(0.,0.,1.));
#128472=DIRECTION('center_axis',(-1.,0.,0.));
#128473=DIRECTION('ref_axis',(0.,0.,1.));
#128474=DIRECTION('center_axis',(-1.,0.,0.));
#128475=DIRECTION('ref_axis',(0.,0.,1.));
#128476=DIRECTION('center_axis',(-1.,0.,0.));
#128477=DIRECTION('ref_axis',(0.,0.,1.));
#128478=DIRECTION('center_axis',(-1.,0.,0.));
#128479=DIRECTION('ref_axis',(0.,0.,1.));
#128480=DIRECTION('',(-1.,0.,0.));
#128481=DIRECTION('',(1.,0.,0.));
#128482=DIRECTION('center_axis',(-1.,0.,0.));
#128483=DIRECTION('ref_axis',(0.,0.,1.));
#128484=DIRECTION('center_axis',(-1.,0.,0.));
#128485=DIRECTION('ref_axis',(0.,0.,1.));
#128486=DIRECTION('center_axis',(-1.,0.,0.));
#128487=DIRECTION('ref_axis',(0.,0.,1.));
#128488=DIRECTION('center_axis',(1.,0.,0.));
#128489=DIRECTION('ref_axis',(0.,0.,-1.));
#128490=DIRECTION('center_axis',(-1.,0.,0.));
#128491=DIRECTION('ref_axis',(0.,-3.090226693085E-15,-1.));
#128492=DIRECTION('center_axis',(-1.,0.,0.));
#128493=DIRECTION('ref_axis',(0.,-7.21052895053167E-15,-1.));
#128494=DIRECTION('center_axis',(-1.,0.,0.));
#128495=DIRECTION('ref_axis',(0.,3.54088475249323E-15,-1.));
#128496=DIRECTION('center_axis',(-1.,0.,0.));
#128497=DIRECTION('ref_axis',(0.,0.,-1.));
#128498=DIRECTION('center_axis',(-1.,0.,0.));
#128499=DIRECTION('ref_axis',(0.,0.,-1.));
#128500=DIRECTION('center_axis',(-1.,0.,0.));
#128501=DIRECTION('ref_axis',(0.,0.,-1.));
#128502=DIRECTION('center_axis',(-1.,0.,0.));
#128503=DIRECTION('ref_axis',(0.,0.,-1.));
#128504=DIRECTION('center_axis',(-1.,0.,0.));
#128505=DIRECTION('ref_axis',(0.,0.,-1.));
#128506=DIRECTION('center_axis',(-1.,0.,0.));
#128507=DIRECTION('ref_axis',(0.,0.,-1.));
#128508=DIRECTION('center_axis',(-1.,0.,0.));
#128509=DIRECTION('ref_axis',(0.,0.,-1.));
#128510=DIRECTION('center_axis',(-1.,0.,0.));
#128511=DIRECTION('ref_axis',(0.,4.12030225744667E-15,-1.));
#128512=DIRECTION('center_axis',(-1.,0.,0.));
#128513=DIRECTION('ref_axis',(0.,0.,-1.));
#128514=DIRECTION('center_axis',(-1.,0.,0.));
#128515=DIRECTION('ref_axis',(0.,8.24060451489334E-15,-1.));
#128516=DIRECTION('center_axis',(-1.,0.,0.));
#128517=DIRECTION('ref_axis',(0.,0.,-1.));
#128518=DIRECTION('center_axis',(-1.,0.,0.));
#128519=DIRECTION('ref_axis',(0.,2.06015112872333E-15,-1.));
#128520=DIRECTION('center_axis',(-1.,0.,0.));
#128521=DIRECTION('ref_axis',(0.,-4.12030225744667E-15,-1.));
#128522=DIRECTION('center_axis',(-1.,0.,0.));
#128523=DIRECTION('ref_axis',(0.,4.12030225744667E-15,-1.));
#128524=DIRECTION('center_axis',(-1.,0.,0.));
#128525=DIRECTION('ref_axis',(0.,4.12030225744667E-15,-1.));
#128526=DIRECTION('center_axis',(-1.,0.,0.));
#128527=DIRECTION('ref_axis',(0.,0.,1.));
#128528=DIRECTION('',(-1.,0.,0.));
#128529=DIRECTION('center_axis',(-1.,0.,0.));
#128530=DIRECTION('ref_axis',(0.,0.,1.));
#128531=DIRECTION('',(-1.,0.,0.));
#128532=DIRECTION('center_axis',(-1.,0.,0.));
#128533=DIRECTION('ref_axis',(0.,0.,1.));
#128534=DIRECTION('center_axis',(-1.,0.,0.));
#128535=DIRECTION('ref_axis',(0.,0.,1.));
#128536=DIRECTION('',(-1.,0.,0.));
#128537=DIRECTION('center_axis',(-1.,0.,0.));
#128538=DIRECTION('ref_axis',(0.,0.,1.));
#128539=DIRECTION('',(-1.,0.,0.));
#128540=DIRECTION('center_axis',(-1.,0.,0.));
#128541=DIRECTION('ref_axis',(0.,0.,1.));
#128542=DIRECTION('center_axis',(-1.,0.,0.));
#128543=DIRECTION('ref_axis',(0.,0.,1.));
#128544=DIRECTION('center_axis',(-1.,0.,0.));
#128545=DIRECTION('ref_axis',(0.,0.,1.));
#128546=DIRECTION('center_axis',(-1.,0.,0.));
#128547=DIRECTION('ref_axis',(0.,0.,1.));
#128548=DIRECTION('center_axis',(-1.,0.,0.));
#128549=DIRECTION('ref_axis',(0.,0.,1.));
#128550=DIRECTION('center_axis',(-1.,0.,0.));
#128551=DIRECTION('ref_axis',(0.,0.,1.));
#128552=DIRECTION('center_axis',(-1.,0.,0.));
#128553=DIRECTION('ref_axis',(0.,0.,1.));
#128554=DIRECTION('center_axis',(-1.,0.,0.));
#128555=DIRECTION('ref_axis',(0.,0.,1.));
#128556=DIRECTION('',(-1.,0.,0.));
#128557=DIRECTION('center_axis',(-1.,0.,0.));
#128558=DIRECTION('ref_axis',(0.,0.,1.));
#128559=DIRECTION('',(-1.,0.,0.));
#128560=DIRECTION('center_axis',(-1.,0.,0.));
#128561=DIRECTION('ref_axis',(0.,0.,1.));
#128562=DIRECTION('center_axis',(-1.,0.,0.));
#128563=DIRECTION('ref_axis',(0.,0.0500387861363127,-0.998747275281392));
#128564=DIRECTION('center_axis',(-1.,0.,0.));
#128565=DIRECTION('ref_axis',(0.,0.,1.));
#128566=DIRECTION('center_axis',(-1.,0.,0.));
#128567=DIRECTION('ref_axis',(0.,0.,1.));
#128568=DIRECTION('center_axis',(-1.,0.,0.));
#128569=DIRECTION('ref_axis',(0.,0.,1.));
#128570=DIRECTION('center_axis',(-1.,0.,0.));
#128571=DIRECTION('ref_axis',(0.,0.,1.));
#128572=DIRECTION('center_axis',(-1.,0.,0.));
#128573=DIRECTION('ref_axis',(0.,0.,1.));
#128574=DIRECTION('center_axis',(-1.,0.,0.));
#128575=DIRECTION('ref_axis',(0.,0.,1.));
#128576=DIRECTION('',(-1.,0.,0.));
#128577=DIRECTION('center_axis',(-1.,0.,0.));
#128578=DIRECTION('ref_axis',(0.,0.,1.));
#128579=DIRECTION('',(-1.,0.,0.));
#128580=DIRECTION('center_axis',(-1.,0.,0.));
#128581=DIRECTION('ref_axis',(0.,0.,1.));
#128582=DIRECTION('center_axis',(-1.,0.,0.));
#128583=DIRECTION('ref_axis',(0.,0.,1.));
#128584=DIRECTION('center_axis',(-1.,0.,0.));
#128585=DIRECTION('ref_axis',(0.,0.,1.));
#128586=DIRECTION('center_axis',(-1.,0.,0.));
#128587=DIRECTION('ref_axis',(0.,0.,1.));
#128588=DIRECTION('center_axis',(-1.,0.,0.));
#128589=DIRECTION('ref_axis',(0.,-0.0500387861362921,-0.998747275281393));
#128590=DIRECTION('center_axis',(-1.,0.,0.));
#128591=DIRECTION('ref_axis',(0.,0.,1.));
#128592=DIRECTION('center_axis',(-1.,0.,0.));
#128593=DIRECTION('ref_axis',(0.,0.,1.));
#128594=DIRECTION('center_axis',(-1.,0.,0.));
#128595=DIRECTION('ref_axis',(0.,0.,1.));
#128596=DIRECTION('center_axis',(-1.,0.,0.));
#128597=DIRECTION('ref_axis',(0.,0.,1.));
#128598=DIRECTION('center_axis',(-1.,0.,0.));
#128599=DIRECTION('ref_axis',(0.,0.,1.));
#128600=DIRECTION('center_axis',(-1.,0.,0.));
#128601=DIRECTION('ref_axis',(0.,0.,1.));
#128602=DIRECTION('center_axis',(-1.,0.,0.));
#128603=DIRECTION('ref_axis',(0.,0.,1.));
#128604=DIRECTION('center_axis',(-1.,0.,0.));
#128605=DIRECTION('ref_axis',(0.,0.,1.));
#128606=DIRECTION('center_axis',(-1.,0.,0.));
#128607=DIRECTION('ref_axis',(0.,0.,1.));
#128608=DIRECTION('',(-1.,0.,0.));
#128609=DIRECTION('center_axis',(-1.,0.,0.));
#128610=DIRECTION('ref_axis',(0.,0.,1.));
#128611=DIRECTION('',(-1.,0.,0.));
#128612=DIRECTION('center_axis',(-1.,0.,0.));
#128613=DIRECTION('ref_axis',(0.,0.309016994374949,-0.951056516295153));
#128614=DIRECTION('center_axis',(-1.,0.,0.));
#128615=DIRECTION('ref_axis',(0.,0.,1.));
#128616=DIRECTION('',(-1.,0.,0.));
#128617=DIRECTION('center_axis',(-1.,0.,0.));
#128618=DIRECTION('ref_axis',(0.,0.,1.));
#128619=DIRECTION('',(-1.,0.,0.));
#128620=DIRECTION('center_axis',(-1.,0.,0.));
#128621=DIRECTION('ref_axis',(0.,0.669130606358861,-0.743144825477392));
#128622=DIRECTION('center_axis',(-1.,0.,0.));
#128623=DIRECTION('ref_axis',(0.,0.,1.));
#128624=DIRECTION('',(-1.,0.,0.));
#128625=DIRECTION('center_axis',(-1.,0.,0.));
#128626=DIRECTION('ref_axis',(0.,0.,1.));
#128627=DIRECTION('',(-1.,0.,0.));
#128628=DIRECTION('center_axis',(-1.,0.,0.));
#128629=DIRECTION('ref_axis',(0.,0.500000000000004,-0.866025403784436));
#128630=DIRECTION('center_axis',(-1.,0.,0.));
#128631=DIRECTION('ref_axis',(0.,0.,1.));
#128632=DIRECTION('',(-1.,0.,0.));
#128633=DIRECTION('center_axis',(-1.,0.,0.));
#128634=DIRECTION('ref_axis',(0.,0.913545457642602,-0.406736643075798));
#128635=DIRECTION('center_axis',(-1.,0.,0.));
#128636=DIRECTION('ref_axis',(0.,0.,1.));
#128637=DIRECTION('',(-1.,0.,0.));
#128638=DIRECTION('center_axis',(-1.,0.,0.));
#128639=DIRECTION('ref_axis',(0.,0.,1.));
#128640=DIRECTION('',(-1.,0.,0.));
#128641=DIRECTION('center_axis',(-1.,0.,0.));
#128642=DIRECTION('ref_axis',(0.,0.809016994374951,-0.587785252292468));
#128643=DIRECTION('center_axis',(-1.,0.,0.));
#128644=DIRECTION('ref_axis',(0.,0.,1.));
#128645=DIRECTION('',(-1.,0.,0.));
#128646=DIRECTION('center_axis',(-1.,0.,0.));
#128647=DIRECTION('ref_axis',(0.,0.,1.));
#128648=DIRECTION('',(-1.,0.,0.));
#128649=DIRECTION('center_axis',(-1.,0.,0.));
#128650=DIRECTION('ref_axis',(0.,0.,1.));
#128651=DIRECTION('center_axis',(-1.,0.,0.));
#128652=DIRECTION('ref_axis',(0.,0.,1.));
#128653=DIRECTION('',(-1.,0.,0.));
#128654=DIRECTION('center_axis',(-1.,0.,0.));
#128655=DIRECTION('ref_axis',(0.,0.,1.));
#128656=DIRECTION('',(-1.,0.,0.));
#128657=DIRECTION('center_axis',(-1.,0.,0.));
#128658=DIRECTION('ref_axis',(0.,0.,1.));
#128659=DIRECTION('center_axis',(-1.,0.,0.));
#128660=DIRECTION('ref_axis',(0.,0.,1.));
#128661=DIRECTION('',(-1.,0.,0.));
#128662=DIRECTION('center_axis',(-1.,0.,0.));
#128663=DIRECTION('ref_axis',(0.,0.,1.));
#128664=DIRECTION('',(-1.,0.,0.));
#128665=DIRECTION('center_axis',(-1.,0.,0.));
#128666=DIRECTION('ref_axis',(0.,-0.809016994374947,-0.587785252292473));
#128667=DIRECTION('center_axis',(-1.,0.,0.));
#128668=DIRECTION('ref_axis',(0.,0.,1.));
#128669=DIRECTION('',(-1.,0.,0.));
#128670=DIRECTION('center_axis',(-1.,0.,0.));
#128671=DIRECTION('ref_axis',(0.,0.,1.));
#128672=DIRECTION('',(-1.,0.,0.));
#128673=DIRECTION('center_axis',(-1.,0.,0.));
#128674=DIRECTION('ref_axis',(0.,-0.669130606358855,-0.743144825477397));
#128675=DIRECTION('center_axis',(-1.,0.,0.));
#128676=DIRECTION('ref_axis',(0.,0.,1.));
#128677=DIRECTION('',(-1.,0.,0.));
#128678=DIRECTION('center_axis',(-1.,0.,0.));
#128679=DIRECTION('ref_axis',(0.,-0.9135454576426,-0.406736643075802));
#128680=DIRECTION('center_axis',(-1.,0.,0.));
#128681=DIRECTION('ref_axis',(0.,0.,1.));
#128682=DIRECTION('',(-1.,0.,0.));
#128683=DIRECTION('center_axis',(-1.,0.,0.));
#128684=DIRECTION('ref_axis',(0.,0.,1.));
#128685=DIRECTION('',(-1.,0.,0.));
#128686=DIRECTION('center_axis',(-1.,0.,0.));
#128687=DIRECTION('ref_axis',(0.,-0.499999999999997,-0.866025403784441));
#128688=DIRECTION('center_axis',(-1.,0.,0.));
#128689=DIRECTION('ref_axis',(0.,0.,1.));
#128690=DIRECTION('',(-1.,0.,0.));
#128691=DIRECTION('center_axis',(-1.,0.,0.));
#128692=DIRECTION('ref_axis',(0.,0.,1.));
#128693=DIRECTION('',(-1.,0.,0.));
#128694=DIRECTION('center_axis',(-1.,0.,0.));
#128695=DIRECTION('ref_axis',(0.,-0.309016994374942,-0.951056516295155));
#128696=DIRECTION('center_axis',(-1.,0.,0.));
#128697=DIRECTION('ref_axis',(0.,0.,1.));
#128698=DIRECTION('',(-1.,0.,0.));
#128699=DIRECTION('center_axis',(-1.,0.,0.));
#128700=DIRECTION('ref_axis',(0.,0.,1.));
#128701=DIRECTION('',(-1.,0.,0.));
#128702=DIRECTION('center_axis',(-1.,0.,0.));
#128703=DIRECTION('ref_axis',(0.,-0.104528463267644,-0.994521895368274));
#128704=DIRECTION('center_axis',(-1.,0.,0.));
#128705=DIRECTION('ref_axis',(0.,0.,1.));
#128706=DIRECTION('',(-1.,0.,0.));
#128707=DIRECTION('center_axis',(-1.,0.,0.));
#128708=DIRECTION('ref_axis',(0.,0.,1.));
#128709=DIRECTION('',(-1.,0.,0.));
#128710=DIRECTION('center_axis',(-1.,0.,0.));
#128711=DIRECTION('ref_axis',(0.,0.104528463267661,-0.994521895368273));
#128712=DIRECTION('center_axis',(0.,-1.,0.));
#128713=DIRECTION('ref_axis',(0.,0.,-1.));
#128714=DIRECTION('',(-1.,0.,0.));
#128715=DIRECTION('',(-1.,0.,0.));
#128716=DIRECTION('center_axis',(0.,0.,1.));
#128717=DIRECTION('ref_axis',(1.,0.,0.));
#128718=DIRECTION('center_axis',(0.,0.,-1.));
#128719=DIRECTION('ref_axis',(-1.,0.,0.));
#272463=CARTESIAN_POINT('',(0.,0.,0.));
#272464=CARTESIAN_POINT('Origin',(4.42504848420342,-17.542318193471,0.972561099047131));
#272465=CARTESIAN_POINT('',(4.76104848420342,-17.542318193471,26.5085610990471));
#272466=CARTESIAN_POINT('Origin',(4.76104848420342,-17.542318193471,0.972561099047131));
#272467=CARTESIAN_POINT('',(4.42504848420342,-17.542318193471,26.1725610990471));
#272468=CARTESIAN_POINT('Origin',(4.42504848420342,-17.542318193471,26.5085610990471));
#272469=CARTESIAN_POINT('Origin',(4.42504848420342,-17.542318193471,0.972561099047131));
#272470=CARTESIAN_POINT('Origin',(-3.14818151579658,-17.542318193471,0.972561099047131));
#272471=CARTESIAN_POINT('',(-3.14818151579658,-17.542318193471,26.1725610990471));
#272472=CARTESIAN_POINT('',(-3.14818151579658,-17.542318193471,26.1725610990471));
#272473=CARTESIAN_POINT('Origin',(-3.14818151579658,-17.542318193471,0.972561099047131));
#272474=CARTESIAN_POINT('Origin',(11.5520284842034,30.3696711225593,-7.21027454921227));
#272475=CARTESIAN_POINT('',(11.5201159294504,29.2525234772273,18.3766132024512));
#272476=CARTESIAN_POINT('',(10.1651884842034,34.038690149408,18.1368188355985));
#272477=CARTESIAN_POINT('Ctrl Pts',(11.5201159294506,29.2525234772274,18.3766132024512));
#272478=CARTESIAN_POINT('Ctrl Pts',(11.5064953958128,29.4369831852153,18.3846668872306));
#272479=CARTESIAN_POINT('Ctrl Pts',(11.4885385348232,29.6214916739098,18.3907232698498));
#272480=CARTESIAN_POINT('Ctrl Pts',(11.2877548088084,31.2852685491064,18.427357082409));
#272481=CARTESIAN_POINT('Ctrl Pts',(10.8383054247332,32.7235821608133,18.3271821312736));
#272482=CARTESIAN_POINT('Ctrl Pts',(10.1651884842031,34.0386901494087,18.1368188355984));
#272483=CARTESIAN_POINT('',(6.14788848420341,34.038690149408,18.1368188355985));
#272484=CARTESIAN_POINT('',(8.15653848420341,34.038690149408,18.1368188355985));
#272485=CARTESIAN_POINT('',(4.79296103895619,29.2525234772273,18.3766132024512));
#272486=CARTESIAN_POINT('Ctrl Pts',(6.14788848420342,34.038690149408,18.1368188355985));
#272487=CARTESIAN_POINT('Ctrl Pts',(6.12358695752486,33.9912108334888,18.1436915176392));
#272488=CARTESIAN_POINT('Ctrl Pts',(6.099576183545,33.9435659759386,18.1504519561046));
#272489=CARTESIAN_POINT('Ctrl Pts',(5.43709796638902,32.6082554610184,18.3360613630301));
#272490=CARTESIAN_POINT('Ctrl Pts',(5.01156238585602,31.2076315268735,18.427677818826));
#272491=CARTESIAN_POINT('Ctrl Pts',(4.82218298524757,29.5970927300154,18.3899136899737));
#272492=CARTESIAN_POINT('Ctrl Pts',(4.80568122363092,29.4247899693517,18.3841345199289));
#272493=CARTESIAN_POINT('Ctrl Pts',(4.79296103895619,29.2525234772273,18.3766132024512));
#272494=CARTESIAN_POINT('',(11.5520284842034,29.2525234772273,18.3766132024512));
#272495=CARTESIAN_POINT('Origin',(11.5520284842034,-65.4543075095013,-7.2102745492126));
#272496=CARTESIAN_POINT('',(10.1651884842034,-69.1233265363501,18.1368188355982));
#272497=CARTESIAN_POINT('',(11.520115929451,-64.3371598641695,18.3766132024509));
#272498=CARTESIAN_POINT('Ctrl Pts',(10.1651884842034,-69.1233265363502,
18.1368188355982));
#272499=CARTESIAN_POINT('Ctrl Pts',(10.189490010882,-69.0758472204308,18.1436915176389));
#272500=CARTESIAN_POINT('Ctrl Pts',(10.2135007848619,-69.0282023628806,
18.1504519561043));
#272501=CARTESIAN_POINT('Ctrl Pts',(10.8759790020178,-67.6928918479604,
18.3360613630298));
#272502=CARTESIAN_POINT('Ctrl Pts',(11.3015145825508,-66.2922679138155,
18.4276778188257));
#272503=CARTESIAN_POINT('Ctrl Pts',(11.4908939831593,-64.6817291169574,
18.3899136899734));
#272504=CARTESIAN_POINT('Ctrl Pts',(11.5073957447759,-64.5094263562938,
18.3841345199286));
#272505=CARTESIAN_POINT('Ctrl Pts',(11.5201159294506,-64.3371598641694,
18.3766132024509));
#272506=CARTESIAN_POINT('',(4.79296103895619,-64.3371598641695,18.3766132024509));
#272507=CARTESIAN_POINT('',(11.5520284842034,-64.3371598641695,18.3766132024509));
#272508=CARTESIAN_POINT('',(6.14788848420341,-69.1233265363501,18.1368188355982));
#272509=CARTESIAN_POINT('Ctrl Pts',(4.79296103895619,-64.3371598641695,
18.3766132024509));
#272510=CARTESIAN_POINT('Ctrl Pts',(4.80658157259404,-64.5216195721574,
18.3846668872303));
#272511=CARTESIAN_POINT('Ctrl Pts',(4.8245384335836,-64.7061280608519,18.3907232698495));
#272512=CARTESIAN_POINT('Ctrl Pts',(5.02532215959842,-66.3699049360485,
18.4273570824086));
#272513=CARTESIAN_POINT('Ctrl Pts',(5.47477154367356,-67.8082185477554,
18.3271821312732));
#272514=CARTESIAN_POINT('Ctrl Pts',(6.14788848420374,-69.1233265363508,
18.1368188355981));
#272515=CARTESIAN_POINT('',(8.15653848420341,-69.1233265363501,18.1368188355982));
#272516=CARTESIAN_POINT('Origin',(11.5520284842034,-22.8798040147362,-49.8102242737207));
#272517=CARTESIAN_POINT('',(11.5520284842034,-19.9972458266101,-48.0680189924834));
#272518=CARTESIAN_POINT('',(11.5520284842034,-25.3371465446537,-47.5067728111188));
#272519=CARTESIAN_POINT('Origin',(11.5520284842034,-22.8798040147362,-49.8102242737207));
#272520=CARTESIAN_POINT('',(11.5201159294503,-25.8673877784838,-48.2549866055504));
#272521=CARTESIAN_POINT('Ctrl Pts',(11.5520284842034,-25.3371465446537,
-47.5067728111188));
#272522=CARTESIAN_POINT('Ctrl Pts',(11.5520284842034,-25.4218077136364,
-47.5970901000009));
#272523=CARTESIAN_POINT('Ctrl Pts',(11.5505455276579,-25.5014883801418,
-47.6920685179292));
#272524=CARTESIAN_POINT('Ctrl Pts',(11.5472515368861,-25.5758260890567,
-47.7913393065626));
#272525=CARTESIAN_POINT('Ctrl Pts',(11.5440442061753,-25.6482080819925,
-47.8879984264961));
#272526=CARTESIAN_POINT('Ctrl Pts',(11.539119436029,-25.7155242765753,-47.9887269871974));
#272527=CARTESIAN_POINT('Ctrl Pts',(11.532206799367,-25.7774102007914,-48.0931625380847));
#272528=CARTESIAN_POINT('Ctrl Pts',(11.5286984812716,-25.8088186948865,
-48.1461659217282));
#272529=CARTESIAN_POINT('Ctrl Pts',(11.5246786952113,-25.8388280077787,
-48.2001237964755));
#272530=CARTESIAN_POINT('Ctrl Pts',(11.5201159294506,-25.8673877784838,
-48.2549866055504));
#272531=CARTESIAN_POINT('',(4.79296103895619,-25.8673877784838,-48.2549866055504));
#272532=CARTESIAN_POINT('',(11.5520284842034,-25.8673877784838,-48.2549866055504));
#272533=CARTESIAN_POINT('',(4.76104848420342,-25.3371465446537,-47.5067728111188));
#272534=CARTESIAN_POINT('Ctrl Pts',(4.79296103895619,-25.8673877784838,
-48.2549866055504));
#272535=CARTESIAN_POINT('Ctrl Pts',(4.77035892158038,-25.725914092661,-47.9832181836481));
#272536=CARTESIAN_POINT('Ctrl Pts',(4.76104848420342,-25.5477399600458,
-47.7314357417538));
#272537=CARTESIAN_POINT('Ctrl Pts',(4.76104848420342,-25.3371465446537,
-47.5067728111189));
#272538=CARTESIAN_POINT('',(4.76104848420342,-19.9972458266101,-48.0680189924834));
#272539=CARTESIAN_POINT('Origin',(4.76104848420342,-22.8798040147362,-49.8102242737207));
#272540=CARTESIAN_POINT('',(4.79296103895619,-19.6341540310225,-48.9101258718094));
#272541=CARTESIAN_POINT('Ctrl Pts',(4.76104848420342,-19.9972458266101,
-48.0680189924834));
#272542=CARTESIAN_POINT('Ctrl Pts',(4.76104848420342,-19.933217960153,-48.1739560210942));
#272543=CARTESIAN_POINT('Ctrl Pts',(4.76253119975839,-19.8750297749198,
-48.2834165710042));
#272544=CARTESIAN_POINT('Ctrl Pts',(4.76582464685228,-19.8229591767546,
-48.3959644781904));
#272545=CARTESIAN_POINT('Ctrl Pts',(4.76903141935803,-19.7722589353985,
-48.505550429947));
#272546=CARTESIAN_POINT('Ctrl Pts',(4.773955313379,-19.7273587788838,-48.618063270801));
#272547=CARTESIAN_POINT('Ctrl Pts',(4.78086668106801,-19.6885398848474,
-48.7330726175708));
#272548=CARTESIAN_POINT('Ctrl Pts',(4.78437582490195,-19.6688301705364,
-48.7914668975778));
#272549=CARTESIAN_POINT('Ctrl Pts',(4.78839676418624,-19.6506885493468,
-48.8505043248586));
#272550=CARTESIAN_POINT('Ctrl Pts',(4.79296103895619,-19.6341540310225,
-48.9101258718095));
#272551=CARTESIAN_POINT('',(11.520115929451,-19.6341540310225,-48.9101258718094));
#272552=CARTESIAN_POINT('',(11.5520284842034,-19.6341540310225,-48.9101258718094));
#272553=CARTESIAN_POINT('Ctrl Pts',(11.5201159294506,-19.6341540310225,
-48.9101258718094));
#272554=CARTESIAN_POINT('Ctrl Pts',(11.5379482942249,-19.6987534640074,
-48.677187841734));
#272555=CARTESIAN_POINT('Ctrl Pts',(11.5475950755165,-19.7884941430255,
-48.4509138861737));
#272556=CARTESIAN_POINT('Ctrl Pts',(11.5516325551658,-19.9325572097809,
-48.1785764633217));
#272557=CARTESIAN_POINT('Ctrl Pts',(11.5520284842034,-19.9641379606009,
-48.1227974685242));
#272558=CARTESIAN_POINT('Ctrl Pts',(11.5520284842034,-19.9972458266101,
-48.0680189924834));
#272559=CARTESIAN_POINT('Origin',(11.5520284842034,-33.3215019147798,-47.5907728700904));
#272560=CARTESIAN_POINT('',(11.5520284842034,-30.139709693315,-46.4859565010363));
#272561=CARTESIAN_POINT('',(11.5520284842034,-35.2462311262936,-44.8267471082261));
#272562=CARTESIAN_POINT('Origin',(11.5520284842034,-33.3215019147798,-47.5907728700904));
#272563=CARTESIAN_POINT('',(11.5201159294502,-35.920447712068,-45.4483672846184));
#272564=CARTESIAN_POINT('Ctrl Pts',(11.5520284842034,-35.2462311262936,
-44.8267471082261));
#272565=CARTESIAN_POINT('Ctrl Pts',(11.5520284842034,-35.3478213939342,
-44.8974894864019));
#272566=CARTESIAN_POINT('Ctrl Pts',(11.5505454949267,-35.4455089937706,
-44.9738267449025));
#272567=CARTESIAN_POINT('Ctrl Pts',(11.5472514286393,-35.5388627267499,
-45.0554735553234));
#272568=CARTESIAN_POINT('Ctrl Pts',(11.5440440212189,-35.6297605502186,
-45.1349724368738));
#272569=CARTESIAN_POINT('Ctrl Pts',(11.539119130381,-35.7165492567715,-45.2195051912617));
#272570=CARTESIAN_POINT('Ctrl Pts',(11.5322063173366,-35.7987969833134,
-45.3087930763808));
#272571=CARTESIAN_POINT('Ctrl Pts',(11.5286981135764,-35.8405371232053,
-45.3541060469908));
#272572=CARTESIAN_POINT('Ctrl Pts',(11.5246784869469,-35.8811072172304,
-45.4006434481913));
#272573=CARTESIAN_POINT('Ctrl Pts',(11.5201159294506,-35.9204477120681,
-45.4483672846184));
#272574=CARTESIAN_POINT('',(4.79296103895619,-35.920447712068,-45.4483672846184));
#272575=CARTESIAN_POINT('',(11.5520284842034,-35.920447712068,-45.4483672846184));
#272576=CARTESIAN_POINT('',(4.76104848420342,-35.2462311262936,-44.8267471082261));
#272577=CARTESIAN_POINT('Ctrl Pts',(4.79296103895618,-35.920447712068,-45.4483672846184));
#272578=CARTESIAN_POINT('Ctrl Pts',(4.77035892158034,-35.7255617336046,
-45.2119516880047));
#272579=CARTESIAN_POINT('Ctrl Pts',(4.76104848420342,-35.4989326200616,
-45.002715781731));
#272580=CARTESIAN_POINT('Ctrl Pts',(4.76104848420342,-35.2462311262936,
-44.8267471082261));
#272581=CARTESIAN_POINT('',(4.76104848420342,-30.139709693315,-46.4859565010363));
#272582=CARTESIAN_POINT('Origin',(4.76104848420342,-33.3215019147798,-47.5907728700904));
#272583=CARTESIAN_POINT('',(4.79296103895619,-29.9596361897448,-47.3851523537532));
#272584=CARTESIAN_POINT('Ctrl Pts',(4.76104848420342,-30.139709693315,-46.4859565010363));
#272585=CARTESIAN_POINT('Ctrl Pts',(4.76104848420342,-30.0991044446722,
-46.6028967165337));
#272586=CARTESIAN_POINT('Ctrl Pts',(4.76253135162959,-30.0649445444981,
-46.7220693473933));
#272587=CARTESIAN_POINT('Ctrl Pts',(4.76582514301997,-30.0374111372492,
-46.8429900493133));
#272588=CARTESIAN_POINT('Ctrl Pts',(4.76903226819381,-30.0106021888235,
-46.9607290865517));
#272589=CARTESIAN_POINT('Ctrl Pts',(4.7739567160318,-29.990075838413,-47.080125258691));
#272590=CARTESIAN_POINT('Ctrl Pts',(4.78086888743444,-29.9760176360285,
-47.2006991758224));
#272591=CARTESIAN_POINT('Ctrl Pts',(4.78437750874215,-29.9688816861856,
-47.2619025502989));
#272592=CARTESIAN_POINT('Ctrl Pts',(4.78839771848159,-29.9634125828066,
-47.3234088729724));
#272593=CARTESIAN_POINT('Ctrl Pts',(4.79296103895619,-29.9596361897448,
-47.3851523537532));
#272594=CARTESIAN_POINT('',(11.520115929451,-29.9596361897448,-47.3851523537532));
#272595=CARTESIAN_POINT('',(11.5520284842034,-29.9596361897448,-47.3851523537532));
#272596=CARTESIAN_POINT('Ctrl Pts',(11.5201159294506,-29.9596361897448,
-47.3851523537531));
#272597=CARTESIAN_POINT('Ctrl Pts',(11.5379482942249,-29.974393430439,-47.1438736011772));
#272598=CARTESIAN_POINT('Ctrl Pts',(11.5475950755165,-30.0151280596203,
-46.9038861381276));
#272599=CARTESIAN_POINT('Ctrl Pts',(11.5516325551658,-30.0994208686632,
-46.6075475455815));
#272600=CARTESIAN_POINT('Ctrl Pts',(11.5520284842034,-30.1187143991867,
-46.5464214483487));
#272601=CARTESIAN_POINT('Ctrl Pts',(11.5520284842034,-30.139709693315,-46.4859565010363));
#272602=CARTESIAN_POINT('Origin',(11.5520284842034,-51.7098072425568,-36.9742798391576));
#272603=CARTESIAN_POINT('',(11.5520284842034,-48.3537261103108,-37.2591313508023));
#272604=CARTESIAN_POINT('',(11.5520284842034,-52.3439043111715,-33.6663587612783));
#272605=CARTESIAN_POINT('Origin',(11.5520284842034,-51.7098072425568,-36.9742798391576));
#272606=CARTESIAN_POINT('',(11.520115929451,-53.212667514387,-33.9600084589965));
#272607=CARTESIAN_POINT('Ctrl Pts',(11.5520284842034,-52.3439043111714,
-33.6663587612783));
#272608=CARTESIAN_POINT('Ctrl Pts',(11.5520284842034,-52.4654852159812,
-33.6896646665657));
#272609=CARTESIAN_POINT('Ctrl Pts',(11.5505454934861,-52.585776508724,-33.7196691161155));
#272610=CARTESIAN_POINT('Ctrl Pts',(11.5472514229146,-52.7042682136749,
-33.7562868369326));
#272611=CARTESIAN_POINT('Ctrl Pts',(11.5440440116043,-52.8196426801257,
-33.7919412315054));
#272612=CARTESIAN_POINT('Ctrl Pts',(11.5391191144802,-52.9333107492123,
-33.8338656362247));
#272613=CARTESIAN_POINT('Ctrl Pts',(11.5322062913588,-53.0447645176165,
-33.8819810649254));
#272614=CARTESIAN_POINT('Ctrl Pts',(11.5286980938785,-53.1013263336234,
-33.9063992256053));
#272615=CARTESIAN_POINT('Ctrl Pts',(11.5246784758733,-53.1573172853413,
-33.9324118527927));
#272616=CARTESIAN_POINT('Ctrl Pts',(11.5201159294506,-53.212667514387,-33.9600084589965));
#272617=CARTESIAN_POINT('',(4.79296103895619,-53.212667514387,-33.9600084589965));
#272618=CARTESIAN_POINT('',(11.5520284842034,-53.212667514387,-33.9600084589965));
#272619=CARTESIAN_POINT('',(4.76104848420342,-52.3439043111715,-33.6663587612783));
#272620=CARTESIAN_POINT('Ctrl Pts',(4.79296103895618,-53.212667514387,-33.9600084589965));
#272621=CARTESIAN_POINT('Ctrl Pts',(4.77035892157491,-52.9384714278002,
-33.8232993332241));
#272622=CARTESIAN_POINT('Ctrl Pts',(4.76104848420342,-52.6463315204171,
-33.7243311863565));
#272623=CARTESIAN_POINT('Ctrl Pts',(4.76104848420342,-52.3439043111715,
-33.6663587612783));
#272624=CARTESIAN_POINT('',(4.76104848420342,-48.3537261103108,-37.2591313508023));
#272625=CARTESIAN_POINT('Origin',(4.76104848420342,-51.7098072425568,-36.9742798391576));
#272626=CARTESIAN_POINT('',(4.79296103895619,-48.5549566816842,-38.1538301299319));
#272627=CARTESIAN_POINT('Ctrl Pts',(4.76104848420342,-48.3537261103108,
-37.2591313508023));
#272628=CARTESIAN_POINT('Ctrl Pts',(4.76104848420342,-48.3641956404984,
-37.382481908162));
#272629=CARTESIAN_POINT('Ctrl Pts',(4.76253146428112,-48.3814617755203,
-37.5052501260783));
#272630=CARTESIAN_POINT('Ctrl Pts',(4.76582551084937,-48.405493015206,-37.6269199042606));
#272631=CARTESIAN_POINT('Ctrl Pts',(4.76903289751466,-48.4288920401198,
-37.74538878927));
#272632=CARTESIAN_POINT('Ctrl Pts',(4.77395775595718,-48.4587050452691,
-37.8628160339725));
#272633=CARTESIAN_POINT('Ctrl Pts',(4.78087052305202,-48.4949065665866,
-37.9786882576892));
#272634=CARTESIAN_POINT('Ctrl Pts',(4.78437875699289,-48.5132788629558,
-38.0374934890054));
#272635=CARTESIAN_POINT('Ctrl Pts',(4.78839842591371,-48.5332966106966,
-38.0958976385085));
#272636=CARTESIAN_POINT('Ctrl Pts',(4.79296103895619,-48.5549566816842,
-38.1538301299319));
#272637=CARTESIAN_POINT('',(11.5201159294503,-48.5549566816842,-38.1538301299319));
#272638=CARTESIAN_POINT('',(11.5520284842034,-48.5549566816842,-38.1538301299319));
#272639=CARTESIAN_POINT('Ctrl Pts',(11.5201159294506,-48.5549566816842,
-38.1538301299319));
#272640=CARTESIAN_POINT('Ctrl Pts',(11.5379482942249,-48.4703011820194,
-37.9274087109495));
#272641=CARTESIAN_POINT('Ctrl Pts',(11.5475950755165,-48.4099024223757,
-37.6916009878592));
#272642=CARTESIAN_POINT('Ctrl Pts',(11.5516325551658,-48.3663759708428,
-37.386597238529));
#272643=CARTESIAN_POINT('Ctrl Pts',(11.5520284842034,-48.3591392644216,
-37.3229083842203));
#272644=CARTESIAN_POINT('Ctrl Pts',(11.5520284842034,-48.3537261103108,
-37.2591313508023));
#272645=CARTESIAN_POINT('Origin',(11.5520284842034,-43.0735737692781,-43.2488707392779));
#272646=CARTESIAN_POINT('',(11.5520284842034,-39.7316071024856,-42.8297290592317));
#272647=CARTESIAN_POINT('',(11.5520284842034,-44.3815697599695,-40.1450718672117));
#272648=CARTESIAN_POINT('Origin',(11.5520284842034,-43.0735737692781,-43.2488707392779));
#272649=CARTESIAN_POINT('',(11.5201159294502,-45.1702951976398,-40.6129306409918));
#272650=CARTESIAN_POINT('Ctrl Pts',(11.5520284842034,-44.3815697599695,
-40.1450718672117));
#272651=CARTESIAN_POINT('Ctrl Pts',(11.5520284842034,-44.4956485670534,
-40.1931467033848));
#272652=CARTESIAN_POINT('Ctrl Pts',(11.5505454855483,-44.6070732101029,
-40.2475056052893));
#272653=CARTESIAN_POINT('Ctrl Pts',(11.5472513973451,-44.7153625908673,
-40.3079591348944));
#272654=CARTESIAN_POINT('Ctrl Pts',(11.5440439677953,-44.8208031675502,
-40.3668222937663));
#272655=CARTESIAN_POINT('Ctrl Pts',(11.5391190420915,-44.9232710031711,
-40.4314636981042));
#272656=CARTESIAN_POINT('Ctrl Pts',(11.5322061778344,-45.0222857184828,
-40.5017004896391));
#272657=CARTESIAN_POINT('Ctrl Pts',(11.5286980071981,-45.0725341399615,
-40.5373445642926));
#272658=CARTESIAN_POINT('Ctrl Pts',(11.5246784267181,-45.1218926824322,
-40.5744295419386));
#272659=CARTESIAN_POINT('Ctrl Pts',(11.5201159294506,-45.1702951976399,
-40.6129306409918));
#272660=CARTESIAN_POINT('',(4.79296103895619,-45.1702951976398,-40.6129306409918));
#272661=CARTESIAN_POINT('',(11.5520284842034,-45.1702951976398,-40.6129306409918));
#272662=CARTESIAN_POINT('',(4.76104848420342,-44.3815697599695,-40.1450718672117));
#272663=CARTESIAN_POINT('Ctrl Pts',(4.79296103895618,-45.1702951976398,
-40.6129306409918));
#272664=CARTESIAN_POINT('Ctrl Pts',(4.77035892157484,-44.9305143789032,
-40.4222003656407));
#272665=CARTESIAN_POINT('Ctrl Pts',(4.76104848420342,-44.66533506417,-40.2646556081339));
#272666=CARTESIAN_POINT('Ctrl Pts',(4.76104848420342,-44.3815697599695,
-40.1450718672118));
#272667=CARTESIAN_POINT('',(4.76104848420342,-39.7316071024856,-42.8297290592317));
#272668=CARTESIAN_POINT('Origin',(4.76104848420342,-43.0735737692781,-43.2488707392779));
#272669=CARTESIAN_POINT('',(4.79296103895619,-39.7424219671274,-43.7467147117553));
#272670=CARTESIAN_POINT('Ctrl Pts',(4.76104848420342,-39.7316071024856,
-42.8297290592317));
#272671=CARTESIAN_POINT('Ctrl Pts',(4.76104848420342,-39.7162020260021,
-42.952559249018));
#272672=CARTESIAN_POINT('Ctrl Pts',(4.7625314258757,-39.7075659332827,-43.0762329497052));
#272673=CARTESIAN_POINT('Ctrl Pts',(4.76582538552449,-39.7057753139107,
-43.2002387723342));
#272674=CARTESIAN_POINT('Ctrl Pts',(4.76903268308154,-39.7040318046544,
-43.3209820765593));
#272675=CARTESIAN_POINT('Ctrl Pts',(4.77395740161558,-39.708778498989,-43.4420400564706));
#272676=CARTESIAN_POINT('Ctrl Pts',(4.78086996580659,-39.7200972254492,
-43.5629052434041));
#272677=CARTESIAN_POINT('Ctrl Pts',(4.78437833171491,-39.7258418714215,
-43.6242485148189));
#272678=CARTESIAN_POINT('Ctrl Pts',(4.78839818488704,-39.7332795799699,
-43.6855415708931));
#272679=CARTESIAN_POINT('Ctrl Pts',(4.79296103895619,-39.7424219671274,
-43.7467147117553));
#272680=CARTESIAN_POINT('',(11.520115929451,-39.7424219671274,-43.7467147117553));
#272681=CARTESIAN_POINT('',(11.5520284842034,-39.7424219671274,-43.7467147117553));
#272682=CARTESIAN_POINT('Ctrl Pts',(11.5201159294506,-39.7424219671274,
-43.7467147117553));
#272683=CARTESIAN_POINT('Ctrl Pts',(11.5379482942249,-39.7066920532994,
-43.5076402759505));
#272684=CARTESIAN_POINT('Ctrl Pts',(11.5475950755165,-39.6966403338822,
-43.2644279091345));
#272685=CARTESIAN_POINT('Ctrl Pts',(11.5516325551658,-39.7174788849758,
-42.9570395653788));
#272686=CARTESIAN_POINT('Ctrl Pts',(11.5520284842034,-39.7236419753383,
-42.8932378694753));
#272687=CARTESIAN_POINT('Ctrl Pts',(11.5520284842034,-39.7316071024856,
-42.8297290592317));
#272688=CARTESIAN_POINT('Origin',(11.5520284842034,-64.1902433118534,-19.7964332737817));
#272689=CARTESIAN_POINT('',(11.5520284842034,-63.4240670938145,-16.5165864857723));
#272690=CARTESIAN_POINT('',(11.5201159294509,-64.3371598641692,-16.4314910043572));
#272691=CARTESIAN_POINT('Ctrl Pts',(11.5520284842034,-63.4240670938102,
-16.5165864857733));
#272692=CARTESIAN_POINT('Ctrl Pts',(11.5520284842035,-63.6673411199273,
-16.4597573759625));
#272693=CARTESIAN_POINT('Ctrl Pts',(11.5459435973759,-63.9165045298839,
-16.430089037035));
#272694=CARTESIAN_POINT('Ctrl Pts',(11.5280276651045,-64.2239049548286,
-16.4279739330299));
#272695=CARTESIAN_POINT('Ctrl Pts',(11.5242910209322,-64.2806175747128,
-16.4290223146854));
#272696=CARTESIAN_POINT('Ctrl Pts',(11.5201159294506,-64.3371598641692,
-16.4314910043572));
#272697=CARTESIAN_POINT('',(4.79296103895619,-64.3371598641692,-16.4314910043572));
#272698=CARTESIAN_POINT('',(11.5520284842034,-64.3371598641692,-16.4314910043572));
#272699=CARTESIAN_POINT('',(4.76104848420342,-63.4240670938145,-16.5165864857723));
#272700=CARTESIAN_POINT('Ctrl Pts',(4.79296103895618,-64.3371598641692,
-16.4314910043572));
#272701=CARTESIAN_POINT('Ctrl Pts',(4.77035892158601,-64.0310646640203,
-16.418126599299));
#272702=CARTESIAN_POINT('Ctrl Pts',(4.76104848420348,-63.7239276068057,
-16.446538703473));
#272703=CARTESIAN_POINT('Ctrl Pts',(4.76104848420342,-63.4240670938177,
-16.5165864857716));
#272704=CARTESIAN_POINT('',(4.76104848420342,-61.2401701856314,-21.4216992519672));
#272705=CARTESIAN_POINT('Origin',(4.76104848420342,-64.1902433118534,-19.7964332737817));
#272706=CARTESIAN_POINT('',(4.79296103895619,-61.7879102380356,-22.1571994105147));
#272707=CARTESIAN_POINT('Ctrl Pts',(4.76104848420342,-61.2401701856314,
-21.4216992519672));
#272708=CARTESIAN_POINT('Ctrl Pts',(4.76104848420342,-61.2999060970774,
-21.5301278472817));
#272709=CARTESIAN_POINT('Ctrl Pts',(4.76253148048503,-61.3656142043588,
-21.6352599593845));
#272710=CARTESIAN_POINT('Ctrl Pts',(4.76582556303018,-61.4370558175347,
-21.7366369273954));
#272711=CARTESIAN_POINT('Ctrl Pts',(4.76903298692,-61.5066179896073,-21.8353469337836));
#272712=CARTESIAN_POINT('Ctrl Pts',(4.77395790368722,-61.5816160066493,
-21.9304964980193));
#272713=CARTESIAN_POINT('Ctrl Pts',(4.78087075471546,-61.6618177977816,
-22.0216269866694));
#272714=CARTESIAN_POINT('Ctrl Pts',(4.78437893387933,-61.7025191309083,
-22.0678744871825));
#272715=CARTESIAN_POINT('Ctrl Pts',(4.78839852622511,-61.7445604645742,
-22.1130863605567));
#272716=CARTESIAN_POINT('Ctrl Pts',(4.79296103895619,-61.7879102380356,
-22.1571994105147));
#272717=CARTESIAN_POINT('',(11.5201159294506,-61.7879102380356,-22.1571994105147));
#272718=CARTESIAN_POINT('',(11.5520284842034,-61.7879102380356,-22.1571994105147));
#272719=CARTESIAN_POINT('',(11.5520284842034,-61.2401701856314,-21.4216992519671));
#272720=CARTESIAN_POINT('Ctrl Pts',(11.5201159294506,-61.7879102380356,
-22.1571994105147));
#272721=CARTESIAN_POINT('Ctrl Pts',(11.5379482942249,-61.6184797029751,
-21.9847856454419));
#272722=CARTESIAN_POINT('Ctrl Pts',(11.5475950755165,-61.4673910487542,
-21.7939309598791));
#272723=CARTESIAN_POINT('Ctrl Pts',(11.5516325551658,-61.3035714555409,
-21.5329999728961));
#272724=CARTESIAN_POINT('Ctrl Pts',(11.5520284842034,-61.2710558044587,
-21.4777607430166));
#272725=CARTESIAN_POINT('Ctrl Pts',(11.5520284842034,-61.2401701856314,
-21.4216992519671));
#272726=CARTESIAN_POINT('Origin',(11.5520284842034,-64.1902433118534,-19.7964332737817));
#272727=CARTESIAN_POINT('Origin',(11.5520284842034,-58.8527574905876,-29.0412299008925));
#272728=CARTESIAN_POINT('',(11.5520284842034,-58.7852425524918,-25.6737586414698));
#272729=CARTESIAN_POINT('',(11.5201159294504,-59.6960744004836,-25.7803653622482));
#272730=CARTESIAN_POINT('Ctrl Pts',(11.5520284842034,-58.7852425524873,
-25.6737586414699));
#272731=CARTESIAN_POINT('Ctrl Pts',(11.5520284842035,-59.0350158937629,
-25.6687508981586));
#272732=CARTESIAN_POINT('Ctrl Pts',(11.5459435973759,-59.2849028799128,
-25.6915348694728));
#272733=CARTESIAN_POINT('Ctrl Pts',(11.5280276651045,-59.5860256228871,
-25.7533781276734));
#272734=CARTESIAN_POINT('Ctrl Pts',(11.5242910209322,-59.6412809651556,
-25.7661948163652));
#272735=CARTESIAN_POINT('Ctrl Pts',(11.5201159294506,-59.6960744004836,
-25.7803653622482));
#272736=CARTESIAN_POINT('',(4.79296103895619,-59.6960744004836,-25.7803653622482));
#272737=CARTESIAN_POINT('',(11.5520284842034,-59.6960744004836,-25.7803653622482));
#272738=CARTESIAN_POINT('',(4.76104848420342,-58.7852425524918,-25.6737586414698));
#272739=CARTESIAN_POINT('Ctrl Pts',(4.79296103895618,-59.6960744004836,
-25.7803653622482));
#272740=CARTESIAN_POINT('Ctrl Pts',(4.77035892158043,-59.399446730841,-25.7036522308722));
#272741=CARTESIAN_POINT('Ctrl Pts',(4.76104848420348,-59.0931141466079,
-25.6675860775439));
#272742=CARTESIAN_POINT('Ctrl Pts',(4.76104848420342,-58.785242552495,-25.6737586414697));
#272743=CARTESIAN_POINT('',(4.76104848420342,-55.6292387426312,-30.0176252263));
#272744=CARTESIAN_POINT('Origin',(4.76104848420342,-58.8527574905876,-29.0412299008925));
#272745=CARTESIAN_POINT('',(4.79296103895619,-56.0120902791558,-30.8509345021466));
#272746=CARTESIAN_POINT('Ctrl Pts',(4.76104848420342,-55.6292387426312,
-30.0176252263));
#272747=CARTESIAN_POINT('Ctrl Pts',(4.76104848420342,-55.6651257148422,
-30.1361042119314));
#272748=CARTESIAN_POINT('Ctrl Pts',(4.76253148100061,-55.7075397574459,
-30.2526004442625));
#272749=CARTESIAN_POINT('Ctrl Pts',(4.76582556519912,-55.7563427586828,
-30.3666156575337));
#272750=CARTESIAN_POINT('Ctrl Pts',(4.76903299054489,-55.803861878925,-30.477631424834));
#272751=CARTESIAN_POINT('Ctrl Pts',(4.77395790968286,-55.8574383198187,
-30.5862947331828));
#272752=CARTESIAN_POINT('Ctrl Pts',(4.7808707646055,-55.9169404382669,-30.6921087199474));
#272753=CARTESIAN_POINT('Ctrl Pts',(4.78437894136648,-55.9471369274894,
-30.7458078317481));
#272754=CARTESIAN_POINT('Ctrl Pts',(4.78839853042556,-55.9788594516498,
-30.7987725514947));
#272755=CARTESIAN_POINT('Ctrl Pts',(4.79296103895619,-56.0120902791558,
-30.8509345021466));
#272756=CARTESIAN_POINT('',(11.5201159294502,-56.0120902791558,-30.8509345021466));
#272757=CARTESIAN_POINT('',(11.5520284842034,-56.0120902791558,-30.8509345021466));
#272758=CARTESIAN_POINT('',(11.5520284842034,-55.6292387426312,-30.0176252263));
#272759=CARTESIAN_POINT('Ctrl Pts',(11.5201159294506,-56.0120902791558,
-30.8509345021466));
#272760=CARTESIAN_POINT('Ctrl Pts',(11.5379482942249,-55.8822090452119,
-30.6470618024867));
#272761=CARTESIAN_POINT('Ctrl Pts',(11.5475950755165,-55.7741029609635,
-30.4289646521523));
#272762=CARTESIAN_POINT('Ctrl Pts',(11.5516325551658,-55.6681138215991,
-30.1396756246635));
#272763=CARTESIAN_POINT('Ctrl Pts',(11.5520284842034,-55.6477935971904,
-30.0788831204959));
#272764=CARTESIAN_POINT('Ctrl Pts',(11.5520284842034,-55.6292387426312,
-30.0176252262999));
#272765=CARTESIAN_POINT('Origin',(11.5520284842034,-58.8527574905876,-29.0412299008925));
#272766=CARTESIAN_POINT('Origin',(11.5520284842034,23.7681211036462,-29.0412299008916));
#272767=CARTESIAN_POINT('',(11.520115929451,24.6114380135421,-25.7803653622474));
#272768=CARTESIAN_POINT('',(11.5520284842034,23.7006061655503,-25.6737586414689));
#272769=CARTESIAN_POINT('Ctrl Pts',(11.5201159294506,24.6114380135421,-25.7803653622474));
#272770=CARTESIAN_POINT('Ctrl Pts',(11.5379482942249,24.3774080454967,-25.7198410972446));
#272771=CARTESIAN_POINT('Ctrl Pts',(11.5475950755165,24.1365787122577,-25.6844218272471));
#272772=CARTESIAN_POINT('Ctrl Pts',(11.5516325551658,23.8286960522908,-25.6730153913783));
#272773=CARTESIAN_POINT('Ctrl Pts',(11.5520284842034,23.7645996503902,-25.6724756264602));
#272774=CARTESIAN_POINT('Ctrl Pts',(11.5520284842034,23.7006061655553,-25.6737586414688));
#272775=CARTESIAN_POINT('',(11.5520284842034,20.5446023556898,-30.0176252262992));
#272776=CARTESIAN_POINT('Origin',(11.5520284842034,23.7681211036462,-29.0412299008916));
#272777=CARTESIAN_POINT('',(11.5201159294503,20.9274538922144,-30.8509345021458));
#272778=CARTESIAN_POINT('Ctrl Pts',(11.5520284842034,20.5446023556898,-30.0176252262992));
#272779=CARTESIAN_POINT('Ctrl Pts',(11.5520284842034,20.5804893279013,-30.1361042119321));
#272780=CARTESIAN_POINT('Ctrl Pts',(11.5505454874062,20.6229033705057,-30.2526004442646));
#272781=CARTESIAN_POINT('Ctrl Pts',(11.5472514032076,20.6717063717434,-30.3666156575372));
#272782=CARTESIAN_POINT('Ctrl Pts',(11.5440439778617,20.7192254919869,-30.4776314248403));
#272783=CARTESIAN_POINT('Ctrl Pts',(11.5391190587235,20.7728019328823,-30.5862947331918));
#272784=CARTESIAN_POINT('Ctrl Pts',(11.5322062038005,20.8323040513325,-30.6921087199588));
#272785=CARTESIAN_POINT('Ctrl Pts',(11.5286980270397,20.8625005405529,-30.7458078317553));
#272786=CARTESIAN_POINT('Ctrl Pts',(11.5246784379809,20.894223064711,-30.7987725514979));
#272787=CARTESIAN_POINT('Ctrl Pts',(11.5201159294506,20.9274538922145,-30.8509345021458));
#272788=CARTESIAN_POINT('',(4.79296103895619,20.9274538922144,-30.8509345021458));
#272789=CARTESIAN_POINT('',(11.5520284842034,20.9274538922144,-30.8509345021458));
#272790=CARTESIAN_POINT('',(4.76104848420342,20.5446023556898,-30.0176252262992));
#272791=CARTESIAN_POINT('Ctrl Pts',(4.79296103895619,20.9274538922145,-30.8509345021458));
#272792=CARTESIAN_POINT('Ctrl Pts',(4.77035892158035,20.7628323778119,-30.5925304853049));
#272793=CARTESIAN_POINT('Ctrl Pts',(4.76104848420342,20.6338694532122,-30.3123359392156));
#272794=CARTESIAN_POINT('Ctrl Pts',(4.76104848420342,20.5446023556898,-30.0176252262992));
#272795=CARTESIAN_POINT('',(4.76104848420342,23.7006061655503,-25.6737586414689));
#272796=CARTESIAN_POINT('Origin',(4.76104848420342,23.7681211036462,-29.0412299008916));
#272797=CARTESIAN_POINT('',(4.79296103895619,24.6114380135421,-25.7803653622474));
#272798=CARTESIAN_POINT('Ctrl Pts',(4.76104848420342,23.7006061655501,-25.6737586414689));
#272799=CARTESIAN_POINT('Ctrl Pts',(4.76104848420341,23.8861826621397,-25.6700379903589));
#272800=CARTESIAN_POINT('Ctrl Pts',(4.76439185786763,24.0720879013436,-25.6816555797029));
#272801=CARTESIAN_POINT('Ctrl Pts',(4.77719931294499,24.376417237712,-25.7262486108204));
#272802=CARTESIAN_POINT('Ctrl Pts',(4.78408071207329,24.4948935931612,-25.7502249257783));
#272803=CARTESIAN_POINT('Ctrl Pts',(4.79296103895618,24.6114380135421,-25.7803653622474));
#272804=CARTESIAN_POINT('',(11.5520284842034,24.6114380135421,-25.7803653622474));
#272805=CARTESIAN_POINT('Origin',(11.5520284842034,16.6251708556156,-36.9742798391569));
#272806=CARTESIAN_POINT('',(11.5520284842034,17.2592679242302,-33.6663587612776));
#272807=CARTESIAN_POINT('',(11.5520284842034,13.2690897233696,-37.2591313508016));
#272808=CARTESIAN_POINT('Origin',(11.5520284842034,16.6251708556156,-36.9742798391569));
#272809=CARTESIAN_POINT('',(11.5201159294504,13.470320294743,-38.1538301299313));
#272810=CARTESIAN_POINT('Ctrl Pts',(11.5520284842034,13.2690897233696,-37.2591313508016));
#272811=CARTESIAN_POINT('Ctrl Pts',(11.5520284842034,13.2795592535577,-37.3824819081667));
#272812=CARTESIAN_POINT('Ctrl Pts',(11.5505455041256,13.2968253885807,-37.5052501260884));
#272813=CARTESIAN_POINT('Ctrl Pts',(11.547251457557,13.320856628268,-37.6269199042761));
#272814=CARTESIAN_POINT('Ctrl Pts',(11.544044070892,13.3442556531797,-37.7453887892715));
#272815=CARTESIAN_POINT('Ctrl Pts',(11.53911921245,13.3740686583253,-37.8628160339603));
#272816=CARTESIAN_POINT('Ctrl Pts',(11.5322064453563,13.4102701796377,-37.9786882576637));
#272817=CARTESIAN_POINT('Ctrl Pts',(11.5286982114151,13.428642476009,-38.0374934889883));
#272818=CARTESIAN_POINT('Ctrl Pts',(11.5246785424938,13.4486602237524,-38.0958976384997));
#272819=CARTESIAN_POINT('Ctrl Pts',(11.5201159294506,13.470320294743,-38.1538301299313));
#272820=CARTESIAN_POINT('',(4.79296103895619,13.470320294743,-38.1538301299313));
#272821=CARTESIAN_POINT('',(11.5520284842034,13.470320294743,-38.1538301299313));
#272822=CARTESIAN_POINT('',(4.76104848420342,13.2690897233696,-37.2591313508017));
#272823=CARTESIAN_POINT('Ctrl Pts',(4.79296103895619,13.470320294743,-38.1538301299313));
#272824=CARTESIAN_POINT('Ctrl Pts',(4.77035892158041,13.3630213714567,-37.8668461234347));
#272825=CARTESIAN_POINT('Ctrl Pts',(4.76104848420342,13.2951323180111,-37.5659616007325));
#272826=CARTESIAN_POINT('Ctrl Pts',(4.76104848420342,13.2690897233696,-37.2591313508017));
#272827=CARTESIAN_POINT('',(4.76104848420342,17.2592679242302,-33.6663587612776));
#272828=CARTESIAN_POINT('Origin',(4.76104848420342,16.6251708556156,-36.9742798391569));
#272829=CARTESIAN_POINT('',(4.79296103895619,18.1280311274457,-33.9600084589958));
#272830=CARTESIAN_POINT('Ctrl Pts',(4.76104848420342,17.2592679242302,-33.6663587612776));
#272831=CARTESIAN_POINT('Ctrl Pts',(4.76104848420342,17.3808488290439,-33.6896646665658));
#272832=CARTESIAN_POINT('Ctrl Pts',(4.76253147492084,17.5011401217906,-33.7196691161167));
#272833=CARTESIAN_POINT('Ctrl Pts',(4.76582554549253,17.6196318267452,-33.7562868369354));
#272834=CARTESIAN_POINT('Ctrl Pts',(4.7690329568029,17.7350062931944,-33.7919412315082));
#272835=CARTESIAN_POINT('Ctrl Pts',(4.77395785392703,17.8486743622794,-33.8338656362274));
#272836=CARTESIAN_POINT('Ctrl Pts',(4.7808706770485,17.9601281306821,-33.8819810649277));
#272837=CARTESIAN_POINT('Ctrl Pts',(4.78437887452869,18.0166899466867,-33.9063992256067));
#272838=CARTESIAN_POINT('Ctrl Pts',(4.78839849253368,18.0726808984023,-33.9324118527932));
#272839=CARTESIAN_POINT('Ctrl Pts',(4.79296103895619,18.1280311274457,-33.9600084589958));
#272840=CARTESIAN_POINT('',(11.5201159294502,18.1280311274457,-33.9600084589958));
#272841=CARTESIAN_POINT('',(11.5520284842034,18.1280311274457,-33.9600084589958));
#272842=CARTESIAN_POINT('Ctrl Pts',(11.5201159294506,18.1280311274458,-33.9600084589958));
#272843=CARTESIAN_POINT('Ctrl Pts',(11.5379482942249,17.9116989779746,-33.8521492280388));
#272844=CARTESIAN_POINT('Ctrl Pts',(11.5475950755165,17.6834964237933,-33.7674327201988));
#272845=CARTESIAN_POINT('Ctrl Pts',(11.5516325551658,17.3847132700051,-33.6922631379132));
#272846=CARTESIAN_POINT('Ctrl Pts',(11.5520284842034,17.3221297517055,-33.6784087768588));
#272847=CARTESIAN_POINT('Ctrl Pts',(11.5520284842034,17.2592679242302,-33.6663587612776));
#272848=CARTESIAN_POINT('Origin',(11.5520284842034,29.1056069249118,-19.7964332737808));
#272849=CARTESIAN_POINT('',(11.5201159294503,29.2525234772276,-16.4314910043563));
#272850=CARTESIAN_POINT('',(11.5520284842034,28.3394307068729,-16.5165864857714));
#272851=CARTESIAN_POINT('Ctrl Pts',(11.5201159294506,29.2525234772276,-16.4314910043563));
#272852=CARTESIAN_POINT('Ctrl Pts',(11.5379482942249,29.011023923212,-16.420946906116));
#272853=CARTESIAN_POINT('Ctrl Pts',(11.5475950755165,28.7680932084051,-16.4363728660204));
#272854=CARTESIAN_POINT('Ctrl Pts',(11.5516325551658,28.4645669918831,-16.4892280925497));
#272855=CARTESIAN_POINT('Ctrl Pts',(11.5520284842034,28.4017590267117,-16.5020265140846));
#272856=CARTESIAN_POINT('Ctrl Pts',(11.5520284842034,28.3394307068777,-16.5165864857703));
#272857=CARTESIAN_POINT('',(11.5520284842034,26.1555337986899,-21.4216992519662));
#272858=CARTESIAN_POINT('Origin',(11.5520284842034,29.1056069249118,-19.7964332737808));
#272859=CARTESIAN_POINT('',(11.5201159294506,26.7032738510941,-22.1571994105138));
#272860=CARTESIAN_POINT('Ctrl Pts',(11.5520284842034,26.1555337986899,-21.4216992519662));
#272861=CARTESIAN_POINT('Ctrl Pts',(11.5520284842034,26.2152697101401,-21.5301278472884));
#272862=CARTESIAN_POINT('Ctrl Pts',(11.5505454879216,26.2809778174266,-21.6352599593984));
#272863=CARTESIAN_POINT('Ctrl Pts',(11.547251405376,26.3524194306083,-21.7366369274159));
#272864=CARTESIAN_POINT('Ctrl Pts',(11.5440439814859,26.4219816026811,-21.8353469338028));
#272865=CARTESIAN_POINT('Ctrl Pts',(11.5391190647185,26.4969796197233,-21.9304964980372));
#272866=CARTESIAN_POINT('Ctrl Pts',(11.53220621369,26.5771814108555,-22.021626986686));
#272867=CARTESIAN_POINT('Ctrl Pts',(11.5286980345265,26.6178827439774,-22.0678744871931));
#272868=CARTESIAN_POINT('Ctrl Pts',(11.5246784421811,26.6599240776381,-22.1130863605614));
#272869=CARTESIAN_POINT('Ctrl Pts',(11.5201159294506,26.7032738510941,-22.1571994105138));
#272870=CARTESIAN_POINT('',(4.79296103895619,26.7032738510941,-22.1571994105138));
#272871=CARTESIAN_POINT('',(11.5520284842034,26.7032738510941,-22.1571994105138));
#272872=CARTESIAN_POINT('',(4.76104848420342,26.1555337986899,-21.4216992519663));
#272873=CARTESIAN_POINT('Ctrl Pts',(4.79296103895619,26.7032738510941,-22.1571994105138));
#272874=CARTESIAN_POINT('Ctrl Pts',(4.77035892158039,26.4885244956969,-21.9386688788256));
#272875=CARTESIAN_POINT('Ctrl Pts',(4.76104848420342,26.3041239985807,-21.6914101555361));
#272876=CARTESIAN_POINT('Ctrl Pts',(4.76104848420342,26.1555337986899,-21.4216992519663));
#272877=CARTESIAN_POINT('',(4.76104848420342,28.3394307068729,-16.5165864857714));
#272878=CARTESIAN_POINT('Origin',(4.76104848420342,29.1056069249118,-19.7964332737808));
#272879=CARTESIAN_POINT('',(4.79296103895619,29.2525234772276,-16.4314910043563));
#272880=CARTESIAN_POINT('Ctrl Pts',(4.76104848420342,28.3394307068727,-16.5165864857715));
#272881=CARTESIAN_POINT('Ctrl Pts',(4.76104848420341,28.5201783449009,-16.4743636166331));
#272882=CARTESIAN_POINT('Ctrl Pts',(4.76439185786762,28.7044365412357,-16.4470754611615));
#272883=CARTESIAN_POINT('Ctrl Pts',(4.77719931294497,29.0113869639358,-16.4274204006687));
#272884=CARTESIAN_POINT('Ctrl Pts',(4.78408071207328,29.1322592829447,-16.4262401562358));
#272885=CARTESIAN_POINT('Ctrl Pts',(4.79296103895619,29.2525234772276,-16.4314910043563));
#272886=CARTESIAN_POINT('',(11.5520284842034,29.2525234772276,-16.4314910043563));
#272887=CARTESIAN_POINT('Origin',(11.5520284842034,7.98893738233704,-43.2488707392774));
#272888=CARTESIAN_POINT('',(11.5520284842034,9.29693337302835,-40.1450718672112));
#272889=CARTESIAN_POINT('',(11.5520284842034,4.64697071554456,-42.8297290592312));
#272890=CARTESIAN_POINT('Origin',(11.5520284842034,7.98893738233704,-43.2488707392774));
#272891=CARTESIAN_POINT('',(11.5201159294509,4.65778558018634,-43.7467147117548));
#272892=CARTESIAN_POINT('Ctrl Pts',(11.5520284842034,4.64697071554456,-42.8297290592312));
#272893=CARTESIAN_POINT('Ctrl Pts',(11.5520284842034,4.63156563906103,-42.9525592490173));
#272894=CARTESIAN_POINT('Ctrl Pts',(11.5505455425311,4.62292954634169,-43.0762329497044));
#272895=CARTESIAN_POINT('Ctrl Pts',(11.5472515828824,4.62113892696966,-43.2002387723334));
#272896=CARTESIAN_POINT('Ctrl Pts',(11.5440442853252,4.61939541771331,-43.3209820765611));
#272897=CARTESIAN_POINT('Ctrl Pts',(11.5391195667911,4.62414211204812,-43.442040056475));
#272898=CARTESIAN_POINT('Ctrl Pts',(11.5322070025998,4.63546083850879,-43.5629052434111));
#272899=CARTESIAN_POINT('Ctrl Pts',(11.5286986366916,4.64120548448104,-43.6242485148234));
#272900=CARTESIAN_POINT('Ctrl Pts',(11.5246787835196,4.64864319302917,-43.6855415708951));
#272901=CARTESIAN_POINT('Ctrl Pts',(11.5201159294506,4.65778558018632,-43.7467147117548));
#272902=CARTESIAN_POINT('',(4.79296103895619,4.65778558018634,-43.7467147117548));
#272903=CARTESIAN_POINT('',(11.5520284842034,4.65778558018634,-43.7467147117548));
#272904=CARTESIAN_POINT('',(4.76104848420342,4.64697071554454,-42.8297290592312));
#272905=CARTESIAN_POINT('Ctrl Pts',(4.79296103895618,4.65778558018634,-43.7467147117548));
#272906=CARTESIAN_POINT('Ctrl Pts',(4.77035892157484,4.61249872582977,-43.4436932937131));
#272907=CARTESIAN_POINT('Ctrl Pts',(4.76104848420341,4.60865062096244,-43.1352688918427));
#272908=CARTESIAN_POINT('Ctrl Pts',(4.76104848420342,4.64697071554455,-42.8297290592312));
#272909=CARTESIAN_POINT('',(4.76104848420342,9.29693337302838,-40.1450718672112));
#272910=CARTESIAN_POINT('Origin',(4.76104848420342,7.98893738233704,-43.2488707392774));
#272911=CARTESIAN_POINT('',(4.79296103895619,10.0856588106987,-40.6129306409912));
#272912=CARTESIAN_POINT('Ctrl Pts',(4.76104848420342,9.29693337302838,-40.1450718672112));
#272913=CARTESIAN_POINT('Ctrl Pts',(4.76104848420342,9.41101218012303,-40.1931467033887));
#272914=CARTESIAN_POINT('Ctrl Pts',(4.76253148285884,9.52243682318274,-40.247505605299));
#272915=CARTESIAN_POINT('Ctrl Pts',(4.76582557106269,9.63072620395674,-40.3079591349109));
#272916=CARTESIAN_POINT('Ctrl Pts',(4.76903300061286,9.73616678064156,-40.3668222937853));
#272917=CARTESIAN_POINT('Ctrl Pts',(4.77395792631717,9.83863461626415,-40.4314636981259));
#272918=CARTESIAN_POINT('Ctrl Pts',(4.78087079057491,9.93764933157731,-40.5017004896638));
#272919=CARTESIAN_POINT('Ctrl Pts',(4.7843789612106,9.98789775304374,-40.5373445643096));
#272920=CARTESIAN_POINT('Ctrl Pts',(4.7883985416898,10.0372562955025,-40.5744295419471));
#272921=CARTESIAN_POINT('Ctrl Pts',(4.79296103895619,10.0856588106987,-40.6129306409912));
#272922=CARTESIAN_POINT('',(11.5201159294506,10.0856588106987,-40.6129306409912));
#272923=CARTESIAN_POINT('',(11.5520284842034,10.0856588106987,-40.6129306409912));
#272924=CARTESIAN_POINT('Ctrl Pts',(11.5201159294506,10.0856588106987,-40.6129306409912));
#272925=CARTESIAN_POINT('Ctrl Pts',(11.5379482942249,9.8964792328107,-40.462450410039));
#272926=CARTESIAN_POINT('Ctrl Pts',(11.5475950755165,9.69087700434215,-40.3321391822639));
#272927=CARTESIAN_POINT('Ctrl Pts',(11.5516325551658,9.41425161427548,-40.1964917250111));
#272928=CARTESIAN_POINT('Ctrl Pts',(11.5520284842034,9.35591617963722,-40.169928269879));
#272929=CARTESIAN_POINT('Ctrl Pts',(11.5520284842034,9.29693337302835,-40.1450718672112));
#272930=CARTESIAN_POINT('Origin',(11.5520284842034,-1.76313447216117,-47.5907728700901));
#272931=CARTESIAN_POINT('',(11.5520284842034,0.161594739352518,-44.8267471082258));
#272932=CARTESIAN_POINT('',(11.5520284842034,-4.944926693626,-46.485956501036));
#272933=CARTESIAN_POINT('Origin',(11.5520284842034,-1.76313447216117,-47.5907728700901));
#272934=CARTESIAN_POINT('',(11.5201159294504,-5.12500019719618,-47.3851523537529));
#272935=CARTESIAN_POINT('Ctrl Pts',(11.5520284842034,-4.94492669362599,
-46.485956501036));
#272936=CARTESIAN_POINT('Ctrl Pts',(11.5520284842034,-4.98553194227204,
-46.6028967165428));
#272937=CARTESIAN_POINT('Ctrl Pts',(11.550545616777,-5.01969184244845,-46.7220693474121));
#272938=CARTESIAN_POINT('Ctrl Pts',(11.5472518253861,-5.04722524969846,
-46.8429900493421));
#272939=CARTESIAN_POINT('Ctrl Pts',(11.5440447002121,-5.07403419812174,
-46.9607290865747));
#272940=CARTESIAN_POINT('Ctrl Pts',(11.5391202523742,-5.09456054853041,
-47.0801252587079));
#272941=CARTESIAN_POINT('Ctrl Pts',(11.5322080809718,-5.10861875091385,
-47.2006991758331));
#272942=CARTESIAN_POINT('Ctrl Pts',(11.5286994596642,-5.11575470075611,
-47.261902550306));
#272943=CARTESIAN_POINT('Ctrl Pts',(11.524679249925,-5.12122380413464,-47.3234088729758));
#272944=CARTESIAN_POINT('Ctrl Pts',(11.5201159294506,-5.12500019719618,
-47.3851523537529));
#272945=CARTESIAN_POINT('',(4.79296103895619,-5.12500019719618,-47.3851523537529));
#272946=CARTESIAN_POINT('',(11.5520284842034,-5.12500019719618,-47.3851523537529));
#272947=CARTESIAN_POINT('',(4.76104848420342,-4.94492669362602,-46.485956501036));
#272948=CARTESIAN_POINT('Ctrl Pts',(4.79296103895618,-5.12500019719618,
-47.3851523537529));
#272949=CARTESIAN_POINT('Ctrl Pts',(4.77035892158036,-5.10629572975537,
-47.0793370143381));
#272950=CARTESIAN_POINT('Ctrl Pts',(4.76104848420342,-5.04593470543677,
-46.7768523596485));
#272951=CARTESIAN_POINT('Ctrl Pts',(4.76104848420342,-4.94492669362601,
-46.485956501036));
#272952=CARTESIAN_POINT('',(4.76104848420342,0.161594739352547,-44.8267471082258));
#272953=CARTESIAN_POINT('Origin',(4.76104848420342,-1.76313447216117,-47.5907728700901));
#272954=CARTESIAN_POINT('',(4.79296103895619,0.835811325126992,-45.448367284618));
#272955=CARTESIAN_POINT('Ctrl Pts',(4.76104848420342,0.161594739352541,
-44.8267471082258));
#272956=CARTESIAN_POINT('Ctrl Pts',(4.76104848420342,0.263185006973524,
-44.8974894863879));
#272957=CARTESIAN_POINT('Ctrl Pts',(4.76253147347957,0.360872606791814,
-44.9738267448727));
#272958=CARTESIAN_POINT('Ctrl Pts',(4.76582553976561,0.454226339754833,
-45.0554735552757));
#272959=CARTESIAN_POINT('Ctrl Pts',(4.76903294718512,0.54512416321815,-45.134972436818));
#272960=CARTESIAN_POINT('Ctrl Pts',(4.77395783802177,0.631912869766447,
-45.2195051911972));
#272961=CARTESIAN_POINT('Ctrl Pts',(4.78087065106457,0.714160596304464,
-45.3087930763068));
#272962=CARTESIAN_POINT('Ctrl Pts',(4.78437885482611,0.755900736220323,
-45.35410604694));
#272963=CARTESIAN_POINT('Ctrl Pts',(4.7883984814575,0.796470830268012,-45.400643448165));
#272964=CARTESIAN_POINT('Ctrl Pts',(4.79296103895619,0.835811325126995,
-45.448367284618));
#272965=CARTESIAN_POINT('',(11.5201159294506,0.835811325126992,-45.448367284618));
#272966=CARTESIAN_POINT('',(11.5520284842034,0.835811325126992,-45.448367284618));
#272967=CARTESIAN_POINT('Ctrl Pts',(11.5201159294506,0.835811325126992,
-45.448367284618));
#272968=CARTESIAN_POINT('Ctrl Pts',(11.5379482942249,0.682052374159662,
-45.261842761847));
#272969=CARTESIAN_POINT('Ctrl Pts',(11.5475950755165,0.508036275376835,
-45.0916320400934));
#272970=CARTESIAN_POINT('Ctrl Pts',(11.5516325551658,0.26565850597392,-44.9014351526643));
#272971=CARTESIAN_POINT('Ctrl Pts',(11.5520284842034,0.214120693415193,
-44.8633235539094));
#272972=CARTESIAN_POINT('Ctrl Pts',(11.5520284842034,0.161594739352511,
-44.8267471082258));
#272973=CARTESIAN_POINT('Origin',(11.5520284842034,-12.2048323722047,-49.8102242737206));
#272974=CARTESIAN_POINT('',(11.5520284842034,-9.7474898422873,-47.5067728111187));
#272975=CARTESIAN_POINT('',(11.5520284842034,-15.0873905603309,-48.0680189924833));
#272976=CARTESIAN_POINT('Origin',(11.5520284842034,-12.2048323722047,-49.8102242737206));
#272977=CARTESIAN_POINT('',(11.5201159294509,-15.4504823559185,-48.9101258718094));
#272978=CARTESIAN_POINT('Ctrl Pts',(11.5520284842034,-15.0873905603309,
-48.0680189924833));
#272979=CARTESIAN_POINT('Ctrl Pts',(11.5520284842034,-15.1514184267909,
-48.173956021099));
#272980=CARTESIAN_POINT('Ctrl Pts',(11.5505457686483,-15.2096066120264,
-48.2834165710142));
#272981=CARTESIAN_POINT('Ctrl Pts',(11.5472523215541,-15.2616772101935,
-48.3959644782058));
#272982=CARTESIAN_POINT('Ctrl Pts',(11.5440455490482,-15.3123774515486,
-48.5055504299616));
#272983=CARTESIAN_POINT('Ctrl Pts',(11.5391216550271,-15.3572776080623,
-48.6180632708147));
#272984=CARTESIAN_POINT('Ctrl Pts',(11.5322102873381,-15.3960965020979,
-48.7330726175836));
#272985=CARTESIAN_POINT('Ctrl Pts',(11.5287011435043,-15.4158062164073,
-48.7914668975864));
#272986=CARTESIAN_POINT('Ctrl Pts',(11.5246802042203,-15.4339478375954,
-48.8505043248629));
#272987=CARTESIAN_POINT('Ctrl Pts',(11.5201159294506,-15.4504823559185,
-48.9101258718094));
#272988=CARTESIAN_POINT('',(4.79296103895619,-15.4504823559185,-48.9101258718094));
#272989=CARTESIAN_POINT('',(11.5520284842034,-15.4504823559185,-48.9101258718094));
#272990=CARTESIAN_POINT('',(4.76104848420342,-15.0873905603309,-48.0680189924834));
#272991=CARTESIAN_POINT('Ctrl Pts',(4.79296103895619,-15.4504823559185,
-48.9101258718094));
#272992=CARTESIAN_POINT('Ctrl Pts',(4.77035892158032,-15.3686040416723,
-48.6148822087441));
#272993=CARTESIAN_POINT('Ctrl Pts',(4.76104848420342,-15.2466719545542,
-48.3315573321263));
#272994=CARTESIAN_POINT('Ctrl Pts',(4.76104848420342,-15.0873905603309,
-48.0680189924834));
#272995=CARTESIAN_POINT('',(4.76104848420342,-9.74748984228727,-47.5067728111187));
#272996=CARTESIAN_POINT('Origin',(4.76104848420342,-12.2048323722047,-49.8102242737206));
#272997=CARTESIAN_POINT('',(4.79296103895619,-9.21724860845719,-48.2549866055502));
#272998=CARTESIAN_POINT('Ctrl Pts',(4.76104848420342,-9.74748984228727,
-47.5067728111187));
#272999=CARTESIAN_POINT('Ctrl Pts',(4.76104848420342,-9.66282867327375,
-47.5970901000337));
#273000=CARTESIAN_POINT('Ctrl Pts',(4.76253144075005,-9.58314800674111,
-47.6920685179983));
#273001=CARTESIAN_POINT('Ctrl Pts',(4.76582543152432,-9.50881029780304,
-47.7913393066709));
#273002=CARTESIAN_POINT('Ctrl Pts',(4.76903276223637,-9.43642830487133,
-47.8879984266072));
#273003=CARTESIAN_POINT('Ctrl Pts',(4.77395753238408,-9.36911211029268,
-47.988726987311));
#273004=CARTESIAN_POINT('Ctrl Pts',(4.78087016904751,-9.30722618608076,
-48.0931625382006));
#273005=CARTESIAN_POINT('Ctrl Pts',(4.78437848714111,-9.27581769201065,
-48.1461659218068));
#273006=CARTESIAN_POINT('Ctrl Pts',(4.78839827319888,-9.24580837914143,
-48.2001237965154));
#273007=CARTESIAN_POINT('Ctrl Pts',(4.79296103895619,-9.21724860845719,
-48.2549866055502));
#273008=CARTESIAN_POINT('',(11.5201159294506,-9.21724860845719,-48.2549866055502));
#273009=CARTESIAN_POINT('',(11.5520284842034,-9.21724860845719,-48.2549866055502));
#273010=CARTESIAN_POINT('Ctrl Pts',(11.5201159294506,-9.21724860845719,
-48.2549866055502));
#273011=CARTESIAN_POINT('Ctrl Pts',(11.5379482942249,-9.32886692852894,
-48.0405698076498));
#273012=CARTESIAN_POINT('Ctrl Pts',(11.5475950755165,-9.46369155908738,
-47.8378986172198));
#273013=CARTESIAN_POINT('Ctrl Pts',(11.5516325551658,-9.66122863624646,
-47.6014648162607));
#273014=CARTESIAN_POINT('Ctrl Pts',(11.5520284842034,-9.70371637701088,
-47.5534707336284));
#273015=CARTESIAN_POINT('Ctrl Pts',(11.5520284842034,-9.7474898422873,-47.5067728111187));
#273016=CARTESIAN_POINT('Origin',(15.4290484842034,-17.542318193471,0.972561099047131));
#273017=CARTESIAN_POINT('',(6.14788848420341,-17.9270891962423,55.333062537043));
#273018=CARTESIAN_POINT('',(6.14788848420342,-17.1575471907001,55.333062537043));
#273019=CARTESIAN_POINT('Origin',(6.14788848420341,-17.542318193471,0.972561099047131));
#273020=CARTESIAN_POINT('',(4.79296103895619,-15.4504823559191,50.8552480699037));
#273021=CARTESIAN_POINT('Ctrl Pts',(4.79296103895619,-15.4504823559191,
50.8552480699037));
#273022=CARTESIAN_POINT('Ctrl Pts',(4.80658157259404,-15.4998240310752,
51.0331684026437));
#273023=CARTESIAN_POINT('Ctrl Pts',(4.8245384335836,-15.5510803275331,51.2105179282822));
#273024=CARTESIAN_POINT('Ctrl Pts',(5.02532215959839,-16.0303748306657,
52.8041842377484));
#273025=CARTESIAN_POINT('Ctrl Pts',(5.47477154367344,-16.5701102199707,
54.1411460083266));
#273026=CARTESIAN_POINT('Ctrl Pts',(6.14788848420342,-17.1575471907001,
55.333062537043));
#273027=CARTESIAN_POINT('',(4.76104848420342,-15.0873905603315,50.0131411905777));
#273028=CARTESIAN_POINT('Ctrl Pts',(4.76104848420342,-15.0873905603315,
50.0131411905777));
#273029=CARTESIAN_POINT('Ctrl Pts',(4.76104848420342,-15.1514184267896,
50.1190782191899));
#273030=CARTESIAN_POINT('Ctrl Pts',(4.76253119975843,-15.2096066120234,
50.2285387691015));
#273031=CARTESIAN_POINT('Ctrl Pts',(4.76582464685242,-15.2616772101892,
50.3410866762893));
#273032=CARTESIAN_POINT('Ctrl Pts',(4.76903141935819,-15.3123774515448,
50.4506726280453));
#273033=CARTESIAN_POINT('Ctrl Pts',(4.77395531337918,-15.3572776080591,
50.5631854688987));
#273034=CARTESIAN_POINT('Ctrl Pts',(4.78086668106818,-15.3960965020952,
50.6781948156679));
#273035=CARTESIAN_POINT('Ctrl Pts',(4.78437582490208,-15.4158062164058,
50.736589095674));
#273036=CARTESIAN_POINT('Ctrl Pts',(4.78839676418632,-15.4339478375951,
50.7956265229538));
#273037=CARTESIAN_POINT('Ctrl Pts',(4.79296103895619,-15.4504823559191,
50.8552480699037));
#273038=CARTESIAN_POINT('',(4.76104848420342,-19.9972458266108,50.0131411905776));
#273039=CARTESIAN_POINT('Origin',(4.76104848420342,-17.542318193471,0.972561099047131));
#273040=CARTESIAN_POINT('',(4.79296103895619,-19.6341540310232,50.8552480699037));
#273041=CARTESIAN_POINT('Ctrl Pts',(4.79296103895619,-19.6341540310232,
50.8552480699037));
#273042=CARTESIAN_POINT('Ctrl Pts',(4.77035892158037,-19.7160323452691,
50.5600044068391));
#273043=CARTESIAN_POINT('Ctrl Pts',(4.76104848420342,-19.8379644323871,
50.2766795302212));
#273044=CARTESIAN_POINT('Ctrl Pts',(4.76104848420342,-19.9972458266108,
50.0131411905776));
#273045=CARTESIAN_POINT('Ctrl Pts',(6.14788848420341,-17.9270891962423,
55.333062537043));
#273046=CARTESIAN_POINT('Ctrl Pts',(6.12358695752485,-17.9482974207819,
55.2900307997962));
#273047=CARTESIAN_POINT('Ctrl Pts',(6.099576183545,-17.969450050515,55.2468069379304));
#273048=CARTESIAN_POINT('Ctrl Pts',(5.43709796638902,-18.558608728335,54.0342076324939));
#273049=CARTESIAN_POINT('Ctrl Pts',(5.01156238585603,-19.0785577539987,
52.7304461548518));
#273050=CARTESIAN_POINT('Ctrl Pts',(4.82218298524757,-19.5403257915009,
51.1870629797606));
#273051=CARTESIAN_POINT('Ctrl Pts',(4.80568122363092,-19.5880739553937,
51.0214074546985));
#273052=CARTESIAN_POINT('Ctrl Pts',(4.79296103895619,-19.6341540310232,
50.8552480699037));
#273053=CARTESIAN_POINT('Origin',(0.561048484203417,-17.542318193471,0.972561099047131));
#273054=CARTESIAN_POINT('',(10.1651884842034,-17.9270891962423,55.333062537043));
#273055=CARTESIAN_POINT('',(10.1651884842034,-17.1575471907001,55.333062537043));
#273056=CARTESIAN_POINT('Origin',(10.1651884842034,-17.542318193471,0.972561099047131));
#273057=CARTESIAN_POINT('',(8.15653848420341,-17.1575471907001,55.333062537043));
#273058=CARTESIAN_POINT('',(8.15653848420342,-17.9270891962423,55.333062537043));
#273059=CARTESIAN_POINT('Origin',(0.884028484203416,-17.542318193471,0.972561099047131));
#273060=CARTESIAN_POINT('',(11.5520284842034,-19.9972458266108,50.0131411905776));
#273061=CARTESIAN_POINT('',(11.5520284842034,-15.0873905603315,50.0131411905776));
#273062=CARTESIAN_POINT('Origin',(11.5520284842034,-17.542318193471,0.972561099047131));
#273063=CARTESIAN_POINT('',(11.520115929451,-15.4504823559191,50.8552480699037));
#273064=CARTESIAN_POINT('Ctrl Pts',(11.5201159294506,-15.4504823559191,
50.8552480699037));
#273065=CARTESIAN_POINT('Ctrl Pts',(11.5379482942249,-15.3858829229342,
50.6223100398281));
#273066=CARTESIAN_POINT('Ctrl Pts',(11.5475950755165,-15.296142243916,50.3960360842679));
#273067=CARTESIAN_POINT('Ctrl Pts',(11.5516325551658,-15.1520791771608,
50.123698661416));
#273068=CARTESIAN_POINT('Ctrl Pts',(11.5520284842034,-15.1204984263408,
50.0679196666184));
#273069=CARTESIAN_POINT('Ctrl Pts',(11.5520284842034,-15.0873905603315,
50.0131411905776));
#273070=CARTESIAN_POINT('Ctrl Pts',(10.1651884842034,-17.1575471907001,
55.333062537043));
#273071=CARTESIAN_POINT('Ctrl Pts',(10.189490010882,-17.1363389661605,55.2900307997962));
#273072=CARTESIAN_POINT('Ctrl Pts',(10.2135007848618,-17.1151863364273,
55.2468069379303));
#273073=CARTESIAN_POINT('Ctrl Pts',(10.8759790020178,-16.5260276586073,
54.0342076324939));
#273074=CARTESIAN_POINT('Ctrl Pts',(11.3015145825508,-16.0060786329436,
52.7304461548518));
#273075=CARTESIAN_POINT('Ctrl Pts',(11.4908939831593,-15.5443105954415,
51.1870629797606));
#273076=CARTESIAN_POINT('Ctrl Pts',(11.5073957447759,-15.4965624315486,
51.0214074546985));
#273077=CARTESIAN_POINT('Ctrl Pts',(11.5201159294506,-15.4504823559191,
50.8552480699037));
#273078=CARTESIAN_POINT('',(11.5201159294504,-19.6341540310232,50.8552480699037));
#273079=CARTESIAN_POINT('Ctrl Pts',(11.5201159294506,-19.6341540310232,
50.8552480699037));
#273080=CARTESIAN_POINT('Ctrl Pts',(11.5064953958128,-19.5848123558671,
51.0331684026437));
#273081=CARTESIAN_POINT('Ctrl Pts',(11.4885385348232,-19.5335560594093,
51.2105179282821));
#273082=CARTESIAN_POINT('Ctrl Pts',(11.2877548088084,-19.0542615562767,
52.8041842377484));
#273083=CARTESIAN_POINT('Ctrl Pts',(10.8383054247334,-18.5145261669716,
54.1411460083265));
#273084=CARTESIAN_POINT('Ctrl Pts',(10.1651884842034,-17.9270891962423,
55.333062537043));
#273085=CARTESIAN_POINT('Ctrl Pts',(11.5520284842034,-19.9972458266108,
50.0131411905776));
#273086=CARTESIAN_POINT('Ctrl Pts',(11.5520284842034,-19.9332179601523,
50.1190782191907));
#273087=CARTESIAN_POINT('Ctrl Pts',(11.5505457686484,-19.875029774918,50.2285387691031));
#273088=CARTESIAN_POINT('Ctrl Pts',(11.5472523215543,-19.822959176752,50.3410866762919));
#273089=CARTESIAN_POINT('Ctrl Pts',(11.5440455490485,-19.7722589353958,
50.4506726280492));
#273090=CARTESIAN_POINT('Ctrl Pts',(11.5391216550274,-19.7273587788812,
50.563185468904));
#273091=CARTESIAN_POINT('Ctrl Pts',(11.5322102873382,-19.6885398848448,
50.6781948156747));
#273092=CARTESIAN_POINT('Ctrl Pts',(11.5287011435044,-19.6688301705351,
50.7365890956786));
#273093=CARTESIAN_POINT('Ctrl Pts',(11.5246802042203,-19.6506885493466,
50.7956265229561));
#273094=CARTESIAN_POINT('Ctrl Pts',(11.5201159294506,-19.6341540310232,
50.8552480699037));
#273095=CARTESIAN_POINT('Origin',(19.4612584842034,-17.542318193471,0.972561099047131));
#273096=CARTESIAN_POINT('',(11.5520284842034,-9.08998123852178,3.49256109904713));
#273097=CARTESIAN_POINT('',(11.5520284842034,-9.08998123852178,-1.54743890095287));
#273098=CARTESIAN_POINT('Origin',(11.5520284842034,-17.542318193471,0.972561099047131));
#273099=CARTESIAN_POINT('',(-3.14818151579658,-9.08998123852178,-1.54743890095287));
#273100=CARTESIAN_POINT('',(19.4612584842034,-9.08998123852178,-1.54743890095287));
#273101=CARTESIAN_POINT('',(-3.14818151579658,-9.08998123852178,3.49256109904713));
#273102=CARTESIAN_POINT('Origin',(-3.14818151579658,-17.542318193471,0.972561099047131));
#273103=CARTESIAN_POINT('',(19.4612584842034,-9.08998123852178,3.49256109904713));
#273104=CARTESIAN_POINT('Origin',(11.5520284842034,-17.542318193471,0.972561099047131));
#273105=CARTESIAN_POINT('',(11.5520284842034,-25.3371465446544,49.451895009213));
#273106=CARTESIAN_POINT('Origin',(11.5520284842034,-22.8798040147369,51.7553464718149));
#273107=CARTESIAN_POINT('',(11.5520284842034,-30.1397096933157,48.4310786991304));
#273108=CARTESIAN_POINT('Origin',(11.5520284842034,-17.542318193471,0.972561099047131));
#273109=CARTESIAN_POINT('',(11.5520284842034,-35.2462311262942,46.7718693063201));
#273110=CARTESIAN_POINT('Origin',(11.5520284842034,-33.3215019147805,49.5358950681845));
#273111=CARTESIAN_POINT('',(11.5520284842034,-39.7316071024862,44.7748512573256));
#273112=CARTESIAN_POINT('Origin',(11.5520284842034,-17.542318193471,0.972561099047131));
#273113=CARTESIAN_POINT('',(11.5520284842034,-44.38156975997,42.0901940653056));
#273114=CARTESIAN_POINT('Origin',(11.5520284842034,-43.0735737692787,45.1939929373718));
#273115=CARTESIAN_POINT('',(11.5520284842034,-48.3537261103113,39.2042535488961));
#273116=CARTESIAN_POINT('Origin',(11.5520284842034,-17.542318193471,0.972561099047131));
#273117=CARTESIAN_POINT('',(11.5520284842034,-52.3439043111719,35.6114809593721));
#273118=CARTESIAN_POINT('Origin',(11.5520284842034,-51.7098072425573,38.9194020372514));
#273119=CARTESIAN_POINT('',(11.5520284842034,-55.6292387426316,31.9627474243937));
#273120=CARTESIAN_POINT('Origin',(11.5520284842034,-17.542318193471,0.972561099047131));
#273121=CARTESIAN_POINT('',(11.5520284842034,-58.7852425524921,27.6188808395635));
#273122=CARTESIAN_POINT('Origin',(11.5520284842034,-58.852757490588,30.9863520989862));
#273123=CARTESIAN_POINT('',(11.5520284842034,-61.2401701856317,23.3668214500608));
#273124=CARTESIAN_POINT('Origin',(11.5520284842034,-17.542318193471,0.972561099047131));
#273125=CARTESIAN_POINT('',(11.5520284842034,-63.4240670938147,18.461708683866));
#273126=CARTESIAN_POINT('Origin',(11.5520284842034,-64.1902433118537,21.7415554718754));
#273127=CARTESIAN_POINT('',(11.5520284842034,-64.9412958110163,13.792158838805));
#273128=CARTESIAN_POINT('Origin',(11.5520284842034,-17.542318193471,0.972561099047131));
#273129=CARTESIAN_POINT('',(11.5520284842034,-66.0576390431342,8.54017685647076));
#273130=CARTESIAN_POINT('Origin',(11.5520284842034,-67.4889909638665,11.5890541299798));
#273131=CARTESIAN_POINT('',(11.5520284842034,-66.5708586689849,3.65721829106678));
#273132=CARTESIAN_POINT('Origin',(11.5520284842034,-17.542318193471,0.972561099047131));
#273133=CARTESIAN_POINT('',(11.5520284842034,-66.5708586689849,-1.7120960929732));
#273134=CARTESIAN_POINT('Origin',(11.5520284842034,-68.604829345086,0.972561099046774));
#273135=CARTESIAN_POINT('',(11.5520284842034,-66.0576390431341,-6.59505465837716));
#273136=CARTESIAN_POINT('Origin',(11.5520284842034,-17.542318193471,0.972561099047131));
#273137=CARTESIAN_POINT('',(11.5520284842034,-64.9412958110161,-11.8470366407114));
#273138=CARTESIAN_POINT('Origin',(11.5520284842034,-67.4889909638663,-9.6439319318862));
#273139=CARTESIAN_POINT('Origin',(11.5520284842034,-17.542318193471,0.972561099047131));
#273140=CARTESIAN_POINT('Origin',(11.5520284842034,-17.542318193471,0.972561099047131));
#273141=CARTESIAN_POINT('Origin',(11.5520284842034,-17.542318193471,0.972561099047131));
#273142=CARTESIAN_POINT('Origin',(11.5520284842034,-17.542318193471,0.972561099047131));
#273143=CARTESIAN_POINT('Origin',(11.5520284842034,-17.542318193471,0.972561099047131));
#273144=CARTESIAN_POINT('Origin',(11.5520284842034,-17.542318193471,0.972561099047131));
#273145=CARTESIAN_POINT('Origin',(11.5520284842034,-17.542318193471,0.972561099047131));
#273146=CARTESIAN_POINT('Origin',(11.5520284842034,-17.542318193471,0.972561099047131));
#273147=CARTESIAN_POINT('Origin',(11.5520284842034,-17.542318193471,0.972561099047131));
#273148=CARTESIAN_POINT('Origin',(11.5520284842034,-17.542318193471,0.972561099047131));
#273149=CARTESIAN_POINT('Origin',(11.5520284842034,-17.542318193471,0.972561099047131));
#273150=CARTESIAN_POINT('Origin',(11.5520284842034,-17.542318193471,0.972561099047131));
#273151=CARTESIAN_POINT('',(11.5520284842034,29.8566594240744,-11.8470366407104));
#273152=CARTESIAN_POINT('Origin',(11.5520284842034,-17.542318193471,0.972561099047131));
#273153=CARTESIAN_POINT('',(11.5520284842034,30.9730026561922,-6.59505465837618));
#273154=CARTESIAN_POINT('Origin',(11.5520284842034,32.4043545769246,-9.6439319318852));
#273155=CARTESIAN_POINT('',(11.5520284842034,31.4862222820429,-1.71209609297287));
#273156=CARTESIAN_POINT('Origin',(11.5520284842034,-17.542318193471,0.972561099047131));
#273157=CARTESIAN_POINT('',(11.5520284842034,31.4862222820429,3.65721829106713));
#273158=CARTESIAN_POINT('Origin',(11.5520284842034,33.520192958144,0.972561099047131));
#273159=CARTESIAN_POINT('',(11.5520284842034,30.9730026561921,8.54017685647108));
#273160=CARTESIAN_POINT('Origin',(11.5520284842034,-17.542318193471,0.972561099047131));
#273161=CARTESIAN_POINT('',(11.5520284842034,29.8566594240743,13.7921588388053));
#273162=CARTESIAN_POINT('Origin',(11.5520284842034,32.4043545769244,11.5890541299801));
#273163=CARTESIAN_POINT('',(11.5520284842034,28.3394307068726,18.4617086838663));
#273164=CARTESIAN_POINT('Origin',(11.5520284842034,-17.542318193471,0.972561099047131));
#273165=CARTESIAN_POINT('',(11.5520284842034,26.1555337986896,23.3668214500611));
#273166=CARTESIAN_POINT('Origin',(11.5520284842034,29.1056069249115,21.7415554718757));
#273167=CARTESIAN_POINT('',(11.5520284842034,23.70060616555,27.6188808395637));
#273168=CARTESIAN_POINT('Origin',(11.5520284842034,-17.542318193471,0.972561099047131));
#273169=CARTESIAN_POINT('',(11.5520284842034,20.5446023556894,31.9627474243939));
#273170=CARTESIAN_POINT('Origin',(11.5520284842034,23.7681211036458,30.9863520989864));
#273171=CARTESIAN_POINT('',(11.5520284842034,17.2592679242297,35.6114809593723));
#273172=CARTESIAN_POINT('Origin',(11.5520284842034,-17.542318193471,0.972561099047131));
#273173=CARTESIAN_POINT('',(11.5520284842034,13.269089723369,39.2042535488963));
#273174=CARTESIAN_POINT('Origin',(11.5520284842034,16.6251708556151,38.9194020372516));
#273175=CARTESIAN_POINT('',(11.5520284842034,9.29693337302777,42.0901940653058));
#273176=CARTESIAN_POINT('Origin',(11.5520284842034,-17.542318193471,0.972561099047131));
#273177=CARTESIAN_POINT('',(11.5520284842034,4.64697071554394,44.7748512573258));
#273178=CARTESIAN_POINT('Origin',(11.5520284842034,7.98893738233642,45.193992937372));
#273179=CARTESIAN_POINT('',(11.5520284842034,0.161594739351914,46.7718693063202));
#273180=CARTESIAN_POINT('Origin',(11.5520284842034,-17.542318193471,0.972561099047131));
#273181=CARTESIAN_POINT('',(11.5520284842034,-4.94492669362662,48.4310786991304));
#273182=CARTESIAN_POINT('Origin',(11.5520284842034,-1.76313447216181,49.5358950681846));
#273183=CARTESIAN_POINT('',(11.5520284842034,-9.74748984228794,49.451895009213));
#273184=CARTESIAN_POINT('Origin',(11.5520284842034,-17.542318193471,0.972561099047131));
#273185=CARTESIAN_POINT('Origin',(11.5520284842034,-12.2048323722054,51.7553464718149));
#273186=CARTESIAN_POINT('',(11.5520284842034,-7.33631819347099,-1.54743890095287));
#273187=CARTESIAN_POINT('',(11.5520284842034,-17.542318193471,-1.54743890095287));
#273188=CARTESIAN_POINT('',(11.5520284842034,-7.33631819347099,3.49256109904713));
#273189=CARTESIAN_POINT('',(11.5520284842034,-17.542318193471,3.49256109904713));
#273190=CARTESIAN_POINT('',(11.5520284842034,-7.33631819347099,0.972561099047131));
#273191=CARTESIAN_POINT('Origin',(-3.14818151579658,-17.542318193471,0.972561099047131));
#273192=CARTESIAN_POINT('',(-3.14818151579658,-7.33631819347099,-1.54743890095287));
#273193=CARTESIAN_POINT('',(-3.14818151579658,-17.542318193471,-1.54743890095287));
#273194=CARTESIAN_POINT('',(-3.14818151579658,-7.33631819347099,3.49256109904713));
#273195=CARTESIAN_POINT('',(-3.14818151579658,-7.33631819347099,0.972561099047131));
#273196=CARTESIAN_POINT('',(-3.14818151579658,-17.542318193471,3.49256109904713));
#273197=CARTESIAN_POINT('Origin',(0.884028484203416,-17.542318193471,0.972561099047131));
#273198=CARTESIAN_POINT('',(10.1651884842034,-28.4681391279536,54.2251535450731));
#273199=CARTESIAN_POINT('',(11.5201159294506,-25.8673877784845,50.2001088036445));
#273200=CARTESIAN_POINT('Ctrl Pts',(10.1651884842034,-28.4681391279536,
54.2251535450731));
#273201=CARTESIAN_POINT('Ctrl Pts',(10.189490010882,-28.4384475527546,54.187471592353));
#273202=CARTESIAN_POINT('Ctrl Pts',(10.2135007848618,-28.4087704125277,
54.1495901545875));
#273203=CARTESIAN_POINT('Ctrl Pts',(10.8759790020178,-27.5803726934888,
53.0859820301889));
#273204=CARTESIAN_POINT('Ctrl Pts',(11.3015145825508,-26.8007185482924,
51.918814349969));
#273205=CARTESIAN_POINT('Ctrl Pts',(11.4908939831593,-26.0281538448012,
50.5051647736832));
#273206=CARTESIAN_POINT('Ctrl Pts',(11.5073957447759,-25.947007372541,50.3530566207839));
#273207=CARTESIAN_POINT('Ctrl Pts',(11.5201159294506,-25.8673877784845,
50.2001088036445));
#273208=CARTESIAN_POINT('',(10.1651884842034,-29.2208647943387,54.0651567655455));
#273209=CARTESIAN_POINT('Origin',(10.1651884842034,-17.542318193471,0.972561099047131));
#273210=CARTESIAN_POINT('',(11.5201159294509,-29.9596361897455,49.3302745518473));
#273211=CARTESIAN_POINT('Ctrl Pts',(11.5201159294506,-29.9596361897455,
49.3302745518472));
#273212=CARTESIAN_POINT('Ctrl Pts',(11.5064953958128,-29.9483644657862,
49.5145656095481));
#273213=CARTESIAN_POINT('Ctrl Pts',(11.4885385348232,-29.9351012821247,
49.6986964058043));
#273214=CARTESIAN_POINT('Ctrl Pts',(11.2877548088084,-29.7976223708411,
51.3571882133249));
#273215=CARTESIAN_POINT('Ctrl Pts',(10.8383054247334,-29.5476514770408,
52.7771514588734));
#273216=CARTESIAN_POINT('Ctrl Pts',(10.1651884842034,-29.2208647943387,
54.0651567655455));
#273217=CARTESIAN_POINT('Ctrl Pts',(11.5520284842034,-30.1397096933157,
48.4310786991304));
#273218=CARTESIAN_POINT('Ctrl Pts',(11.5520284842034,-30.0991044446738,
48.5480189146251));
#273219=CARTESIAN_POINT('Ctrl Pts',(11.5505456167773,-30.0649445445003,
48.6671915454817));
#273220=CARTESIAN_POINT('Ctrl Pts',(11.5472518253871,-30.0374111372518,
48.7881122473988));
#273221=CARTESIAN_POINT('Ctrl Pts',(11.5440447002134,-30.0106021888263,
48.905851284635));
#273222=CARTESIAN_POINT('Ctrl Pts',(11.5391202523756,-29.9900758384157,
49.025247456772));
#273223=CARTESIAN_POINT('Ctrl Pts',(11.5322080809733,-29.9760176360309,
49.1458213739011));
#273224=CARTESIAN_POINT('Ctrl Pts',(11.5286994596654,-29.9688816861871,
49.2070247483827));
#273225=CARTESIAN_POINT('Ctrl Pts',(11.5246792499256,-29.9634125828076,
49.2685310710613));
#273226=CARTESIAN_POINT('Ctrl Pts',(11.5201159294506,-29.9596361897455,
49.3302745518473));
#273227=CARTESIAN_POINT('Ctrl Pts',(11.5201159294506,-25.8673877784845,
50.2001088036445));
#273228=CARTESIAN_POINT('Ctrl Pts',(11.5379482942249,-25.7557694584127,
49.9856920057442));
#273229=CARTESIAN_POINT('Ctrl Pts',(11.5475950755165,-25.6209448278543,
49.7830208153142));
#273230=CARTESIAN_POINT('Ctrl Pts',(11.5516325551658,-25.4234077506953,
49.5465870143551));
#273231=CARTESIAN_POINT('Ctrl Pts',(11.5520284842034,-25.3809200099309,
49.4985929317228));
#273232=CARTESIAN_POINT('Ctrl Pts',(11.5520284842034,-25.3371465446544,
49.451895009213));
#273233=CARTESIAN_POINT('Origin',(0.884028484203416,-17.542318193471,0.972561099047131));
#273234=CARTESIAN_POINT('',(11.5201159294503,-9.21724860845784,50.2001088036446));
#273235=CARTESIAN_POINT('Ctrl Pts',(11.5520284842034,-9.74748984228794,
49.451895009213));
#273236=CARTESIAN_POINT('Ctrl Pts',(11.5520284842034,-9.66282867329459,
49.5422122981065));
#273237=CARTESIAN_POINT('Ctrl Pts',(11.5505455276575,-9.58314800677971,
49.6371907160474));
#273238=CARTESIAN_POINT('Ctrl Pts',(11.5472515368849,-9.50881029785681,
49.7364615046943));
#273239=CARTESIAN_POINT('Ctrl Pts',(11.5440442061737,-9.43642830492456,
49.833120624626));
#273240=CARTESIAN_POINT('Ctrl Pts',(11.5391194360271,-9.36911211034505,
49.9338491853251));
#273241=CARTESIAN_POINT('Ctrl Pts',(11.532206799365,-9.30722618613184,50.0382847362099));
#273242=CARTESIAN_POINT('Ctrl Pts',(11.52869848127,-9.27581769204343,50.0912881198434));
#273243=CARTESIAN_POINT('Ctrl Pts',(11.5246786952104,-9.24580837915736,
50.1452459945804));
#273244=CARTESIAN_POINT('Ctrl Pts',(11.5201159294506,-9.21724860845783,
50.2001088036446));
#273245=CARTESIAN_POINT('',(11.520115929451,-5.12500019719682,49.3302745518473));
#273246=CARTESIAN_POINT('Ctrl Pts',(11.5201159294506,-5.12500019719681,
49.3302745518473));
#273247=CARTESIAN_POINT('Ctrl Pts',(11.5379482942249,-5.11024295650262,
49.0889957992713));
#273248=CARTESIAN_POINT('Ctrl Pts',(11.5475950755165,-5.06950832732133,
48.8490083362216));
#273249=CARTESIAN_POINT('Ctrl Pts',(11.5516325551658,-4.98521551827838,
48.5526697436755));
#273250=CARTESIAN_POINT('Ctrl Pts',(11.5520284842034,-4.96592198775489,
48.4915436464428));
#273251=CARTESIAN_POINT('Ctrl Pts',(11.5520284842034,-4.94492669362662,
48.4310786991304));
#273252=CARTESIAN_POINT('',(10.1651884842034,-5.86377159260369,54.0651567655456));
#273253=CARTESIAN_POINT('Ctrl Pts',(10.1651884842034,-5.86377159260369,
54.0651567655456));
#273254=CARTESIAN_POINT('Ctrl Pts',(10.189490010882,-5.85197361990428,54.018655937179));
#273255=CARTESIAN_POINT('Ctrl Pts',(10.2135007848618,-5.84026997208577,
53.9719787413874));
#273256=CARTESIAN_POINT('Ctrl Pts',(10.8759790020178,-5.51609939680231,
52.6633846632577));
#273257=CARTESIAN_POINT('Ctrl Pts',(11.3015145825508,-5.27857975808516,
51.2800100209082));
#273258=CARTESIAN_POINT('Ctrl Pts',(11.4908939831593,-5.14778986561978,
49.6743464977371));
#273259=CARTESIAN_POINT('Ctrl Pts',(11.5073957447759,-5.1355268339775,49.5023835418609));
#273260=CARTESIAN_POINT('Ctrl Pts',(11.5201159294506,-5.12500019719682,
49.3302745518473));
#273261=CARTESIAN_POINT('',(10.1651884842034,-6.6164972589887,54.2251535450731));
#273262=CARTESIAN_POINT('Origin',(10.1651884842034,-17.542318193471,0.972561099047131));
#273263=CARTESIAN_POINT('Ctrl Pts',(11.5201159294506,-9.21724860845782,
50.2001088036446));
#273264=CARTESIAN_POINT('Ctrl Pts',(11.5064953958128,-9.13199345007686,
50.3638824391265));
#273265=CARTESIAN_POINT('Ctrl Pts',(11.4885385348232,-9.04498418693293,
50.5266996688594));
#273266=CARTESIAN_POINT('Ctrl Pts',(11.2877548088084,-8.24482156164845,
51.9858896152882));
#273267=CARTESIAN_POINT('Ctrl Pts',(10.8383054247334,-7.438910703289,53.1814182660674));
#273268=CARTESIAN_POINT('Ctrl Pts',(10.1651884842034,-6.61649725898869,
54.2251535450731));
#273269=CARTESIAN_POINT('Origin',(0.884028484203416,-17.542318193471,0.972561099047131));
#273270=CARTESIAN_POINT('',(11.5201159294502,0.835811325126388,47.3934894827125));
#273271=CARTESIAN_POINT('Ctrl Pts',(11.5520284842034,0.161594739351916,
46.7718693063203));
#273272=CARTESIAN_POINT('Ctrl Pts',(11.5520284842034,0.2631850069628,46.8426116844753));
#273273=CARTESIAN_POINT('Ctrl Pts',(11.5505454949276,0.360872606771722,
46.918948942952));
#273274=CARTESIAN_POINT('Ctrl Pts',(11.5472514286422,0.454226339726327,
47.0005957533459));
#273275=CARTESIAN_POINT('Ctrl Pts',(11.5440440212228,0.545124163197585,
47.0800946348934));
#273276=CARTESIAN_POINT('Ctrl Pts',(11.539119130386,0.631912869753242,47.1646273892785));
#273277=CARTESIAN_POINT('Ctrl Pts',(11.5322063173428,0.714160596297907,
47.2539152743948));
#273278=CARTESIAN_POINT('Ctrl Pts',(11.5286981135811,0.755900736215872,
47.2992282450301));
#273279=CARTESIAN_POINT('Ctrl Pts',(11.5246784869495,0.796470830265539,
47.3457656462573));
#273280=CARTESIAN_POINT('Ctrl Pts',(11.5201159294506,0.8358113251264,47.3934894827125));
#273281=CARTESIAN_POINT('',(11.520115929451,4.65778558018571,45.6918369098494));
#273282=CARTESIAN_POINT('Ctrl Pts',(11.5201159294506,4.65778558018571,45.6918369098493));
#273283=CARTESIAN_POINT('Ctrl Pts',(11.5379482942249,4.62205566635771,45.4527624740445));
#273284=CARTESIAN_POINT('Ctrl Pts',(11.5475950755165,4.6120039469405,45.2095501072284));
#273285=CARTESIAN_POINT('Ctrl Pts',(11.5516325551658,4.63284249803413,44.9021617634728));
#273286=CARTESIAN_POINT('Ctrl Pts',(11.5520284842034,4.63900558839659,44.8383600675693));
#273287=CARTESIAN_POINT('Ctrl Pts',(11.5520284842034,4.64697071554394,44.7748512573258));
#273288=CARTESIAN_POINT('',(10.1651884842034,4.91959547915064,50.4768497968823));
#273289=CARTESIAN_POINT('Ctrl Pts',(10.1651884842034,4.91959547915065,50.4768497968823));
#273290=CARTESIAN_POINT('Ctrl Pts',(10.189490010882,4.92146757198998,50.4289121867312));
#273291=CARTESIAN_POINT('Ctrl Pts',(10.2135007848618,4.9232107323238,50.380821674452));
#273292=CARTESIAN_POINT('Ctrl Pts',(10.8759790020178,4.96822539538776,49.0334246641745));
#273293=CARTESIAN_POINT('Ctrl Pts',(11.3015145825508,4.91293489920084,47.6308969671562));
#273294=CARTESIAN_POINT('Ctrl Pts',(11.4908939831593,4.70703050072919,46.0331282966963));
#273295=CARTESIAN_POINT('Ctrl Pts',(11.5073957447759,4.68327244679356,45.8623735163476));
#273296=CARTESIAN_POINT('Ctrl Pts',(11.5201159294506,4.65778558018571,45.6918369098494));
#273297=CARTESIAN_POINT('',(10.1651884842034,4.21658387552238,50.7898507289224));
#273298=CARTESIAN_POINT('Origin',(10.1651884842034,-17.542318193471,0.972561099047131));
#273299=CARTESIAN_POINT('Ctrl Pts',(11.5201159294506,0.83581132512641,47.3934894827125));
#273300=CARTESIAN_POINT('Ctrl Pts',(11.5064953958128,0.953253907211338,
47.5359587271927));
#273301=CARTESIAN_POINT('Ctrl Pts',(11.4885385348232,1.07221341472524,47.677127766797));
#273302=CARTESIAN_POINT('Ctrl Pts',(11.2877548088084,2.15827321583037,48.9380677475591));
#273303=CARTESIAN_POINT('Ctrl Pts',(10.8383054247334,3.19513737154455,49.9399129397174));
#273304=CARTESIAN_POINT('Ctrl Pts',(10.1651884842034,4.21658387552238,50.7898507289224));
#273305=CARTESIAN_POINT('Origin',(0.884028484203416,-17.542318193471,0.972561099047131));
#273306=CARTESIAN_POINT('',(11.5201159294502,10.0856588106982,42.5580528390859));
#273307=CARTESIAN_POINT('Ctrl Pts',(11.5520284842034,9.29693337302777,42.0901940653058));
#273308=CARTESIAN_POINT('Ctrl Pts',(11.5520284842034,9.41101218010821,42.1382689014774));
#273309=CARTESIAN_POINT('Ctrl Pts',(11.5505454855484,9.52243682315436,42.19262780338));
#273310=CARTESIAN_POINT('Ctrl Pts',(11.5472513973454,9.63072620391565,42.2530813329829));
#273311=CARTESIAN_POINT('Ctrl Pts',(11.5440439677956,9.73616678060244,42.3119444918565));
#273312=CARTESIAN_POINT('Ctrl Pts',(11.5391190420917,9.83863461622702,42.3765858961965));
#273313=CARTESIAN_POINT('Ctrl Pts',(11.5322061778343,9.93764933154213,42.4468226877339));
#273314=CARTESIAN_POINT('Ctrl Pts',(11.5286980071981,9.98789775302051,42.4824667623872));
#273315=CARTESIAN_POINT('Ctrl Pts',(11.5246784267181,10.0372562954908,42.5195517400329));
#273316=CARTESIAN_POINT('Ctrl Pts',(11.5201159294506,10.0856588106982,42.5580528390859));
#273317=CARTESIAN_POINT('',(11.520115929451,13.4703202947425,40.098952328026));
#273318=CARTESIAN_POINT('Ctrl Pts',(11.5201159294506,13.4703202947425,40.0989523280259));
#273319=CARTESIAN_POINT('Ctrl Pts',(11.5379482942249,13.3856647950777,39.8725309090435));
#273320=CARTESIAN_POINT('Ctrl Pts',(11.5475950755165,13.325266035434,39.6367231859533));
#273321=CARTESIAN_POINT('Ctrl Pts',(11.5516325551658,13.2817395839011,39.3317194366231));
#273322=CARTESIAN_POINT('Ctrl Pts',(11.5520284842034,13.2745028774799,39.2680305823144));
#273323=CARTESIAN_POINT('Ctrl Pts',(11.5520284842034,13.2690897233691,39.2042535488963));
#273324=CARTESIAN_POINT('',(10.1651884842034,14.7212691391912,44.7249678641909));
#273325=CARTESIAN_POINT('Ctrl Pts',(10.1651884842034,14.7212691391912,44.7249678641909));
#273326=CARTESIAN_POINT('Ctrl Pts',(10.189490010882,14.71313353273,44.6776885758492));
#273327=CARTESIAN_POINT('Ctrl Pts',(10.2135007848618,14.704840021108,44.6302865332328));
#273328=CARTESIAN_POINT('Ctrl Pts',(10.8759790020178,14.4687314151723,43.3029743056847));
#273329=CARTESIAN_POINT('Ctrl Pts',(11.3015145825508,14.1230472440778,41.9425907444319));
#273330=CARTESIAN_POINT('Ctrl Pts',(11.4908939831593,13.5894475649212,40.422547084527));
#273331=CARTESIAN_POINT('Ctrl Pts',(11.5073957447759,13.5307067663685,40.2604632829794));
#273332=CARTESIAN_POINT('Ctrl Pts',(11.5201159294506,13.4703202947424,40.0989523280259));
#273333=CARTESIAN_POINT('',(10.1651884842034,14.0986965788221,45.1772933060682));
#273334=CARTESIAN_POINT('Origin',(10.1651884842034,-17.542318193471,0.972561099047131));
#273335=CARTESIAN_POINT('Ctrl Pts',(11.5201159294506,10.0856588106982,42.5580528390859));
#273336=CARTESIAN_POINT('Ctrl Pts',(11.5064953958128,10.2301560120979,42.6729911029372));
#273337=CARTESIAN_POINT('Ctrl Pts',(11.4885385348232,10.3758666626724,42.786342187978));
#273338=CARTESIAN_POINT('Ctrl Pts',(11.2877548088084,11.7003576147968,43.7939230752528));
#273339=CARTESIAN_POINT('Ctrl Pts',(10.8383054247334,12.9228591288348,44.5582993665063));
#273340=CARTESIAN_POINT('Ctrl Pts',(10.1651884842034,14.0986965788221,45.1772933060682));
#273341=CARTESIAN_POINT('Origin',(0.884028484203416,-17.542318193471,0.972561099047131));
#273342=CARTESIAN_POINT('',(10.1651884842034,29.7276425156794,27.8195903550057));
#273343=CARTESIAN_POINT('',(11.5201159294506,26.7032738510938,24.1023216086087));
#273344=CARTESIAN_POINT('Ctrl Pts',(10.1651884842034,29.7276425156794,27.8195903550057));
#273345=CARTESIAN_POINT('Ctrl Pts',(10.189490010882,29.7009800503245,27.7797076251619));
#273346=CARTESIAN_POINT('Ctrl Pts',(10.2135007848618,29.6741234027656,27.7397769795232));
#273347=CARTESIAN_POINT('Ctrl Pts',(10.8759790020178,28.9185609385563,26.6232509449527));
#273348=CARTESIAN_POINT('Ctrl Pts',(11.3015145825508,28.0494448912745,25.521081141234));
#273349=CARTESIAN_POINT('Ctrl Pts',(11.4908939831593,26.9437198726232,24.3494867025559));
#273350=CARTESIAN_POINT('Ctrl Pts',(11.5073957447759,26.8241320615886,24.2253078171096));
#273351=CARTESIAN_POINT('Ctrl Pts',(11.5201159294506,26.7032738510938,24.1023216086087));
#273352=CARTESIAN_POINT('',(10.1651884842034,29.3428715129083,28.4860332810845));
#273353=CARTESIAN_POINT('Origin',(10.1651884842034,-17.542318193471,0.972561099047131));
#273354=CARTESIAN_POINT('',(11.5201159294504,24.6114380135418,27.7254875603422));
#273355=CARTESIAN_POINT('Ctrl Pts',(11.5201159294506,24.6114380135418,27.7254875603422));
#273356=CARTESIAN_POINT('Ctrl Pts',(11.5064953958128,24.7901923791225,27.7717165825618));
#273357=CARTESIAN_POINT('Ctrl Pts',(11.4885385348232,24.9694097219034,27.8160020905446));
#273358=CARTESIAN_POINT('Ctrl Pts',(11.2877548088084,26.5892124826229,28.1977540296707));
#273359=CARTESIAN_POINT('Ctrl Pts',(10.8383054247334,28.0169230344847,28.3988103565001));
#273360=CARTESIAN_POINT('Ctrl Pts',(10.1651884842034,29.3428715129083,28.4860332810845));
#273361=CARTESIAN_POINT('Ctrl Pts',(11.5520284842034,23.7006061655499,27.6188808395637));
#273362=CARTESIAN_POINT('Ctrl Pts',(11.5520284842034,23.8243746910238,27.6163993857689));
#273363=CARTESIAN_POINT('Ctrl Pts',(11.5505455200547,23.9482745265803,27.6207381048773));
#273364=CARTESIAN_POINT('Ctrl Pts',(11.547251509512,24.0717890993467,27.631919614997));
#273365=CARTESIAN_POINT('Ctrl Pts',(11.544044159792,24.1920541759846,27.6428069551817));
#273366=CARTESIAN_POINT('Ctrl Pts',(11.5391193593529,24.311953775325,27.6601819444671));
#273367=CARTESIAN_POINT('Ctrl Pts',(11.5322066763546,24.4309746622713,27.6840729200195));
#273368=CARTESIAN_POINT('Ctrl Pts',(11.5286983877109,24.4913795189887,27.6961979427118));
#273369=CARTESIAN_POINT('Ctrl Pts',(11.5246786424116,24.5515574771146,27.7100014006615));
#273370=CARTESIAN_POINT('Ctrl Pts',(11.5201159294506,24.6114380135418,27.7254875603422));
#273371=CARTESIAN_POINT('Ctrl Pts',(11.5201159294506,26.7032738510938,24.1023216086087));
#273372=CARTESIAN_POINT('Ctrl Pts',(11.5379482942249,26.5338433160333,23.9299078435359));
#273373=CARTESIAN_POINT('Ctrl Pts',(11.5475950755165,26.3827546618124,23.7390531579732));
#273374=CARTESIAN_POINT('Ctrl Pts',(11.5516325551658,26.218935068599,23.47812217099));
#273375=CARTESIAN_POINT('Ctrl Pts',(11.5520284842034,26.1864194175169,23.4228829411106));
#273376=CARTESIAN_POINT('Ctrl Pts',(11.5520284842034,26.1555337986896,23.3668214500611));
#273377=CARTESIAN_POINT('Origin',(0.884028484203416,-17.542318193471,0.972561099047131));
#273378=CARTESIAN_POINT('Ctrl Pts',(11.5520284842034,28.3394307068726,18.4617086838663));
#273379=CARTESIAN_POINT('Ctrl Pts',(11.5520284842034,28.4599764800091,18.4335490439404));
#273380=CARTESIAN_POINT('Ctrl Pts',(11.5505455736236,28.5820687040887,18.4120329930338));
#273381=CARTESIAN_POINT('Ctrl Pts',(11.5472516844235,28.7052067728467,18.3972900560855));
#273382=CARTESIAN_POINT('Ctrl Pts',(11.544044459049,28.8251050191691,18.3829350129735));
#273383=CARTESIAN_POINT('Ctrl Pts',(11.539119853862,28.9459946217007,18.3750015769573));
#273384=CARTESIAN_POINT('Ctrl Pts',(11.5322074541281,29.067379435199,18.3736241726326));
#273385=CARTESIAN_POINT('Ctrl Pts',(11.528698981281,29.1289897787257,18.3729250542571));
#273386=CARTESIAN_POINT('Ctrl Pts',(11.5246789788102,29.1907271647795,18.3739151171815));
#273387=CARTESIAN_POINT('Ctrl Pts',(11.5201159294506,29.2525234772274,18.3766132024512));
#273388=CARTESIAN_POINT('',(11.5201159294506,30.5453491237196,14.397704993804));
#273389=CARTESIAN_POINT('Ctrl Pts',(11.5201159294506,30.5453491237196,14.397704993804));
#273390=CARTESIAN_POINT('Ctrl Pts',(11.5379482942249,30.3437742149424,14.264285472185));
#273391=CARTESIAN_POINT('Ctrl Pts',(11.5475950755165,30.1563062899423,14.1090145169754));
#273392=CARTESIAN_POINT('Ctrl Pts',(11.5516325551658,29.9418159451973,13.887845506715));
#273393=CARTESIAN_POINT('Ctrl Pts',(11.5520284842034,29.8985259574212,13.8405737705366));
#273394=CARTESIAN_POINT('Ctrl Pts',(11.5520284842034,29.8566594240743,13.7921588388053));
#273395=CARTESIAN_POINT('',(10.1651884842034,34.2764917070059,17.4049408966648));
#273396=CARTESIAN_POINT('Ctrl Pts',(10.1651884842034,34.2764917070059,17.4049408966648));
#273397=CARTESIAN_POINT('Ctrl Pts',(10.189490010882,34.2421197946932,17.3714731384106));
#273398=CARTESIAN_POINT('Ctrl Pts',(10.2135007848618,34.2075479812695,17.337998884187));
#273399=CARTESIAN_POINT('Ctrl Pts',(10.8759790020178,33.236357554009,16.4029618917673));
#273400=CARTESIAN_POINT('Ctrl Pts',(11.3015145825508,32.1570797901417,15.5055765295658));
#273401=CARTESIAN_POINT('Ctrl Pts',(11.4908939831593,30.8319293353782,14.589477398547));
#273402=CARTESIAN_POINT('Ctrl Pts',(11.5073957447759,30.6891365629007,14.4928758236793));
#273403=CARTESIAN_POINT('Ctrl Pts',(11.5201159294506,30.5453491237196,14.397704993804));
#273404=CARTESIAN_POINT('Origin',(10.1651884842034,-17.542318193471,0.972561099047131));
#273405=CARTESIAN_POINT('Origin',(0.884028484203416,-17.542318193471,0.972561099047131));
#273406=CARTESIAN_POINT('',(11.5201159294503,18.1280311274453,35.9051306570905));
#273407=CARTESIAN_POINT('Ctrl Pts',(11.5520284842034,17.2592679242297,35.6114809593723));
#273408=CARTESIAN_POINT('Ctrl Pts',(11.5520284842034,17.3808488290273,35.6347868646574));
#273409=CARTESIAN_POINT('Ctrl Pts',(11.5505454934864,17.5011401217583,35.6647913142035));
#273410=CARTESIAN_POINT('Ctrl Pts',(11.5472514229156,17.6196318266977,35.7014090350157));
#273411=CARTESIAN_POINT('Ctrl Pts',(11.5440440116058,17.7350062931456,35.7370634295862));
#273412=CARTESIAN_POINT('Ctrl Pts',(11.5391191144822,17.8486743622293,35.7789878343029));
#273413=CARTESIAN_POINT('Ctrl Pts',(11.5322062913615,17.9601281306309,35.8271032630006));
#273414=CARTESIAN_POINT('Ctrl Pts',(11.5286980938805,18.0166899466528,35.8515214236859));
#273415=CARTESIAN_POINT('Ctrl Pts',(11.5246784758745,18.0726808983853,35.8775340508797));
#273416=CARTESIAN_POINT('Ctrl Pts',(11.5201159294506,18.1280311274453,35.9051306570905));
#273417=CARTESIAN_POINT('',(11.5201159294502,20.927453892214,32.7960567002406));
#273418=CARTESIAN_POINT('Ctrl Pts',(11.5201159294506,20.927453892214,32.7960567002406));
#273419=CARTESIAN_POINT('Ctrl Pts',(11.5379482942249,20.7975726582702,32.5921840005807));
#273420=CARTESIAN_POINT('Ctrl Pts',(11.5475950755165,20.6894665740218,32.3740868502464));
#273421=CARTESIAN_POINT('Ctrl Pts',(11.5516325551658,20.5834774346573,32.0847978227575));
#273422=CARTESIAN_POINT('Ctrl Pts',(11.5520284842034,20.5631572102486,32.0240053185899));
#273423=CARTESIAN_POINT('Ctrl Pts',(11.5520284842034,20.5446023556894,31.9627474243939));
#273424=CARTESIAN_POINT('',(10.1651884842034,23.1128692149255,37.0608958085218));
#273425=CARTESIAN_POINT('Ctrl Pts',(10.1651884842034,23.1128692149255,37.0608958085218));
#273426=CARTESIAN_POINT('Ctrl Pts',(10.189490010882,23.0950814742053,37.0163411737611));
#273427=CARTESIAN_POINT('Ctrl Pts',(10.2135007848618,23.0771137568819,36.9716992975302));
#273428=CARTESIAN_POINT('Ctrl Pts',(10.8759790020178,22.5702009610007,35.722481766206));
#273429=CARTESIAN_POINT('Ctrl Pts',(11.3015145825508,21.9492311720522,34.4636976301901));
#273430=CARTESIAN_POINT('Ctrl Pts',(11.4908939831593,21.1112570786853,33.0878121827568));
#273431=CARTESIAN_POINT('Ctrl Pts',(11.5073957447759,21.0201007902818,32.9414831999023));
#273432=CARTESIAN_POINT('Ctrl Pts',(11.5201159294506,20.927453892214,32.7960567002406));
#273433=CARTESIAN_POINT('',(10.1651884842034,22.5979451061385,37.632776967928));
#273434=CARTESIAN_POINT('Origin',(10.1651884842034,-17.542318193471,0.972561099047131));
#273435=CARTESIAN_POINT('Ctrl Pts',(11.5201159294506,18.1280311274453,35.9051306570905));
#273436=CARTESIAN_POINT('Ctrl Pts',(11.5064953958128,18.2932677270842,35.9875145866478));
#273437=CARTESIAN_POINT('Ctrl Pts',(11.4885385348232,18.4593612660918,36.0680937307899));
#273438=CARTESIAN_POINT('Ctrl Pts',(11.2877548088084,19.9643967590149,36.778279404894));
#273439=CARTESIAN_POINT('Ctrl Pts',(10.8383054247334,21.3191064490001,37.2717798834305));
#273440=CARTESIAN_POINT('Ctrl Pts',(10.1651884842034,22.5979451061385,37.632776967928));
#273441=CARTESIAN_POINT('Origin',(0.884028484203416,-17.542318193471,0.972561099047131));
#273442=CARTESIAN_POINT('',(10.1651884842034,-71.6452466383859,-4.32699539176734));
#273443=CARTESIAN_POINT('',(11.5201159294503,-67.370398971297,-2.16122297171674));
#273444=CARTESIAN_POINT('Ctrl Pts',(10.1651884842034,-71.6452466383859,
-4.32699539176736));
#273445=CARTESIAN_POINT('Ctrl Pts',(10.189490010882,-71.604667496618,-4.30140530673472));
#273446=CARTESIAN_POINT('Ctrl Pts',(10.2135007848618,-71.5638914714702,
-4.27585042946313));
#273447=CARTESIAN_POINT('Ctrl Pts',(10.8759790020178,-70.4195187631186,
-3.56316808256816));
#273448=CARTESIAN_POINT('Ctrl Pts',(11.3015145825508,-69.177248899896,-2.90978720834477));
#273449=CARTESIAN_POINT('Ctrl Pts',(11.4908939831593,-67.690588442671,-2.28922131294222));
#273450=CARTESIAN_POINT('Ctrl Pts',(11.5073957447759,-67.5308314381036,
-2.22441900102061));
#273451=CARTESIAN_POINT('Ctrl Pts',(11.5201159294506,-67.370398971297,-2.16122297171675));
#273452=CARTESIAN_POINT('',(10.1651884842034,-71.5648075951267,-5.09232176568469));
#273453=CARTESIAN_POINT('Origin',(10.1651884842034,-17.542318193471,0.972561099047131));
#273454=CARTESIAN_POINT('',(11.5201159294504,-66.9330862002819,-6.32197605563978));
#273455=CARTESIAN_POINT('Ctrl Pts',(11.5201159294506,-66.933086200282,-6.32197605563978));
#273456=CARTESIAN_POINT('Ctrl Pts',(11.5064953958128,-67.1151894763022,
-6.29150241830828));
#273457=CARTESIAN_POINT('Ctrl Pts',(11.4885385348232,-67.2969252045844,
-6.25906498258172));
#273458=CARTESIAN_POINT('Ctrl Pts',(11.2877548088084,-68.9319611611244,
-5.94897959517663));
#273459=CARTESIAN_POINT('Ctrl Pts',(10.8383054247334,-70.3180166260499,
-5.55195149213379));
#273460=CARTESIAN_POINT('Ctrl Pts',(10.1651884842034,-71.5648075951267,
-5.0923217656847));
#273461=CARTESIAN_POINT('Ctrl Pts',(11.5520284842034,-66.0576390431341,
-6.59505465837715));
#273462=CARTESIAN_POINT('Ctrl Pts',(11.5520284842034,-66.1696919168509,
-6.54244936087575));
#273463=CARTESIAN_POINT('Ctrl Pts',(11.5505456780052,-66.2846386577793,
-6.49602047434678));
#273464=CARTESIAN_POINT('Ctrl Pts',(11.5472520254149,-66.4020164824461,
-6.45599878354303));
#273465=CARTESIAN_POINT('Ctrl Pts',(11.5440450424203,-66.5163056120188,
-6.41703022863092));
#273466=CARTESIAN_POINT('Ctrl Pts',(11.5391208178552,-66.6328994339461,
-6.3841363514087));
#273467=CARTESIAN_POINT('Ctrl Pts',(11.532208970468,-66.7513405603435,-6.35755179799039));
#273468=CARTESIAN_POINT('Ctrl Pts',(11.5287001384983,-66.8114677575395,
-6.34405602389257));
#273469=CARTESIAN_POINT('Ctrl Pts',(11.5246796346431,-66.8720705537274,
-6.332186573129));
#273470=CARTESIAN_POINT('Ctrl Pts',(11.5201159294506,-66.9330862002819,
-6.32197605563978));
#273471=CARTESIAN_POINT('Ctrl Pts',(11.5201159294506,-67.370398971297,-2.16122297171675));
#273472=CARTESIAN_POINT('Ctrl Pts',(11.5379482942249,-67.1454894795807,
-2.07262876686444));
#273473=CARTESIAN_POINT('Ctrl Pts',(11.5475950755165,-66.9298355316947,
-1.95972762782341));
#273474=CARTESIAN_POINT('Ctrl Pts',(11.5516325551658,-66.674048692722,-1.78798674132045));
#273475=CARTESIAN_POINT('Ctrl Pts',(11.5520284842034,-66.6218763484463,
-1.750748500549));
#273476=CARTESIAN_POINT('Ctrl Pts',(11.5520284842034,-66.5708586689849,
-1.71209609297321));
#273477=CARTESIAN_POINT('Origin',(0.884028484203416,-17.542318193471,0.972561099047131));
#273478=CARTESIAN_POINT('',(11.5201159294509,-67.370398971297,4.1063451698103));
#273479=CARTESIAN_POINT('Ctrl Pts',(11.5520284842034,-66.5708586689849,
3.65721829106678));
#273480=CARTESIAN_POINT('Ctrl Pts',(11.5520284842034,-66.6695318325109,
3.73197581382481));
#273481=CARTESIAN_POINT('Ctrl Pts',(11.5505454936051,-66.7723200664417,
3.80129276827458));
#273482=CARTESIAN_POINT('Ctrl Pts',(11.5472514232079,-66.8788187601877,
3.86484722697449));
#273483=CARTESIAN_POINT('Ctrl Pts',(11.5440440121231,-66.98251572159,3.92672971603551));
#273484=CARTESIAN_POINT('Ctrl Pts',(11.5391191153365,-67.0897304064872,
3.98314865000039));
#273485=CARTESIAN_POINT('Ctrl Pts',(11.5322062926153,-67.200064263055,4.03377943485101));
#273486=CARTESIAN_POINT('Ctrl Pts',(11.5286980948493,-67.2560577413694,
4.05947412043318));
#273487=CARTESIAN_POINT('Ctrl Pts',(11.524678476432,-67.312854156827,4.08367766457325));
#273488=CARTESIAN_POINT('Ctrl Pts',(11.5201159294506,-67.370398971297,4.1063451698103));
#273489=CARTESIAN_POINT('',(11.5201159294503,-66.933086200282,8.26709825373337));
#273490=CARTESIAN_POINT('Ctrl Pts',(11.5201159294506,-66.9330862002821,
8.26709825373337));
#273491=CARTESIAN_POINT('Ctrl Pts',(11.5379482942249,-66.6946717496501,
8.30699514994484));
#273492=CARTESIAN_POINT('Ctrl Pts',(11.5475950755165,-66.4602568912234,
8.37259215128143));
#273493=CARTESIAN_POINT('Ctrl Pts',(11.5516325551658,-66.1743526702874,
8.4873990131825));
#273494=CARTESIAN_POINT('Ctrl Pts',(11.5520284842034,-66.1155781513076,
8.51297626873635));
#273495=CARTESIAN_POINT('Ctrl Pts',(11.5520284842034,-66.0576390431342,
8.54017685647076));
#273496=CARTESIAN_POINT('',(10.1651884842034,-71.5648075951268,7.03744396377821));
#273497=CARTESIAN_POINT('Ctrl Pts',(10.1651884842034,-71.5648075951268,
7.03744396377821));
#273498=CARTESIAN_POINT('Ctrl Pts',(10.189490010882,-71.5197947271194,7.05403796607858));
#273499=CARTESIAN_POINT('Ctrl Pts',(10.2135007848618,-71.4745965982113,
7.07055659563549));
#273500=CARTESIAN_POINT('Ctrl Pts',(10.8759790020178,-70.2070561874331,
7.52973665861706));
#273501=CARTESIAN_POINT('Ctrl Pts',(11.3015145825508,-68.8560873789502,
7.91055716538948));
#273502=CARTESIAN_POINT('Ctrl Pts',(11.4908939831593,-67.2728911150328,
8.20846811774117));
#273503=CARTESIAN_POINT('Ctrl Pts',(11.5073957447759,-67.1031520260743,
8.23863899472971));
#273504=CARTESIAN_POINT('Ctrl Pts',(11.5201159294506,-66.9330862002821,
8.26709825373337));
#273505=CARTESIAN_POINT('',(10.1651884842034,-71.645246638386,6.27211758986086));
#273506=CARTESIAN_POINT('Origin',(10.1651884842034,-17.542318193471,0.972561099047131));
#273507=CARTESIAN_POINT('Ctrl Pts',(11.5201159294507,-67.370398971297,4.10634516981029));
#273508=CARTESIAN_POINT('Ctrl Pts',(11.5064953958128,-67.5421870283591,
4.17401428507257));
#273509=CARTESIAN_POINT('Ctrl Pts',(11.4885385348232,-67.7132072728382,
4.24352786755159));
#273510=CARTESIAN_POINT('Ctrl Pts',(11.2877548088084,-69.2480433936481,
4.88678023553657));
#273511=CARTESIAN_POINT('Ctrl Pts',(10.8383054247334,-70.5212634369431,
5.5633094572317));
#273512=CARTESIAN_POINT('Ctrl Pts',(10.1651884842034,-71.645246638386,6.27211758986087));
#273513=CARTESIAN_POINT('Origin',(0.884028484203416,-17.542318193471,0.972561099047131));
#273514=CARTESIAN_POINT('',(11.5201159294503,-65.6299855106617,14.3977049938037));
#273515=CARTESIAN_POINT('Ctrl Pts',(11.5520284842034,-64.9412958110163,
13.792158838805));
#273516=CARTESIAN_POINT('Ctrl Pts',(11.5520284842034,-65.0222693835792,
13.8857975921066));
#273517=CARTESIAN_POINT('Ctrl Pts',(11.5505455075224,-65.1083992116548,
13.9749702764953));
#273518=CARTESIAN_POINT('Ctrl Pts',(11.5472514703206,-65.1993564521249,
14.0592778788253));
#273519=CARTESIAN_POINT('Ctrl Pts',(11.544044092433,-65.287920795488,14.1413675222917));
#273520=CARTESIAN_POINT('Ctrl Pts',(11.539119248065,-65.3810618737815,14.2188444200145));
#273521=CARTESIAN_POINT('Ctrl Pts',(11.5322065029564,-65.4784573259309,
14.2913082108836));
#273522=CARTESIAN_POINT('Ctrl Pts',(11.5286982551647,-65.5278859356303,
14.3280838955502));
#273523=CARTESIAN_POINT('Ctrl Pts',(11.5246785671409,-65.5784100024307,
14.3635679095943));
#273524=CARTESIAN_POINT('Ctrl Pts',(11.5201159294506,-65.6299855106617,
14.3977049938037));
#273525=CARTESIAN_POINT('Ctrl Pts',(11.5201159294506,-64.3371598641694,
18.3766132024509));
#273526=CARTESIAN_POINT('Ctrl Pts',(11.5379482942249,-64.095660310154,18.3660691042106));
#273527=CARTESIAN_POINT('Ctrl Pts',(11.5475950755165,-63.8527295953472,
18.381495064115));
#273528=CARTESIAN_POINT('Ctrl Pts',(11.5516325551658,-63.5492033788236,
18.4343502906445));
#273529=CARTESIAN_POINT('Ctrl Pts',(11.5520284842034,-63.4863954136504,
18.4471487121798));
#273530=CARTESIAN_POINT('Ctrl Pts',(11.5520284842034,-63.4240670938147,
18.461708683866));
#273531=CARTESIAN_POINT('',(10.1651884842034,-69.361128093948,17.4049408966644));
#273532=CARTESIAN_POINT('Origin',(10.1651884842034,-17.542318193471,0.972561099047131));
#273533=CARTESIAN_POINT('Ctrl Pts',(11.5201159294506,-65.6299855106617,
14.3977049938037));
#273534=CARTESIAN_POINT('Ctrl Pts',(11.5064953958128,-65.7839503863413,
14.4996121219473));
#273535=CARTESIAN_POINT('Ctrl Pts',(11.4885385348232,-65.9367807416874,
14.6031637740613));
#273536=CARTESIAN_POINT('Ctrl Pts',(11.2877548088084,-67.3043373233269,
15.5514699074779));
#273537=CARTESIAN_POINT('Ctrl Pts',(10.8383054247334,-68.4090761195119,
16.4779326744898));
#273538=CARTESIAN_POINT('Ctrl Pts',(10.1651884842034,-69.361128093948,17.4049408966644));
#273539=CARTESIAN_POINT('Origin',(0.884028484203416,-17.542318193471,0.972561099047131));
#273540=CARTESIAN_POINT('',(10.1651884842034,-64.4275078998505,28.4860332810842));
#273541=CARTESIAN_POINT('',(11.5201159294503,-59.6960744004839,27.7254875603419));
#273542=CARTESIAN_POINT('Ctrl Pts',(10.1651884842034,-64.4275078998505,
28.4860332810842));
#273543=CARTESIAN_POINT('Ctrl Pts',(10.189490010882,-64.379637209956,28.4828842736812));
#273544=CARTESIAN_POINT('Ctrl Pts',(10.2135007848618,-64.3316279326639,
28.4795910574541));
#273545=CARTESIAN_POINT('Ctrl Pts',(10.8759790020178,-62.9869067906345,
28.3835177865881));
#273546=CARTESIAN_POINT('Ctrl Pts',(11.3015145825508,-61.5978417176892,
28.1819261126647));
#273547=CARTESIAN_POINT('Ctrl Pts',(11.4908939831593,-60.0303486615357,
27.8101373762517));
#273548=CARTESIAN_POINT('Ctrl Pts',(11.5073957447759,-59.8630126866082,
27.7686607366359));
#273549=CARTESIAN_POINT('Ctrl Pts',(11.5201159294506,-59.6960744004839,
27.7254875603419));
#273550=CARTESIAN_POINT('',(10.1651884842034,-64.8122789026216,27.8195903550054));
#273551=CARTESIAN_POINT('Origin',(10.1651884842034,-17.542318193471,0.972561099047131));
#273552=CARTESIAN_POINT('',(11.5201159294506,-61.7879102380359,24.1023216086084));
#273553=CARTESIAN_POINT('Ctrl Pts',(11.5201159294506,-61.7879102380359,
24.1023216086084));
#273554=CARTESIAN_POINT('Ctrl Pts',(11.5064953958128,-61.9173229284605,
24.2340129191289));
#273555=CARTESIAN_POINT('Ctrl Pts',(11.4885385348232,-62.0452839747836,
24.3670769367845));
#273556=CARTESIAN_POINT('Ctrl Pts',(11.2877548088084,-63.1857922323705,
25.5789913071247));
#273557=CARTESIAN_POINT('Ctrl Pts',(10.8383054247334,-64.0737673949273,
26.7148967508734));
#273558=CARTESIAN_POINT('Ctrl Pts',(10.1651884842034,-64.8122789026216,
27.8195903550054));
#273559=CARTESIAN_POINT('Ctrl Pts',(11.5520284842034,-61.2401701856317,
23.3668214500608));
#273560=CARTESIAN_POINT('Ctrl Pts',(11.5520284842034,-61.2999060970714,
23.475250045364));
#273561=CARTESIAN_POINT('Ctrl Pts',(11.5505454879221,-61.3656142043454,
23.5803821574562));
#273562=CARTESIAN_POINT('Ctrl Pts',(11.5472514053777,-61.4370558175126,
23.6817591254573));
#273563=CARTESIAN_POINT('Ctrl Pts',(11.5440439814882,-61.5066179895845,
23.7804691318469));
#273564=CARTESIAN_POINT('Ctrl Pts',(11.5391190647213,-61.5816160066261,
23.8756186960842));
#273565=CARTESIAN_POINT('Ctrl Pts',(11.5322062136934,-61.6618177977578,
23.9667491847357));
#273566=CARTESIAN_POINT('Ctrl Pts',(11.5286980345291,-61.702519130892,24.0129966852584));
#273567=CARTESIAN_POINT('Ctrl Pts',(11.5246784421826,-61.7445604645659,
24.0582085586416));
#273568=CARTESIAN_POINT('Ctrl Pts',(11.5201159294506,-61.7879102380359,
24.1023216086084));
#273569=CARTESIAN_POINT('Ctrl Pts',(11.5201159294506,-59.6960744004839,
27.7254875603419));
#273570=CARTESIAN_POINT('Ctrl Pts',(11.5379482942249,-59.4620444324384,
27.6649632953391));
#273571=CARTESIAN_POINT('Ctrl Pts',(11.5475950755165,-59.2212150991993,
27.6295440253416));
#273572=CARTESIAN_POINT('Ctrl Pts',(11.5516325551658,-58.9133324392308,
27.6181375894728));
#273573=CARTESIAN_POINT('Ctrl Pts',(11.5520284842034,-58.8492360373286,
27.6175978245548));
#273574=CARTESIAN_POINT('Ctrl Pts',(11.5520284842034,-58.7852425524921,
27.6188808395635));
#273575=CARTESIAN_POINT('Origin',(0.884028484203416,-17.542318193471,0.972561099047131));
#273576=CARTESIAN_POINT('',(11.5201159294503,-56.0120902791562,32.7960567002403));
#273577=CARTESIAN_POINT('Ctrl Pts',(11.5520284842034,-55.6292387426316,
31.9627474243937));
#273578=CARTESIAN_POINT('Ctrl Pts',(11.5520284842034,-55.6651257148405,
32.0812264100182));
#273579=CARTESIAN_POINT('Ctrl Pts',(11.5505454874064,-55.7075397574413,
32.1977226423425));
#273580=CARTESIAN_POINT('Ctrl Pts',(11.5472514032083,-55.7563427586746,
32.3117378556073));
#273581=CARTESIAN_POINT('Ctrl Pts',(11.5440439778628,-55.8038618789157,
32.422753622907));
#273582=CARTESIAN_POINT('Ctrl Pts',(11.5391190587251,-55.8574383198082,
32.5314169312553));
#273583=CARTESIAN_POINT('Ctrl Pts',(11.5322062038027,-55.916940438255,32.6372309180193));
#273584=CARTESIAN_POINT('Ctrl Pts',(11.5286980270414,-55.9471369274812,
32.6909300298275));
#273585=CARTESIAN_POINT('Ctrl Pts',(11.5246784379819,-55.9788594516457,
32.7438947495814));
#273586=CARTESIAN_POINT('Ctrl Pts',(11.5201159294506,-56.0120902791562,
32.7960567002404));
#273587=CARTESIAN_POINT('',(11.5201159294502,-53.2126675143875,35.9051306570903));
#273588=CARTESIAN_POINT('Ctrl Pts',(11.5201159294506,-53.2126675143875,
35.9051306570903));
#273589=CARTESIAN_POINT('Ctrl Pts',(11.5379482942249,-52.9963353649162,
35.7972714261332));
#273590=CARTESIAN_POINT('Ctrl Pts',(11.5475950755165,-52.7681328107348,
35.7125549182932));
#273591=CARTESIAN_POINT('Ctrl Pts',(11.5516325551658,-52.4693496569467,
35.6373853360076));
#273592=CARTESIAN_POINT('Ctrl Pts',(11.5520284842034,-52.4067661386471,
35.6235309749533));
#273593=CARTESIAN_POINT('Ctrl Pts',(11.5520284842034,-52.3439043111719,
35.6114809593721));
#273594=CARTESIAN_POINT('',(10.1651884842034,-57.6825814930807,37.6327769679278));
#273595=CARTESIAN_POINT('Ctrl Pts',(10.1651884842034,-57.6825814930807,
37.6327769679277));
#273596=CARTESIAN_POINT('Ctrl Pts',(10.189490010882,-57.6364116080685,37.6197438978153));
#273597=CARTESIAN_POINT('Ctrl Pts',(10.2135007848618,-57.5901361468263,
37.6065409562473));
#273598=CARTESIAN_POINT('Ctrl Pts',(10.8759790020178,-56.2947751442824,
37.2329838705373));
#273599=CARTESIAN_POINT('Ctrl Pts',(11.3015145825508,-54.9779777416979,
36.7469945903893));
#273600=CARTESIAN_POINT('Ctrl Pts',(11.4908939831593,-53.5220373944691,
36.057430198237));
#273601=CARTESIAN_POINT('Ctrl Pts',(11.5073957447759,-53.3669815903493,
35.9820688172286));
#273602=CARTESIAN_POINT('Ctrl Pts',(11.5201159294506,-53.2126675143875,
35.9051306570903));
#273603=CARTESIAN_POINT('',(10.1651884842034,-58.1975056018677,37.0608958085216));
#273604=CARTESIAN_POINT('Origin',(10.1651884842034,-17.542318193471,0.972561099047131));
#273605=CARTESIAN_POINT('Ctrl Pts',(11.5201159294506,-56.0120902791562,
32.7960567002404));
#273606=CARTESIAN_POINT('Ctrl Pts',(11.5064953958128,-56.1112948287632,
32.9517766509429));
#273607=CARTESIAN_POINT('Ctrl Pts',(11.4885385348232,-56.2087940543137,
33.1085374980566));
#273608=CARTESIAN_POINT('Ctrl Pts',(11.2877548088084,-57.0724083042256,
34.5310936319262));
#273609=CARTESIAN_POINT('Ctrl Pts',(10.8383054247334,-57.7048110575729,
35.8267972338408));
#273610=CARTESIAN_POINT('Ctrl Pts',(10.1651884842034,-58.1975056018678,
37.0608958085216));
#273611=CARTESIAN_POINT('Origin',(0.884028484203416,-17.542318193471,0.972561099047131));
#273612=CARTESIAN_POINT('',(10.1651884842034,-49.1833329657644,45.177293306068));
#273613=CARTESIAN_POINT('',(11.5201159294506,-45.1702951976404,42.5580528390857));
#273614=CARTESIAN_POINT('Ctrl Pts',(10.1651884842034,-49.1833329657644,
45.177293306068));
#273615=CARTESIAN_POINT('Ctrl Pts',(10.189490010882,-49.1408817311572,45.1549457809496));
#273616=CARTESIAN_POINT('Ctrl Pts',(10.2135007848618,-49.0983625456755,
45.1324101459419));
#273617=CARTESIAN_POINT('Ctrl Pts',(10.8759790020178,-47.9089751742599,
44.4976954825594));
#273618=CARTESIAN_POINT('Ctrl Pts',(11.3015145825508,-46.7219958072243,
43.7485486597644));
#273619=CARTESIAN_POINT('Ctrl Pts',(11.4908939831593,-45.441239748471,42.7713458847071));
#273620=CARTESIAN_POINT('Ctrl Pts',(11.5073957447759,-45.3052407978392,
42.6653934162801));
#273621=CARTESIAN_POINT('Ctrl Pts',(11.5201159294506,-45.1702951976404,
42.5580528390857));
#273622=CARTESIAN_POINT('',(10.1651884842034,-49.8059055261334,44.7249678641907));
#273623=CARTESIAN_POINT('Origin',(10.1651884842034,-17.542318193471,0.972561099047131));
#273624=CARTESIAN_POINT('',(11.5201159294504,-48.5549566816847,40.0989523280257));
#273625=CARTESIAN_POINT('Ctrl Pts',(11.5201159294506,-48.5549566816847,
40.0989523280258));
#273626=CARTESIAN_POINT('Ctrl Pts',(11.5064953958128,-48.61961737562,40.2718952098375));
#273627=CARTESIAN_POINT('Ctrl Pts',(11.4885385348232,-48.6823935963883,
40.4455016851683));
#273628=CARTESIAN_POINT('Ctrl Pts',(11.2877548088084,-49.2313697518231,
42.0165270533355));
#273629=CARTESIAN_POINT('Ctrl Pts',(10.8383054247334,-49.5805610610345,
43.4154003485366));
#273630=CARTESIAN_POINT('Ctrl Pts',(10.1651884842034,-49.8059055261334,
44.7249678641907));
#273631=CARTESIAN_POINT('Ctrl Pts',(11.5520284842034,-48.3537261103113,
39.2042535488961));
#273632=CARTESIAN_POINT('Ctrl Pts',(11.5520284842034,-48.3641956404978,
39.3276041062429));
#273633=CARTESIAN_POINT('Ctrl Pts',(11.550545504126,-48.3814617755172,39.4503723241464));
#273634=CARTESIAN_POINT('Ctrl Pts',(11.5472514575585,-48.405493015199,39.5720421023164));
#273635=CARTESIAN_POINT('Ctrl Pts',(11.5440440708938,-48.4288920401097,
39.690510987317));
#273636=CARTESIAN_POINT('Ctrl Pts',(11.5391192124522,-48.4587050452548,
39.8079382320109));
#273637=CARTESIAN_POINT('Ctrl Pts',(11.5322064453586,-48.4949065665672,
39.9238104557194));
#273638=CARTESIAN_POINT('Ctrl Pts',(11.5286982114168,-48.5132788629418,
39.9826156870571));
#273639=CARTESIAN_POINT('Ctrl Pts',(11.5246785424948,-48.5332966106893,
40.0410198365814));
#273640=CARTESIAN_POINT('Ctrl Pts',(11.5201159294506,-48.5549566816847,
40.0989523280258));
#273641=CARTESIAN_POINT('Ctrl Pts',(11.5201159294506,-45.1702951976404,
42.5580528390857));
#273642=CARTESIAN_POINT('Ctrl Pts',(11.5379482942249,-44.9811156197522,
42.4075726081333));
#273643=CARTESIAN_POINT('Ctrl Pts',(11.5475950755165,-44.7755133912835,
42.2772613803582));
#273644=CARTESIAN_POINT('Ctrl Pts',(11.5516325551658,-44.4988880012169,
42.1416139231055));
#273645=CARTESIAN_POINT('Ctrl Pts',(11.5520284842034,-44.4405525665788,
42.1150504679734));
#273646=CARTESIAN_POINT('Ctrl Pts',(11.5520284842034,-44.38156975997,42.0901940653056));
#273647=CARTESIAN_POINT('Origin',(0.884028484203416,-17.542318193471,0.972561099047131));
#273648=CARTESIAN_POINT('',(11.5201159294504,-39.742421967128,45.6918369098492));
#273649=CARTESIAN_POINT('Ctrl Pts',(11.5520284842034,-39.7316071024862,
44.7748512573256));
#273650=CARTESIAN_POINT('Ctrl Pts',(11.5520284842034,-39.7162020260023,
44.897681447115));
#273651=CARTESIAN_POINT('Ctrl Pts',(11.5505455425311,-39.7075659332829,
45.0213551478053));
#273652=CARTESIAN_POINT('Ctrl Pts',(11.5472515828821,-39.7057753139112,
45.1453609704374));
#273653=CARTESIAN_POINT('Ctrl Pts',(11.5440442853249,-39.7040318046552,
45.2661042746653));
#273654=CARTESIAN_POINT('Ctrl Pts',(11.5391195667906,-39.7087784989904,
45.3871622545795));
#273655=CARTESIAN_POINT('Ctrl Pts',(11.5322070025992,-39.7200972254515,
45.5080274415157));
#273656=CARTESIAN_POINT('Ctrl Pts',(11.5286986366911,-39.7258418714236,
45.5693707129246));
#273657=CARTESIAN_POINT('Ctrl Pts',(11.5246787835194,-39.7332795799714,
45.630663768993));
#273658=CARTESIAN_POINT('Ctrl Pts',(11.5201159294506,-39.742421967128,45.6918369098492));
#273659=CARTESIAN_POINT('',(11.5201159294506,-35.9204477120687,47.3934894827124));
#273660=CARTESIAN_POINT('Ctrl Pts',(11.5201159294506,-35.9204477120687,
47.3934894827124));
#273661=CARTESIAN_POINT('Ctrl Pts',(11.5379482942249,-35.7666887611015,
47.2069649599417));
#273662=CARTESIAN_POINT('Ctrl Pts',(11.5475950755165,-35.5926726623188,
47.0367542381881));
#273663=CARTESIAN_POINT('Ctrl Pts',(11.5516325551658,-35.3502948929158,
46.8465573507588));
#273664=CARTESIAN_POINT('Ctrl Pts',(11.5520284842034,-35.298757080357,46.8084457520039));
#273665=CARTESIAN_POINT('Ctrl Pts',(11.5520284842034,-35.2462311262942,
46.7718693063201));
#273666=CARTESIAN_POINT('',(10.1651884842034,-39.3012202624647,50.7898507289222));
#273667=CARTESIAN_POINT('Ctrl Pts',(10.1651884842034,-39.3012202624647,
50.7898507289222));
#273668=CARTESIAN_POINT('Ctrl Pts',(10.189490010882,-39.2643430009184,50.7591654428808));
#273669=CARTESIAN_POINT('Ctrl Pts',(10.2135007848618,-39.2274383836324,
50.7282820298214));
#273670=CARTESIAN_POINT('Ctrl Pts',(10.8759790020178,-38.1960065787899,
49.8601498652548));
#273671=CARTESIAN_POINT('Ctrl Pts',(11.3015145825508,-37.1907219414015,
48.8805868107745));
#273672=CARTESIAN_POINT('Ctrl Pts',(11.4908939831593,-36.1411253566406,
47.6584541032212));
#273673=CARTESIAN_POINT('Ctrl Pts',(11.5073957447759,-36.0301270662348,
47.5265411786622));
#273674=CARTESIAN_POINT('Ctrl Pts',(11.5201159294506,-35.9204477120687,
47.3934894827124));
#273675=CARTESIAN_POINT('',(10.1651884842034,-40.004231866093,50.4768497968822));
#273676=CARTESIAN_POINT('Origin',(10.1651884842034,-17.542318193471,0.972561099047131));
#273677=CARTESIAN_POINT('Ctrl Pts',(11.5201159294506,-39.742421967128,45.6918369098492));
#273678=CARTESIAN_POINT('Ctrl Pts',(11.5064953958128,-39.7697128227903,
45.8744442889629));
#273679=CARTESIAN_POINT('Ctrl Pts',(11.4885385348232,-39.7950224166949,
46.0573089564827));
#273680=CARTESIAN_POINT('Ctrl Pts',(11.2877548088084,-40.0053675853803,
47.7081422117425));
#273681=CARTESIAN_POINT('Ctrl Pts',(10.8383054247334,-40.0560861146374,
49.1490477246911));
#273682=CARTESIAN_POINT('Ctrl Pts',(10.1651884842034,-40.004231866093,50.4768497968821));
#273683=CARTESIAN_POINT('Origin',(0.884028484203416,-17.542318193471,0.972561099047131));
#273684=CARTESIAN_POINT('',(10.1651884842034,-17.9270891962415,-53.3879403389487));
#273685=CARTESIAN_POINT('Ctrl Pts',(10.1651884842034,-17.9270891962415,
-53.3879403389487));
#273686=CARTESIAN_POINT('Ctrl Pts',(10.189490010882,-17.9482974207811,-53.3449086017019));
#273687=CARTESIAN_POINT('Ctrl Pts',(10.2135007848618,-17.9694500505142,
-53.3016847398361));
#273688=CARTESIAN_POINT('Ctrl Pts',(10.8759790020178,-18.5586087283343,
-52.0890854343996));
#273689=CARTESIAN_POINT('Ctrl Pts',(11.3015145825508,-19.0785577539979,
-50.7853239567576));
#273690=CARTESIAN_POINT('Ctrl Pts',(11.4908939831593,-19.5403257915001,
-49.2419407816664));
#273691=CARTESIAN_POINT('Ctrl Pts',(11.5073957447759,-19.588073955393,-49.0762852566043));
#273692=CARTESIAN_POINT('Ctrl Pts',(11.5201159294506,-19.6341540310225,
-48.9101258718094));
#273693=CARTESIAN_POINT('',(10.1651884842034,-17.1575471906993,-53.3879403389487));
#273694=CARTESIAN_POINT('Origin',(10.1651884842034,-17.542318193471,0.972561099047131));
#273695=CARTESIAN_POINT('Ctrl Pts',(11.5201159294506,-15.4504823559185,
-48.9101258718094));
#273696=CARTESIAN_POINT('Ctrl Pts',(11.5064953958128,-15.4998240310746,
-49.0880462045494));
#273697=CARTESIAN_POINT('Ctrl Pts',(11.4885385348232,-15.5510803275324,
-49.2653957301879));
#273698=CARTESIAN_POINT('Ctrl Pts',(11.2877548088084,-16.030374830665,-50.8590620396541));
#273699=CARTESIAN_POINT('Ctrl Pts',(10.8383054247334,-16.57011021997,-52.1960238102323));
#273700=CARTESIAN_POINT('Ctrl Pts',(10.1651884842034,-17.1575471906993,
-53.3879403389487));
#273701=CARTESIAN_POINT('Origin',(0.884028484203416,-17.542318193471,0.972561099047131));
#273702=CARTESIAN_POINT('',(10.1651884842034,-29.2208647943379,-52.1200345674514));
#273703=CARTESIAN_POINT('Ctrl Pts',(10.1651884842034,-29.2208647943379,
-52.1200345674514));
#273704=CARTESIAN_POINT('Ctrl Pts',(10.189490010882,-29.2326627670373,-52.0735337390848));
#273705=CARTESIAN_POINT('Ctrl Pts',(10.2135007848618,-29.2443664148558,
-52.0268565432932));
#273706=CARTESIAN_POINT('Ctrl Pts',(10.8759790020178,-29.5685369901393,
-50.7182624651635));
#273707=CARTESIAN_POINT('Ctrl Pts',(11.3015145825508,-29.8060566288565,
-49.334887822814));
#273708=CARTESIAN_POINT('Ctrl Pts',(11.4908939831593,-29.9368465213218,
-47.729224299643));
#273709=CARTESIAN_POINT('Ctrl Pts',(11.5073957447759,-29.9491095529641,
-47.5572613437668));
#273710=CARTESIAN_POINT('Ctrl Pts',(11.5201159294507,-29.9596361897448,
-47.3851523537531));
#273711=CARTESIAN_POINT('',(10.1651884842034,-28.4681391279529,-52.280031346979));
#273712=CARTESIAN_POINT('Origin',(10.1651884842034,-17.542318193471,0.972561099047131));
#273713=CARTESIAN_POINT('Ctrl Pts',(11.5201159294506,-25.8673877784838,
-48.2549866055504));
#273714=CARTESIAN_POINT('Ctrl Pts',(11.5064953958128,-25.9526429368648,
-48.4187602410323));
#273715=CARTESIAN_POINT('Ctrl Pts',(11.4885385348232,-26.0396522000087,
-48.5815774707652));
#273716=CARTESIAN_POINT('Ctrl Pts',(11.2877548088084,-26.8398148252932,
-50.040767417194));
#273717=CARTESIAN_POINT('Ctrl Pts',(10.8383054247334,-27.6457256836526,
-51.2362960679732));
#273718=CARTESIAN_POINT('Ctrl Pts',(10.1651884842034,-28.4681391279529,
-52.2800313469789));
#273719=CARTESIAN_POINT('Origin',(0.884028484203416,-17.542318193471,0.972561099047131));
#273720=CARTESIAN_POINT('',(10.1651884842034,-40.0042318660923,-48.5317275987882));
#273721=CARTESIAN_POINT('Ctrl Pts',(10.1651884842034,-40.0042318660923,
-48.5317275987882));
#273722=CARTESIAN_POINT('Ctrl Pts',(10.189490010882,-40.0061039589316,-48.4837899886371));
#273723=CARTESIAN_POINT('Ctrl Pts',(10.2135007848618,-40.0078471192654,
-48.4356994763579));
#273724=CARTESIAN_POINT('Ctrl Pts',(10.8759790020178,-40.0528617823294,
-47.0883024660804));
#273725=CARTESIAN_POINT('Ctrl Pts',(11.3015145825508,-39.9975712861425,
-45.6857747690621));
#273726=CARTESIAN_POINT('Ctrl Pts',(11.4908939831593,-39.7916668876708,
-44.0880060986022));
#273727=CARTESIAN_POINT('Ctrl Pts',(11.5073957447759,-39.7679088337352,
-43.9172513182535));
#273728=CARTESIAN_POINT('Ctrl Pts',(11.5201159294506,-39.7424219671274,
-43.7467147117552));
#273729=CARTESIAN_POINT('',(10.1651884842034,-39.301220262464,-48.8447285308283));
#273730=CARTESIAN_POINT('Origin',(10.1651884842034,-17.542318193471,0.972561099047131));
#273731=CARTESIAN_POINT('Ctrl Pts',(11.5201159294506,-35.9204477120681,
-45.4483672846184));
#273732=CARTESIAN_POINT('Ctrl Pts',(11.5064953958128,-36.037890294153,-45.5908365290986));
#273733=CARTESIAN_POINT('Ctrl Pts',(11.4885385348232,-36.1568498016669,
-45.7320055687029));
#273734=CARTESIAN_POINT('Ctrl Pts',(11.2877548088084,-37.242909602772,-46.9929455494649));
#273735=CARTESIAN_POINT('Ctrl Pts',(10.8383054247334,-38.2797737584862,
-47.9947907416233));
#273736=CARTESIAN_POINT('Ctrl Pts',(10.1651884842034,-39.301220262464,-48.8447285308282));
#273737=CARTESIAN_POINT('Origin',(0.884028484203416,-17.542318193471,0.972561099047131));
#273738=CARTESIAN_POINT('',(10.1651884842034,-49.8059055261328,-42.7798456660969));
#273739=CARTESIAN_POINT('Ctrl Pts',(10.1651884842034,-49.8059055261328,
-42.7798456660969));
#273740=CARTESIAN_POINT('Ctrl Pts',(10.189490010882,-49.7977699196717,-42.7325663777551));
#273741=CARTESIAN_POINT('Ctrl Pts',(10.2135007848618,-49.7894764080497,
-42.6851643351388));
#273742=CARTESIAN_POINT('Ctrl Pts',(10.8759790020178,-49.5533678021139,
-41.3578521075907));
#273743=CARTESIAN_POINT('Ctrl Pts',(11.3015145825508,-49.2076836310195,
-39.9974685463379));
#273744=CARTESIAN_POINT('Ctrl Pts',(11.4908939831593,-48.674083951863,-38.477424886433));
#273745=CARTESIAN_POINT('Ctrl Pts',(11.5073957447759,-48.6153431533102,
-38.3153410848854));
#273746=CARTESIAN_POINT('Ctrl Pts',(11.5201159294506,-48.5549566816842,
-38.1538301299319));
#273747=CARTESIAN_POINT('',(10.1651884842034,-49.1833329657638,-43.2321711079742));
#273748=CARTESIAN_POINT('Origin',(10.1651884842034,-17.542318193471,0.972561099047131));
#273749=CARTESIAN_POINT('Ctrl Pts',(11.5201159294506,-45.1702951976399,
-40.6129306409918));
#273750=CARTESIAN_POINT('Ctrl Pts',(11.5064953958128,-45.3147923990396,
-40.7278689048432));
#273751=CARTESIAN_POINT('Ctrl Pts',(11.4885385348232,-45.4605030496141,
-40.841219989884));
#273752=CARTESIAN_POINT('Ctrl Pts',(11.2877548088084,-46.7849940017385,
-41.8488008771588));
#273753=CARTESIAN_POINT('Ctrl Pts',(10.8383054247334,-48.0074955157765,
-42.6131771684123));
#273754=CARTESIAN_POINT('Ctrl Pts',(10.1651884842034,-49.1833329657638,
-43.2321711079742));
#273755=CARTESIAN_POINT('Origin',(0.884028484203416,-17.542318193471,0.972561099047131));
#273756=CARTESIAN_POINT('',(10.1651884842034,-58.1975056018673,-35.1157736104279));
#273757=CARTESIAN_POINT('Ctrl Pts',(10.1651884842034,-58.1975056018673,
-35.1157736104278));
#273758=CARTESIAN_POINT('Ctrl Pts',(10.189490010882,-58.179717861147,-35.0712189756671));
#273759=CARTESIAN_POINT('Ctrl Pts',(10.2135007848618,-58.1617501438237,
-35.0265770994362));
#273760=CARTESIAN_POINT('Ctrl Pts',(10.8759790020178,-57.6548373479424,
-33.7773595681121));
#273761=CARTESIAN_POINT('Ctrl Pts',(11.3015145825508,-57.033867558994,-32.5185754320962));
#273762=CARTESIAN_POINT('Ctrl Pts',(11.4908939831593,-56.1958934656271,
-31.1426899846628));
#273763=CARTESIAN_POINT('Ctrl Pts',(11.5073957447759,-56.1047371772236,
-30.9963610018083));
#273764=CARTESIAN_POINT('Ctrl Pts',(11.5201159294506,-56.0120902791558,
-30.8509345021466));
#273765=CARTESIAN_POINT('',(10.1651884842034,-57.6825814930802,-35.687654769834));
#273766=CARTESIAN_POINT('Origin',(10.1651884842034,-17.542318193471,0.972561099047131));
#273767=CARTESIAN_POINT('Ctrl Pts',(11.5201159294506,-53.212667514387,-33.9600084589965));
#273768=CARTESIAN_POINT('Ctrl Pts',(11.5064953958128,-53.3779041140259,
-34.0423923885538));
#273769=CARTESIAN_POINT('Ctrl Pts',(11.4885385348232,-53.5439976530335,
-34.1229715326959));
#273770=CARTESIAN_POINT('Ctrl Pts',(11.2877548088084,-55.0490331459566,
-34.8331572068));
#273771=CARTESIAN_POINT('Ctrl Pts',(10.8383054247334,-56.4037428359418,
-35.3266576853365));
#273772=CARTESIAN_POINT('Ctrl Pts',(10.1651884842034,-57.6825814930802,
-35.687654769834));
#273773=CARTESIAN_POINT('Origin',(0.884028484203416,-17.542318193471,0.972561099047131));
#273774=CARTESIAN_POINT('',(10.1651884842034,-64.8122789026212,-25.8744681569117));
#273775=CARTESIAN_POINT('Ctrl Pts',(10.1651884842034,-64.8122789026212,
-25.8744681569117));
#273776=CARTESIAN_POINT('Ctrl Pts',(10.189490010882,-64.7856164372663,-25.8345854270679));
#273777=CARTESIAN_POINT('Ctrl Pts',(10.2135007848618,-64.7587597897074,
-25.7946547814292));
#273778=CARTESIAN_POINT('Ctrl Pts',(10.8759790020178,-64.0031973254981,
-24.6781287468588));
#273779=CARTESIAN_POINT('Ctrl Pts',(11.3015145825508,-63.1340812782164,
-23.5759589431401));
#273780=CARTESIAN_POINT('Ctrl Pts',(11.4908939831593,-62.028356259565,-22.4043645044619));
#273781=CARTESIAN_POINT('Ctrl Pts',(11.5073957447759,-61.9087684485304,
-22.2801856190156));
#273782=CARTESIAN_POINT('Ctrl Pts',(11.5201159294506,-61.7879102380356,
-22.1571994105147));
#273783=CARTESIAN_POINT('',(10.1651884842034,-64.4275078998501,-26.5409110829905));
#273784=CARTESIAN_POINT('Origin',(10.1651884842034,-17.542318193471,0.972561099047131));
#273785=CARTESIAN_POINT('Ctrl Pts',(11.5201159294506,-59.6960744004836,
-25.7803653622482));
#273786=CARTESIAN_POINT('Ctrl Pts',(11.5064953958128,-59.8748287660643,
-25.8265943844678));
#273787=CARTESIAN_POINT('Ctrl Pts',(11.4885385348232,-60.0540461088452,
-25.8708798924506));
#273788=CARTESIAN_POINT('Ctrl Pts',(11.2877548088084,-61.6738488695646,
-26.2526318315767));
#273789=CARTESIAN_POINT('Ctrl Pts',(10.8383054247334,-63.1015594214264,
-26.4536881584061));
#273790=CARTESIAN_POINT('Ctrl Pts',(10.1651884842034,-64.4275078998501,
-26.5409110829905));
#273791=CARTESIAN_POINT('Origin',(0.884028484203416,-17.542318193471,0.972561099047131));
#273792=CARTESIAN_POINT('',(11.5201159294506,-65.6299855106615,-12.4525827957101));
#273793=CARTESIAN_POINT('Ctrl Pts',(11.5201159294506,-65.6299855106615,
-12.4525827957101));
#273794=CARTESIAN_POINT('Ctrl Pts',(11.5379482942249,-65.4284106018844,
-12.3191632740911));
#273795=CARTESIAN_POINT('Ctrl Pts',(11.5475950755165,-65.2409426768843,
-12.1638923188816));
#273796=CARTESIAN_POINT('Ctrl Pts',(11.5516325551658,-65.0264523321392,
-11.9427233086211));
#273797=CARTESIAN_POINT('Ctrl Pts',(11.5520284842034,-64.9831623443631,
-11.8954515724427));
#273798=CARTESIAN_POINT('Ctrl Pts',(11.5520284842034,-64.9412958110162,
-11.8470366407114));
#273799=CARTESIAN_POINT('',(10.1651884842034,-69.3611280939478,-15.4598186985709));
#273800=CARTESIAN_POINT('Ctrl Pts',(10.1651884842034,-69.3611280939478,
-15.4598186985709));
#273801=CARTESIAN_POINT('Ctrl Pts',(10.189490010882,-69.3267561816351,-15.4263509403167));
#273802=CARTESIAN_POINT('Ctrl Pts',(10.2135007848618,-69.2921843682114,
-15.3928766860931));
#273803=CARTESIAN_POINT('Ctrl Pts',(10.8759790020178,-68.3209939409509,
-14.4578396936734));
#273804=CARTESIAN_POINT('Ctrl Pts',(11.3015145825508,-67.2417161770836,
-13.5604543314719));
#273805=CARTESIAN_POINT('Ctrl Pts',(11.4908939831593,-65.9165657223201,
-12.6443552004531));
#273806=CARTESIAN_POINT('Ctrl Pts',(11.5073957447759,-65.7737729498426,
-12.5477536255854));
#273807=CARTESIAN_POINT('Ctrl Pts',(11.5201159294506,-65.6299855106615,
-12.4525827957101));
#273808=CARTESIAN_POINT('',(10.1651884842034,-69.1233265363499,-16.1916966375046));
#273809=CARTESIAN_POINT('Origin',(10.1651884842034,-17.542318193471,0.972561099047131));
#273810=CARTESIAN_POINT('Ctrl Pts',(11.5201159294507,-64.3371598641692,
-16.4314910043572));
#273811=CARTESIAN_POINT('Ctrl Pts',(11.5064953958128,-64.5216195721572,
-16.4395446891366));
#273812=CARTESIAN_POINT('Ctrl Pts',(11.4885385348232,-64.7061280608517,
-16.4456010717559));
#273813=CARTESIAN_POINT('Ctrl Pts',(11.2877548088084,-66.369904936048,-16.4822348843151));
#273814=CARTESIAN_POINT('Ctrl Pts',(10.8383054247334,-67.8082185477548,
-16.3820599331797));
#273815=CARTESIAN_POINT('Ctrl Pts',(10.1651884842034,-69.1233265363499,
-16.1916966375046));
#273816=CARTESIAN_POINT('Origin',(0.884028484203416,-17.542318193471,0.972561099047131));
#273817=CARTESIAN_POINT('',(10.1651884842034,29.3428715129087,-26.5409110829896));
#273818=CARTESIAN_POINT('Ctrl Pts',(10.1651884842034,29.3428715129087,-26.5409110829896));
#273819=CARTESIAN_POINT('Ctrl Pts',(10.189490010882,29.2950008230142,-26.5377620755867));
#273820=CARTESIAN_POINT('Ctrl Pts',(10.2135007848618,29.2469915457221,-26.5344688593595));
#273821=CARTESIAN_POINT('Ctrl Pts',(10.8759790020178,27.9022704036928,-26.4383955884935));
#273822=CARTESIAN_POINT('Ctrl Pts',(11.3015145825508,26.5132053307474,-26.2368039145702));
#273823=CARTESIAN_POINT('Ctrl Pts',(11.4908939831593,24.9457122745938,-25.8650151781571));
#273824=CARTESIAN_POINT('Ctrl Pts',(11.5073957447759,24.7783762996664,-25.8235385385413));
#273825=CARTESIAN_POINT('Ctrl Pts',(11.5201159294506,24.6114380135421,-25.7803653622474));
#273826=CARTESIAN_POINT('',(10.1651884842034,29.7276425156798,-25.8744681569108));
#273827=CARTESIAN_POINT('Origin',(10.1651884842034,-17.542318193471,0.972561099047131));
#273828=CARTESIAN_POINT('Ctrl Pts',(11.5201159294506,26.7032738510941,-22.1571994105139));
#273829=CARTESIAN_POINT('Ctrl Pts',(11.5064953958128,26.8326865415187,-22.2888907210343));
#273830=CARTESIAN_POINT('Ctrl Pts',(11.4885385348232,26.9606475878418,-22.4219547386899));
#273831=CARTESIAN_POINT('Ctrl Pts',(11.2877548088084,28.1011558454287,-23.6338691090301));
#273832=CARTESIAN_POINT('Ctrl Pts',(10.8383054247334,28.9891310079854,-24.7697745527788));
#273833=CARTESIAN_POINT('Ctrl Pts',(10.1651884842034,29.7276425156798,-25.8744681569108));
#273834=CARTESIAN_POINT('Origin',(0.884028484203416,-17.542318193471,0.972561099047131));
#273835=CARTESIAN_POINT('',(10.1651884842034,22.597945106139,-35.6876547698332));
#273836=CARTESIAN_POINT('Ctrl Pts',(10.1651884842034,22.5979451061389,-35.6876547698332));
#273837=CARTESIAN_POINT('Ctrl Pts',(10.189490010882,22.5517752211267,-35.6746216997208));
#273838=CARTESIAN_POINT('Ctrl Pts',(10.2135007848618,22.5054997598846,-35.6614187581527));
#273839=CARTESIAN_POINT('Ctrl Pts',(10.8759790020178,21.2101387573406,-35.2878616724428));
#273840=CARTESIAN_POINT('Ctrl Pts',(11.3015145825508,19.8933413547562,-34.8018723922948));
#273841=CARTESIAN_POINT('Ctrl Pts',(11.4908939831593,18.4374010075274,-34.1123080001425));
#273842=CARTESIAN_POINT('Ctrl Pts',(11.5073957447759,18.2823452034076,-34.0369466191341));
#273843=CARTESIAN_POINT('Ctrl Pts',(11.5201159294506,18.1280311274458,-33.9600084589958));
#273844=CARTESIAN_POINT('',(10.1651884842034,23.112869214926,-35.115773610427));
#273845=CARTESIAN_POINT('Origin',(10.1651884842034,-17.542318193471,0.972561099047131));
#273846=CARTESIAN_POINT('Ctrl Pts',(11.5201159294506,20.9274538922145,-30.8509345021458));
#273847=CARTESIAN_POINT('Ctrl Pts',(11.5064953958128,21.0266584418215,-31.0066544528484));
#273848=CARTESIAN_POINT('Ctrl Pts',(11.4885385348232,21.124157667372,-31.163415299962));
#273849=CARTESIAN_POINT('Ctrl Pts',(11.2877548088084,21.9877719172839,-32.5859714338316));
#273850=CARTESIAN_POINT('Ctrl Pts',(10.8383054247334,22.6201746706312,-33.8816750357462));
#273851=CARTESIAN_POINT('Ctrl Pts',(10.1651884842034,23.112869214926,-35.115773610427));
#273852=CARTESIAN_POINT('Origin',(0.884028484203416,-17.542318193471,0.972561099047131));
#273853=CARTESIAN_POINT('',(10.1651884842034,14.0986965788227,-43.2321711079735));
#273854=CARTESIAN_POINT('Ctrl Pts',(10.1651884842034,14.0986965788227,-43.2321711079735));
#273855=CARTESIAN_POINT('Ctrl Pts',(10.189490010882,14.0562453442155,-43.2098235828551));
#273856=CARTESIAN_POINT('Ctrl Pts',(10.2135007848618,14.0137261587338,-43.1872879478475));
#273857=CARTESIAN_POINT('Ctrl Pts',(10.8759790020178,12.8243387873183,-42.5525732844649));
#273858=CARTESIAN_POINT('Ctrl Pts',(11.3015145825508,11.6373594202826,-41.80342646167));
#273859=CARTESIAN_POINT('Ctrl Pts',(11.4908939831593,10.3566033615292,-40.8262236866127));
#273860=CARTESIAN_POINT('Ctrl Pts',(11.5073957447759,10.2206044108975,-40.7202712181856));
#273861=CARTESIAN_POINT('Ctrl Pts',(11.5201159294506,10.0856588106987,-40.6129306409912));
#273862=CARTESIAN_POINT('',(10.1651884842034,14.7212691391918,-42.7798456660962));
#273863=CARTESIAN_POINT('Origin',(10.1651884842034,-17.542318193471,0.972561099047131));
#273864=CARTESIAN_POINT('Ctrl Pts',(11.5201159294506,13.470320294743,-38.1538301299313));
#273865=CARTESIAN_POINT('Ctrl Pts',(11.5064953958128,13.5349809886783,-38.326773011743));
#273866=CARTESIAN_POINT('Ctrl Pts',(11.4885385348232,13.5977572094466,-38.5003794870738));
#273867=CARTESIAN_POINT('Ctrl Pts',(11.2877548088084,14.1467333648814,-40.071404855241));
#273868=CARTESIAN_POINT('Ctrl Pts',(10.8383054247334,14.4959246740928,-41.4702781504422));
#273869=CARTESIAN_POINT('Ctrl Pts',(10.1651884842034,14.7212691391918,-42.7798456660963));
#273870=CARTESIAN_POINT('Origin',(0.884028484203416,-17.542318193471,0.972561099047131));
#273871=CARTESIAN_POINT('',(10.1651884842034,34.0386901494083,-16.1916966375036));
#273872=CARTESIAN_POINT('Ctrl Pts',(10.1651884842034,34.0386901494082,-16.1916966375036));
#273873=CARTESIAN_POINT('Ctrl Pts',(10.189490010882,33.991210833489,-16.1985693195443));
#273874=CARTESIAN_POINT('Ctrl Pts',(10.2135007848618,33.9435659759387,-16.2053297580097));
#273875=CARTESIAN_POINT('Ctrl Pts',(10.8759790020178,32.6082554610186,-16.3909391649352));
#273876=CARTESIAN_POINT('Ctrl Pts',(11.3015145825508,31.2076315268737,-16.4825556207311));
#273877=CARTESIAN_POINT('Ctrl Pts',(11.4908939831593,29.5970927300156,-16.4447914918788));
#273878=CARTESIAN_POINT('Ctrl Pts',(11.5073957447759,29.4247899693519,-16.439012321834));
#273879=CARTESIAN_POINT('Ctrl Pts',(11.5201159294506,29.2525234772276,-16.4314910043563));
#273880=CARTESIAN_POINT('',(10.1651884842034,34.2764917070062,-15.4598186985698));
#273881=CARTESIAN_POINT('Origin',(10.1651884842034,-17.542318193471,0.972561099047131));
#273882=CARTESIAN_POINT('',(11.5201159294503,30.5453491237198,-12.4525827957091));
#273883=CARTESIAN_POINT('Ctrl Pts',(11.5201159294506,30.5453491237198,-12.4525827957091));
#273884=CARTESIAN_POINT('Ctrl Pts',(11.5064953958128,30.6993139993994,-12.5544899238528));
#273885=CARTESIAN_POINT('Ctrl Pts',(11.4885385348232,30.8521443547455,-12.6580415759667));
#273886=CARTESIAN_POINT('Ctrl Pts',(11.2877548088084,32.219700936385,-13.6063477093833));
#273887=CARTESIAN_POINT('Ctrl Pts',(10.8383054247334,33.32443973257,-14.5328104763952));
#273888=CARTESIAN_POINT('Ctrl Pts',(10.1651884842034,34.2764917070062,-15.4598186985698));
#273889=CARTESIAN_POINT('Ctrl Pts',(11.5520284842034,29.8566594240744,-11.8470366407104));
#273890=CARTESIAN_POINT('Ctrl Pts',(11.5520284842034,29.9376329966379,-11.9406753940128));
#273891=CARTESIAN_POINT('Ctrl Pts',(11.5505455075224,30.0237628247143,-12.0298480784021));
#273892=CARTESIAN_POINT('Ctrl Pts',(11.5472514703205,30.1147200651852,-12.1141556807327));
#273893=CARTESIAN_POINT('Ctrl Pts',(11.544044092433,30.2032844085471,-12.196245324198));
#273894=CARTESIAN_POINT('Ctrl Pts',(11.539119248065,30.2964254868395,-12.2737222219197));
#273895=CARTESIAN_POINT('Ctrl Pts',(11.5322065029565,30.3938209389875,-12.3461860127879));
#273896=CARTESIAN_POINT('Ctrl Pts',(11.5286982551648,30.4432495486874,-12.3829616974549));
#273897=CARTESIAN_POINT('Ctrl Pts',(11.5246785671409,30.4937736154884,-12.4184457114994));
#273898=CARTESIAN_POINT('Ctrl Pts',(11.5201159294506,30.5453491237198,-12.4525827957091));
#273899=CARTESIAN_POINT('Origin',(0.884028484203416,-17.542318193471,0.972561099047131));
#273900=CARTESIAN_POINT('',(10.1651884842034,36.4801712081848,-5.09232176568361));
#273901=CARTESIAN_POINT('',(11.520115929451,31.8484498133401,-6.32197605563879));
#273902=CARTESIAN_POINT('Ctrl Pts',(10.1651884842034,36.4801712081848,-5.09232176568361));
#273903=CARTESIAN_POINT('Ctrl Pts',(10.189490010882,36.4351583401774,-5.10891576798397));
#273904=CARTESIAN_POINT('Ctrl Pts',(10.2135007848618,36.3899602112694,-5.12543439754089));
#273905=CARTESIAN_POINT('Ctrl Pts',(10.8759790020178,35.1224198004912,-5.58461446052246));
#273906=CARTESIAN_POINT('Ctrl Pts',(11.3015145825508,33.7714509920083,-5.96543496729491));
#273907=CARTESIAN_POINT('Ctrl Pts',(11.4908939831593,32.1882547280909,-6.26334591964661));
#273908=CARTESIAN_POINT('Ctrl Pts',(11.5073957447759,32.0185156391323,-6.29351679663514));
#273909=CARTESIAN_POINT('Ctrl Pts',(11.5201159294506,31.8484498133401,-6.3219760556388));
#273910=CARTESIAN_POINT('',(10.1651884842034,36.560610251444,-4.32699539176697));
#273911=CARTESIAN_POINT('Origin',(10.1651884842034,-17.542318193471,0.972561099047131));
#273912=CARTESIAN_POINT('',(11.5201159294509,32.2857625843551,-2.16122297171639));
#273913=CARTESIAN_POINT('Ctrl Pts',(11.5201159294506,32.285762584355,-2.16122297171638));
#273914=CARTESIAN_POINT('Ctrl Pts',(11.5064953958128,32.4575506414171,-2.22889208697866));
#273915=CARTESIAN_POINT('Ctrl Pts',(11.4885385348232,32.6285708858962,-2.29840566945766));
#273916=CARTESIAN_POINT('Ctrl Pts',(11.2877548088084,34.1634070067061,-2.94165803744265));
#273917=CARTESIAN_POINT('Ctrl Pts',(10.8383054247334,35.4366270500011,-3.6181872591378));
#273918=CARTESIAN_POINT('Ctrl Pts',(10.1651884842034,36.560610251444,-4.32699539176698));
#273919=CARTESIAN_POINT('Ctrl Pts',(11.5520284842034,31.4862222820429,-1.71209609297288));
#273920=CARTESIAN_POINT('Ctrl Pts',(11.5520284842034,31.5848954455677,-1.78685361573));
#273921=CARTESIAN_POINT('Ctrl Pts',(11.5505454936052,31.6876836794972,-1.85617057017899));
#273922=CARTESIAN_POINT('Ctrl Pts',(11.547251423208,31.7941823732418,-1.91972502887827));
#273923=CARTESIAN_POINT('Ctrl Pts',(11.5440440121231,31.8978793346475,-1.98160751794148));
#273924=CARTESIAN_POINT('Ctrl Pts',(11.5391191153364,32.0050940195483,-2.03802645190818));
#273925=CARTESIAN_POINT('Ctrl Pts',(11.5322062926149,32.1154278761199,-2.08865723676024));
#273926=CARTESIAN_POINT('Ctrl Pts',(11.528698094849,32.1714213544321,-2.11435192234124));
#273927=CARTESIAN_POINT('Ctrl Pts',(11.5246784764318,32.2282177698874,-2.13855546648027));
#273928=CARTESIAN_POINT('Ctrl Pts',(11.5201159294506,32.285762584355,-2.16122297171638));
#273929=CARTESIAN_POINT('Ctrl Pts',(11.5201159294506,31.8484498133401,-6.32197605563879));
#273930=CARTESIAN_POINT('Ctrl Pts',(11.5379482942249,31.610035362708,-6.36187295185028));
#273931=CARTESIAN_POINT('Ctrl Pts',(11.5475950755165,31.3756205042814,-6.42746995318688));
#273932=CARTESIAN_POINT('Ctrl Pts',(11.5516325551658,31.0897162833456,-6.54227681508785));
#273933=CARTESIAN_POINT('Ctrl Pts',(11.5520284842034,31.0309417643657,-6.56785407064173));
#273934=CARTESIAN_POINT('Ctrl Pts',(11.5520284842034,30.9730026561922,-6.59505465837618));
#273935=CARTESIAN_POINT('Origin',(0.884028484203416,-17.542318193471,0.972561099047131));
#273936=CARTESIAN_POINT('',(10.1651884842034,4.21658387552303,-48.8447285308278));
#273937=CARTESIAN_POINT('Ctrl Pts',(10.1651884842034,4.21658387552304,-48.8447285308278));
#273938=CARTESIAN_POINT('Ctrl Pts',(10.189490010882,4.17970661397677,-48.8140432447864));
#273939=CARTESIAN_POINT('Ctrl Pts',(10.2135007848618,4.14280199669075,-48.783159831727));
#273940=CARTESIAN_POINT('Ctrl Pts',(10.8759790020178,3.11137019184823,-47.9150276671604));
#273941=CARTESIAN_POINT('Ctrl Pts',(11.3015145825508,2.10608555445984,-46.9354646126801));
#273942=CARTESIAN_POINT('Ctrl Pts',(11.4908939831593,1.05648896969897,-45.7133319051268));
#273943=CARTESIAN_POINT('Ctrl Pts',(11.5073957447759,0.945490679293149,
-45.5814189805678));
#273944=CARTESIAN_POINT('Ctrl Pts',(11.5201159294506,0.835811325126995,
-45.448367284618));
#273945=CARTESIAN_POINT('',(10.1651884842034,4.91959547915134,-48.5317275987877));
#273946=CARTESIAN_POINT('Origin',(10.1651884842034,-17.542318193471,0.972561099047131));
#273947=CARTESIAN_POINT('Ctrl Pts',(11.5201159294506,4.65778558018633,-43.7467147117548));
#273948=CARTESIAN_POINT('Ctrl Pts',(11.5064953958128,4.68507643584861,-43.9293220908684));
#273949=CARTESIAN_POINT('Ctrl Pts',(11.4885385348232,4.71038602975324,-44.1121867583883));
#273950=CARTESIAN_POINT('Ctrl Pts',(11.2877548088084,4.9207311984387,-45.763020013648));
#273951=CARTESIAN_POINT('Ctrl Pts',(10.8383054247334,4.97144972769578,-47.2039255265966));
#273952=CARTESIAN_POINT('Ctrl Pts',(10.1651884842034,4.91959547915134,-48.5317275987877));
#273953=CARTESIAN_POINT('Origin',(0.884028484203416,-17.542318193471,0.972561099047131));
#273954=CARTESIAN_POINT('',(10.1651884842034,-6.616497258988,-52.2800313469788));
#273955=CARTESIAN_POINT('Ctrl Pts',(10.1651884842034,-6.61649725898799,
-52.2800313469787));
#273956=CARTESIAN_POINT('Ctrl Pts',(10.189490010882,-6.646188834187,-52.2423493942587));
#273957=CARTESIAN_POINT('Ctrl Pts',(10.2135007848618,-6.67586597441391,
-52.2044679564932));
#273958=CARTESIAN_POINT('Ctrl Pts',(10.8759790020178,-7.50426369345284,
-51.1408598320946));
#273959=CARTESIAN_POINT('Ctrl Pts',(11.3015145825508,-8.28391783864927,
-49.9736921518746));
#273960=CARTESIAN_POINT('Ctrl Pts',(11.4908939831593,-9.05648254214045,
-48.5600425755889));
#273961=CARTESIAN_POINT('Ctrl Pts',(11.5073957447759,-9.13762901440063,
-48.4079344226896));
#273962=CARTESIAN_POINT('Ctrl Pts',(11.5201159294506,-9.21724860845719,
-48.2549866055502));
#273963=CARTESIAN_POINT('',(10.1651884842034,-5.863771592603,-52.1200345674512));
#273964=CARTESIAN_POINT('Origin',(10.1651884842034,-17.542318193471,0.972561099047131));
#273965=CARTESIAN_POINT('Ctrl Pts',(11.5201159294506,-5.12500019719618,
-47.3851523537529));
#273966=CARTESIAN_POINT('Ctrl Pts',(11.5064953958128,-5.13627192115547,
-47.5694434114538));
#273967=CARTESIAN_POINT('Ctrl Pts',(11.4885385348232,-5.14953510481703,
-47.75357420771));
#273968=CARTESIAN_POINT('Ctrl Pts',(11.2877548088084,-5.28701401610064,
-49.4120660152306));
#273969=CARTESIAN_POINT('Ctrl Pts',(10.8383054247334,-5.53698490990081,
-50.832029260779));
#273970=CARTESIAN_POINT('Ctrl Pts',(10.1651884842034,-5.863771592603,-52.1200345674512));
#273971=CARTESIAN_POINT('Origin',(0.561048484203417,-17.542318193471,0.972561099047131));
#273972=CARTESIAN_POINT('',(6.14788848420341,-28.4681391279537,54.2251535450731));
#273973=CARTESIAN_POINT('',(8.15653848420341,-28.4681391279536,54.2251535450731));
#273974=CARTESIAN_POINT('',(6.14788848420341,-29.2208647943386,54.0651567655455));
#273975=CARTESIAN_POINT('Origin',(6.14788848420341,-17.542318193471,0.972561099047131));
#273976=CARTESIAN_POINT('',(8.15653848420342,-29.2208647943386,54.0651567655455));
#273977=CARTESIAN_POINT('Origin',(0.561048484203417,-17.542318193471,0.972561099047131));
#273978=CARTESIAN_POINT('',(6.14788848420341,-6.6164972589887,54.2251535450731));
#273979=CARTESIAN_POINT('',(8.15653848420342,-6.6164972589887,54.2251535450731));
#273980=CARTESIAN_POINT('',(6.14788848420341,-5.86377159260369,54.0651567655456));
#273981=CARTESIAN_POINT('',(8.15653848420342,-5.86377159260369,54.0651567655456));
#273982=CARTESIAN_POINT('Origin',(6.14788848420341,-17.542318193471,0.972561099047131));
#273983=CARTESIAN_POINT('Origin',(0.561048484203417,-17.542318193471,0.972561099047131));
#273984=CARTESIAN_POINT('',(6.14788848420341,4.21658387552239,50.7898507289224));
#273985=CARTESIAN_POINT('',(8.15653848420342,4.21658387552238,50.7898507289224));
#273986=CARTESIAN_POINT('',(6.14788848420341,4.91959547915065,50.4768497968823));
#273987=CARTESIAN_POINT('',(8.15653848420342,4.91959547915064,50.4768497968823));
#273988=CARTESIAN_POINT('Origin',(6.14788848420341,-17.542318193471,0.972561099047131));
#273989=CARTESIAN_POINT('Origin',(0.561048484203417,-17.542318193471,0.972561099047131));
#273990=CARTESIAN_POINT('',(6.14788848420341,14.0986965788221,45.1772933060682));
#273991=CARTESIAN_POINT('',(8.15653848420342,14.0986965788221,45.1772933060682));
#273992=CARTESIAN_POINT('',(6.14788848420341,14.7212691391912,44.7249678641909));
#273993=CARTESIAN_POINT('',(8.15653848420341,14.7212691391912,44.7249678641909));
#273994=CARTESIAN_POINT('Origin',(6.14788848420341,-17.542318193471,0.972561099047131));
#273995=CARTESIAN_POINT('Origin',(0.561048484203417,-17.542318193471,0.972561099047131));
#273996=CARTESIAN_POINT('',(6.14788848420341,29.7276425156794,27.8195903550057));
#273997=CARTESIAN_POINT('',(8.15653848420341,29.7276425156794,27.8195903550057));
#273998=CARTESIAN_POINT('',(6.14788848420342,29.3428715129083,28.4860332810845));
#273999=CARTESIAN_POINT('Origin',(6.14788848420341,-17.542318193471,0.972561099047131));
#274000=CARTESIAN_POINT('',(8.15653848420341,29.3428715129083,28.4860332810845));
#274001=CARTESIAN_POINT('Origin',(0.561048484203417,-17.542318193471,0.972561099047131));
#274002=CARTESIAN_POINT('',(6.14788848420342,34.2764917070059,17.4049408966648));
#274003=CARTESIAN_POINT('',(8.15653848420342,34.2764917070059,17.4049408966648));
#274004=CARTESIAN_POINT('Origin',(6.14788848420341,-17.542318193471,0.972561099047131));
#274005=CARTESIAN_POINT('Origin',(0.561048484203417,-17.542318193471,0.972561099047131));
#274006=CARTESIAN_POINT('',(6.14788848420341,22.5979451061385,37.632776967928));
#274007=CARTESIAN_POINT('',(8.15653848420341,22.5979451061385,37.632776967928));
#274008=CARTESIAN_POINT('',(6.14788848420341,23.1128692149255,37.0608958085218));
#274009=CARTESIAN_POINT('',(8.15653848420341,23.1128692149255,37.0608958085218));
#274010=CARTESIAN_POINT('Origin',(6.14788848420341,-17.542318193471,0.972561099047131));
#274011=CARTESIAN_POINT('Origin',(0.561048484203417,-17.542318193471,0.972561099047131));
#274012=CARTESIAN_POINT('',(6.14788848420342,-71.6452466383859,-4.32699539176735));
#274013=CARTESIAN_POINT('',(8.15653848420341,-71.6452466383859,-4.32699539176735));
#274014=CARTESIAN_POINT('',(6.14788848420341,-71.5648075951267,-5.0923217656847));
#274015=CARTESIAN_POINT('Origin',(6.14788848420341,-17.542318193471,0.972561099047131));
#274016=CARTESIAN_POINT('',(8.15653848420342,-71.5648075951267,-5.0923217656847));
#274017=CARTESIAN_POINT('Origin',(0.561048484203417,-17.542318193471,0.972561099047131));
#274018=CARTESIAN_POINT('',(6.14788848420341,-71.645246638386,6.27211758986086));
#274019=CARTESIAN_POINT('',(8.15653848420342,-71.645246638386,6.27211758986086));
#274020=CARTESIAN_POINT('',(6.14788848420341,-71.5648075951268,7.03744396377822));
#274021=CARTESIAN_POINT('',(8.15653848420341,-71.5648075951268,7.03744396377822));
#274022=CARTESIAN_POINT('Origin',(6.14788848420341,-17.542318193471,0.972561099047131));
#274023=CARTESIAN_POINT('Origin',(0.561048484203417,-17.542318193471,0.972561099047131));
#274024=CARTESIAN_POINT('',(6.14788848420341,-69.361128093948,17.4049408966644));
#274025=CARTESIAN_POINT('',(8.15653848420342,-69.361128093948,17.4049408966644));
#274026=CARTESIAN_POINT('Origin',(6.14788848420341,-17.542318193471,0.972561099047131));
#274027=CARTESIAN_POINT('Origin',(0.561048484203417,-17.542318193471,0.972561099047131));
#274028=CARTESIAN_POINT('',(6.14788848420341,-64.4275078998505,28.4860332810842));
#274029=CARTESIAN_POINT('',(8.15653848420341,-64.4275078998505,28.4860332810842));
#274030=CARTESIAN_POINT('',(6.14788848420341,-64.8122789026216,27.8195903550054));
#274031=CARTESIAN_POINT('Origin',(6.14788848420341,-17.542318193471,0.972561099047131));
#274032=CARTESIAN_POINT('',(8.15653848420342,-64.8122789026216,27.8195903550054));
#274033=CARTESIAN_POINT('Origin',(0.561048484203417,-17.542318193471,0.972561099047131));
#274034=CARTESIAN_POINT('',(6.14788848420341,-58.1975056018677,37.0608958085216));
#274035=CARTESIAN_POINT('',(8.15653848420341,-58.1975056018677,37.0608958085215));
#274036=CARTESIAN_POINT('',(6.14788848420342,-57.6825814930807,37.6327769679278));
#274037=CARTESIAN_POINT('',(8.15653848420341,-57.6825814930807,37.6327769679278));
#274038=CARTESIAN_POINT('Origin',(6.14788848420341,-17.542318193471,0.972561099047131));
#274039=CARTESIAN_POINT('Origin',(0.561048484203417,-17.542318193471,0.972561099047131));
#274040=CARTESIAN_POINT('',(6.14788848420341,-49.1833329657644,45.177293306068));
#274041=CARTESIAN_POINT('',(8.15653848420341,-49.1833329657644,45.177293306068));
#274042=CARTESIAN_POINT('',(6.14788848420341,-49.8059055261334,44.7249678641907));
#274043=CARTESIAN_POINT('Origin',(6.14788848420341,-17.542318193471,0.972561099047131));
#274044=CARTESIAN_POINT('',(8.15653848420341,-49.8059055261334,44.7249678641907));
#274045=CARTESIAN_POINT('Origin',(0.561048484203417,-17.542318193471,0.972561099047131));
#274046=CARTESIAN_POINT('',(6.14788848420341,-40.004231866093,50.4768497968821));
#274047=CARTESIAN_POINT('',(8.15653848420341,-40.004231866093,50.4768497968821));
#274048=CARTESIAN_POINT('',(6.14788848420341,-39.3012202624647,50.7898507289222));
#274049=CARTESIAN_POINT('',(8.15653848420341,-39.3012202624647,50.7898507289222));
#274050=CARTESIAN_POINT('Origin',(6.14788848420341,-17.542318193471,0.972561099047131));
#274051=CARTESIAN_POINT('Origin',(0.561048484203417,-17.542318193471,0.972561099047131));
#274052=CARTESIAN_POINT('',(6.14788848420341,-17.9270891962415,-53.3879403389487));
#274053=CARTESIAN_POINT('',(8.15653848420342,-17.9270891962415,-53.3879403389487));
#274054=CARTESIAN_POINT('',(6.14788848420341,-17.1575471906993,-53.3879403389487));
#274055=CARTESIAN_POINT('Origin',(6.14788848420341,-17.542318193471,0.972561099047131));
#274056=CARTESIAN_POINT('',(8.15653848420341,-17.1575471906993,-53.3879403389487));
#274057=CARTESIAN_POINT('Origin',(0.561048484203417,-17.542318193471,0.972561099047131));
#274058=CARTESIAN_POINT('',(6.14788848420341,-28.4681391279529,-52.280031346979));
#274059=CARTESIAN_POINT('',(8.15653848420342,-28.4681391279529,-52.280031346979));
#274060=CARTESIAN_POINT('',(6.14788848420341,-29.2208647943379,-52.1200345674514));
#274061=CARTESIAN_POINT('',(8.15653848420342,-29.2208647943379,-52.1200345674514));
#274062=CARTESIAN_POINT('Origin',(6.14788848420341,-17.542318193471,0.972561099047131));
#274063=CARTESIAN_POINT('Origin',(0.561048484203417,-17.542318193471,0.972561099047131));
#274064=CARTESIAN_POINT('',(6.14788848420341,-39.301220262464,-48.8447285308283));
#274065=CARTESIAN_POINT('',(8.15653848420342,-39.301220262464,-48.8447285308283));
#274066=CARTESIAN_POINT('',(6.14788848420342,-40.0042318660923,-48.5317275987882));
#274067=CARTESIAN_POINT('',(8.15653848420342,-40.0042318660923,-48.5317275987882));
#274068=CARTESIAN_POINT('Origin',(6.14788848420341,-17.542318193471,0.972561099047131));
#274069=CARTESIAN_POINT('Origin',(0.561048484203417,-17.542318193471,0.972561099047131));
#274070=CARTESIAN_POINT('',(6.14788848420342,-49.8059055261329,-42.7798456660969));
#274071=CARTESIAN_POINT('',(8.15653848420341,-49.8059055261328,-42.7798456660969));
#274072=CARTESIAN_POINT('',(6.14788848420341,-49.1833329657638,-43.2321711079742));
#274073=CARTESIAN_POINT('Origin',(6.14788848420341,-17.542318193471,0.972561099047131));
#274074=CARTESIAN_POINT('',(8.15653848420342,-49.1833329657638,-43.2321711079742));
#274075=CARTESIAN_POINT('Origin',(0.561048484203417,-17.542318193471,0.972561099047131));
#274076=CARTESIAN_POINT('',(6.14788848420341,-57.6825814930802,-35.687654769834));
#274077=CARTESIAN_POINT('',(8.15653848420341,-57.6825814930802,-35.687654769834));
#274078=CARTESIAN_POINT('',(6.14788848420341,-58.1975056018673,-35.1157736104278));
#274079=CARTESIAN_POINT('',(8.15653848420341,-58.1975056018673,-35.1157736104278));
#274080=CARTESIAN_POINT('Origin',(6.14788848420341,-17.542318193471,0.972561099047131));
#274081=CARTESIAN_POINT('Origin',(0.561048484203417,-17.542318193471,0.972561099047131));
#274082=CARTESIAN_POINT('',(6.14788848420341,-64.8122789026212,-25.8744681569117));
#274083=CARTESIAN_POINT('',(8.15653848420341,-64.8122789026212,-25.8744681569117));
#274084=CARTESIAN_POINT('',(6.14788848420341,-64.4275078998501,-26.5409110829905));
#274085=CARTESIAN_POINT('Origin',(6.14788848420341,-17.542318193471,0.972561099047131));
#274086=CARTESIAN_POINT('',(8.15653848420341,-64.4275078998501,-26.5409110829905));
#274087=CARTESIAN_POINT('Origin',(0.561048484203417,-17.542318193471,0.972561099047131));
#274088=CARTESIAN_POINT('',(6.14788848420341,-69.1233265363499,-16.1916966375046));
#274089=CARTESIAN_POINT('',(8.15653848420341,-69.1233265363499,-16.1916966375046));
#274090=CARTESIAN_POINT('',(6.14788848420341,-69.3611280939478,-15.4598186985709));
#274091=CARTESIAN_POINT('',(8.15653848420342,-69.3611280939478,-15.4598186985708));
#274092=CARTESIAN_POINT('Origin',(6.14788848420341,-17.542318193471,0.972561099047131));
#274093=CARTESIAN_POINT('Origin',(0.561048484203417,-17.542318193471,0.972561099047131));
#274094=CARTESIAN_POINT('',(6.14788848420342,29.3428715129087,-26.5409110829896));
#274095=CARTESIAN_POINT('',(8.15653848420341,29.3428715129087,-26.5409110829896));
#274096=CARTESIAN_POINT('',(6.14788848420341,29.7276425156798,-25.8744681569108));
#274097=CARTESIAN_POINT('Origin',(6.14788848420341,-17.542318193471,0.972561099047131));
#274098=CARTESIAN_POINT('',(8.15653848420341,29.7276425156798,-25.8744681569108));
#274099=CARTESIAN_POINT('Origin',(0.561048484203417,-17.542318193471,0.972561099047131));
#274100=CARTESIAN_POINT('',(6.14788848420341,23.112869214926,-35.115773610427));
#274101=CARTESIAN_POINT('',(8.15653848420341,23.112869214926,-35.115773610427));
#274102=CARTESIAN_POINT('',(6.14788848420341,22.597945106139,-35.6876547698332));
#274103=CARTESIAN_POINT('',(8.15653848420341,22.5979451061389,-35.6876547698332));
#274104=CARTESIAN_POINT('Origin',(6.14788848420341,-17.542318193471,0.972561099047131));
#274105=CARTESIAN_POINT('Origin',(0.561048484203417,-17.542318193471,0.972561099047131));
#274106=CARTESIAN_POINT('',(6.14788848420341,14.7212691391918,-42.7798456660962));
#274107=CARTESIAN_POINT('',(8.15653848420341,14.7212691391918,-42.7798456660962));
#274108=CARTESIAN_POINT('',(6.14788848420341,14.0986965788227,-43.2321711079735));
#274109=CARTESIAN_POINT('',(8.15653848420341,14.0986965788227,-43.2321711079735));
#274110=CARTESIAN_POINT('Origin',(6.14788848420341,-17.542318193471,0.972561099047131));
#274111=CARTESIAN_POINT('Origin',(0.561048484203417,-17.542318193471,0.972561099047131));
#274112=CARTESIAN_POINT('',(6.14788848420341,34.0386901494082,-16.1916966375036));
#274113=CARTESIAN_POINT('',(8.15653848420342,34.0386901494082,-16.1916966375036));
#274114=CARTESIAN_POINT('',(6.14788848420341,34.2764917070062,-15.4598186985698));
#274115=CARTESIAN_POINT('Origin',(6.14788848420341,-17.542318193471,0.972561099047131));
#274116=CARTESIAN_POINT('',(8.15653848420341,34.2764917070062,-15.4598186985698));
#274117=CARTESIAN_POINT('Origin',(0.561048484203417,-17.542318193471,0.972561099047131));
#274118=CARTESIAN_POINT('',(6.14788848420341,36.4801712081848,-5.09232176568361));
#274119=CARTESIAN_POINT('',(8.15653848420342,36.4801712081848,-5.09232176568361));
#274120=CARTESIAN_POINT('',(6.14788848420341,36.560610251444,-4.32699539176698));
#274121=CARTESIAN_POINT('Origin',(6.14788848420341,-17.542318193471,0.972561099047131));
#274122=CARTESIAN_POINT('',(8.15653848420341,36.560610251444,-4.32699539176697));
#274123=CARTESIAN_POINT('Origin',(0.561048484203417,-17.542318193471,0.972561099047131));
#274124=CARTESIAN_POINT('',(6.14788848420341,4.91959547915134,-48.5317275987877));
#274125=CARTESIAN_POINT('',(8.15653848420341,4.91959547915134,-48.5317275987877));
#274126=CARTESIAN_POINT('',(6.14788848420342,4.21658387552304,-48.8447285308278));
#274127=CARTESIAN_POINT('',(8.15653848420342,4.21658387552303,-48.8447285308278));
#274128=CARTESIAN_POINT('Origin',(6.14788848420341,-17.542318193471,0.972561099047131));
#274129=CARTESIAN_POINT('Origin',(0.561048484203417,-17.542318193471,0.972561099047131));
#274130=CARTESIAN_POINT('',(6.14788848420341,-5.863771592603,-52.1200345674512));
#274131=CARTESIAN_POINT('',(8.15653848420341,-5.863771592603,-52.1200345674512));
#274132=CARTESIAN_POINT('',(6.14788848420341,-6.61649725898799,-52.2800313469788));
#274133=CARTESIAN_POINT('',(8.15653848420342,-6.61649725898799,-52.2800313469788));
#274134=CARTESIAN_POINT('Origin',(6.14788848420341,-17.542318193471,0.972561099047131));
#274135=CARTESIAN_POINT('Origin',(15.4290484842034,-17.542318193471,0.972561099047131));
#274136=CARTESIAN_POINT('',(4.79296103895619,-25.8673877784845,50.2001088036445));
#274137=CARTESIAN_POINT('Ctrl Pts',(4.79296103895619,-25.8673877784845,
50.2001088036445));
#274138=CARTESIAN_POINT('Ctrl Pts',(4.80658157259404,-25.9526429368654,
50.3638824391265));
#274139=CARTESIAN_POINT('Ctrl Pts',(4.8245384335836,-26.0396522000094,50.5266996688594));
#274140=CARTESIAN_POINT('Ctrl Pts',(5.0253221595984,-26.8398148252939,51.9858896152881));
#274141=CARTESIAN_POINT('Ctrl Pts',(5.47477154367345,-27.6457256836533,
53.1814182660674));
#274142=CARTESIAN_POINT('Ctrl Pts',(6.14788848420342,-28.4681391279537,
54.2251535450731));
#274143=CARTESIAN_POINT('',(4.76104848420342,-25.3371465446544,49.451895009213));
#274144=CARTESIAN_POINT('Ctrl Pts',(4.76104848420342,-25.3371465446544,
49.451895009213));
#274145=CARTESIAN_POINT('Ctrl Pts',(4.76104848420342,-25.4218077136479,
49.5422122981067));
#274146=CARTESIAN_POINT('Ctrl Pts',(4.76253144074934,-25.5014883801629,
49.6371907160477));
#274147=CARTESIAN_POINT('Ctrl Pts',(4.76582543152198,-25.575826089086,49.7364615046949));
#274148=CARTESIAN_POINT('Ctrl Pts',(4.76903276223312,-25.6482080820183,
49.8331206246266));
#274149=CARTESIAN_POINT('Ctrl Pts',(4.77395753237976,-25.7155242765978,
49.9338491853259));
#274150=CARTESIAN_POINT('Ctrl Pts',(4.78087016904194,-25.777410200811,50.0382847362108));
#274151=CARTESIAN_POINT('Ctrl Pts',(4.78437848713686,-25.8088186948993,
50.091288119844));
#274152=CARTESIAN_POINT('Ctrl Pts',(4.78839827319647,-25.8388280077851,
50.1452459945807));
#274153=CARTESIAN_POINT('Ctrl Pts',(4.79296103895619,-25.8673877784845,
50.2001088036445));
#274154=CARTESIAN_POINT('',(4.76104848420342,-30.1397096933157,48.4310786991304));
#274155=CARTESIAN_POINT('Origin',(4.76104848420342,-17.542318193471,0.972561099047131));
#274156=CARTESIAN_POINT('',(4.79296103895619,-29.9596361897455,49.3302745518473));
#274157=CARTESIAN_POINT('Ctrl Pts',(4.79296103895619,-29.9596361897455,
49.3302745518473));
#274158=CARTESIAN_POINT('Ctrl Pts',(4.77035892158036,-29.9783406571863,
49.0244592124324));
#274159=CARTESIAN_POINT('Ctrl Pts',(4.76104848420342,-30.0387016815049,
48.7219745577429));
#274160=CARTESIAN_POINT('Ctrl Pts',(4.76104848420342,-30.1397096933157,
48.4310786991304));
#274161=CARTESIAN_POINT('Ctrl Pts',(6.14788848420341,-29.2208647943386,
54.0651567655455));
#274162=CARTESIAN_POINT('Ctrl Pts',(6.12358695752486,-29.2326627670381,
54.0186559371789));
#274163=CARTESIAN_POINT('Ctrl Pts',(6.099576183545,-29.2443664148566,53.9719787413873));
#274164=CARTESIAN_POINT('Ctrl Pts',(5.437097966389,-29.56853699014,52.6633846632577));
#274165=CARTESIAN_POINT('Ctrl Pts',(5.01156238585602,-29.8060566288571,
51.2800100209081));
#274166=CARTESIAN_POINT('Ctrl Pts',(4.82218298524757,-29.9368465213225,
49.6743464977371));
#274167=CARTESIAN_POINT('Ctrl Pts',(4.80568122363092,-29.9491095529648,
49.5023835418609));
#274168=CARTESIAN_POINT('Ctrl Pts',(4.79296103895619,-29.9596361897455,
49.3302745518473));
#274169=CARTESIAN_POINT('Origin',(15.4290484842034,-17.542318193471,0.972561099047131));
#274170=CARTESIAN_POINT('',(4.79296103895619,-9.21724860845784,50.2001088036446));
#274171=CARTESIAN_POINT('',(4.76104848420342,-9.74748984228791,49.4518950092131));
#274172=CARTESIAN_POINT('Ctrl Pts',(4.79296103895619,-9.21724860845785,
50.2001088036446));
#274173=CARTESIAN_POINT('Ctrl Pts',(4.77035892158039,-9.35872229428056,
49.9283403817424));
#274174=CARTESIAN_POINT('Ctrl Pts',(4.76104848420342,-9.53689642689581,
49.6765579398481));
#274175=CARTESIAN_POINT('Ctrl Pts',(4.76104848420342,-9.74748984228792,
49.4518950092131));
#274176=CARTESIAN_POINT('Ctrl Pts',(6.14788848420341,-6.61649725898869,
54.2251535450731));
#274177=CARTESIAN_POINT('Ctrl Pts',(6.12358695752485,-6.64618883418769,
54.1874715923531));
#274178=CARTESIAN_POINT('Ctrl Pts',(6.099576183545,-6.6758659744146,54.1495901545876));
#274179=CARTESIAN_POINT('Ctrl Pts',(5.43709796638901,-7.50426369345351,
53.085982030189));
#274180=CARTESIAN_POINT('Ctrl Pts',(5.01156238585602,-8.28391783864993,
51.918814349969));
#274181=CARTESIAN_POINT('Ctrl Pts',(4.82218298524757,-9.05648254214109,
50.5051647736833));
#274182=CARTESIAN_POINT('Ctrl Pts',(4.80568122363092,-9.13762901440128,
50.3530566207839));
#274183=CARTESIAN_POINT('Ctrl Pts',(4.79296103895619,-9.21724860845783,
50.2001088036446));
#274184=CARTESIAN_POINT('',(4.79296103895619,-5.12500019719682,49.3302745518473));
#274185=CARTESIAN_POINT('Ctrl Pts',(4.79296103895619,-5.12500019719682,
49.3302745518473));
#274186=CARTESIAN_POINT('Ctrl Pts',(4.80658157259404,-5.13627192115611,
49.5145656095482));
#274187=CARTESIAN_POINT('Ctrl Pts',(4.8245384335836,-5.14953510481761,49.6986964058044));
#274188=CARTESIAN_POINT('Ctrl Pts',(5.02532215959839,-5.28701401610125,
51.357188213325));
#274189=CARTESIAN_POINT('Ctrl Pts',(5.47477154367344,-5.53698490990151,
52.7771514588735));
#274190=CARTESIAN_POINT('Ctrl Pts',(6.14788848420341,-5.86377159260369,
54.0651567655456));
#274191=CARTESIAN_POINT('',(4.76104848420342,-4.94492669362663,48.4310786991305));
#274192=CARTESIAN_POINT('Ctrl Pts',(4.76104848420342,-4.94492669362663,
48.4310786991305));
#274193=CARTESIAN_POINT('Ctrl Pts',(4.76104848420342,-4.98553194226763,
48.5480189146228));
#274194=CARTESIAN_POINT('Ctrl Pts',(4.76253135162946,-5.01969184244055,
48.6671915454769));
#274195=CARTESIAN_POINT('Ctrl Pts',(4.76582514301953,-5.0472252496888,48.7881122473915));
#274196=CARTESIAN_POINT('Ctrl Pts',(4.76903226819321,-5.07403419811496,
48.9058512846292));
#274197=CARTESIAN_POINT('Ctrl Pts',(4.773956716031,-5.09456054852597,49.0252474567679));
#274198=CARTESIAN_POINT('Ctrl Pts',(4.7808688874334,-5.1086187509111,49.1458213738986));
#274199=CARTESIAN_POINT('Ctrl Pts',(4.78437750874136,-5.11575470075501,
49.2070247483811));
#274200=CARTESIAN_POINT('Ctrl Pts',(4.78839771848114,-5.12122380413468,
49.2685310710606));
#274201=CARTESIAN_POINT('Ctrl Pts',(4.79296103895619,-5.12500019719681,
49.3302745518474));
#274202=CARTESIAN_POINT('Origin',(4.76104848420342,-17.542318193471,0.972561099047131));
#274203=CARTESIAN_POINT('Origin',(15.4290484842034,-17.542318193471,0.972561099047131));
#274204=CARTESIAN_POINT('',(4.79296103895619,0.835811325126388,47.3934894827125));
#274205=CARTESIAN_POINT('',(4.76104848420342,0.161594739351947,46.7718693063203));
#274206=CARTESIAN_POINT('Ctrl Pts',(4.79296103895619,0.835811325126386,
47.3934894827125));
#274207=CARTESIAN_POINT('Ctrl Pts',(4.77035892158032,0.640925346662839,
47.1570738860987));
#274208=CARTESIAN_POINT('Ctrl Pts',(4.76104848420342,0.414296233119738,
46.947837979825));
#274209=CARTESIAN_POINT('Ctrl Pts',(4.76104848420342,0.161594739351935,
46.7718693063203));
#274210=CARTESIAN_POINT('Ctrl Pts',(6.14788848420341,4.21658387552238,50.7898507289224));
#274211=CARTESIAN_POINT('Ctrl Pts',(6.12358695752485,4.17970661397612,50.7591654428809));
#274212=CARTESIAN_POINT('Ctrl Pts',(6.09957618354499,4.14280199669011,50.7282820298215));
#274213=CARTESIAN_POINT('Ctrl Pts',(5.43709796638899,3.11137019184759,49.860149865255));
#274214=CARTESIAN_POINT('Ctrl Pts',(5.01156238585601,2.10608555445921,48.8805868107746));
#274215=CARTESIAN_POINT('Ctrl Pts',(4.82218298524757,1.05648896969834,47.6584541032213));
#274216=CARTESIAN_POINT('Ctrl Pts',(4.80568122363092,0.945490679292535,
47.5265411786623));
#274217=CARTESIAN_POINT('Ctrl Pts',(4.79296103895619,0.835811325126389,
47.3934894827125));
#274218=CARTESIAN_POINT('',(4.79296103895619,4.65778558018571,45.6918369098494));
#274219=CARTESIAN_POINT('Ctrl Pts',(4.79296103895619,4.65778558018571,45.6918369098494));
#274220=CARTESIAN_POINT('Ctrl Pts',(4.80658157259404,4.68507643584799,45.874444288963));
#274221=CARTESIAN_POINT('Ctrl Pts',(4.8245384335836,4.71038602975262,46.0573089564828));
#274222=CARTESIAN_POINT('Ctrl Pts',(5.02532215959839,4.92073119843806,47.7081422117426));
#274223=CARTESIAN_POINT('Ctrl Pts',(5.47477154367343,4.97144972769511,49.1490477246912));
#274224=CARTESIAN_POINT('Ctrl Pts',(6.14788848420341,4.91959547915065,50.4768497968823));
#274225=CARTESIAN_POINT('',(4.76104848420342,4.64697071554394,44.7748512573258));
#274226=CARTESIAN_POINT('Ctrl Pts',(4.76104848420342,4.64697071554394,44.7748512573258));
#274227=CARTESIAN_POINT('Ctrl Pts',(4.76104848420342,4.63156563905975,44.8976814471172));
#274228=CARTESIAN_POINT('Ctrl Pts',(4.76253142587583,4.62292954634033,45.0213551478097));
#274229=CARTESIAN_POINT('Ctrl Pts',(4.7658253855249,4.6211389269688,45.1453609704439));
#274230=CARTESIAN_POINT('Ctrl Pts',(4.76903268308216,4.61939541771304,45.2661042746713));
#274231=CARTESIAN_POINT('Ctrl Pts',(4.77395740161648,4.62414211204842,45.3871622545849));
#274232=CARTESIAN_POINT('Ctrl Pts',(4.78086996580786,4.6354608385096,45.5080274415206));
#274233=CARTESIAN_POINT('Ctrl Pts',(4.78437833171589,4.64120548448167,45.5693707129278));
#274234=CARTESIAN_POINT('Ctrl Pts',(4.78839818488759,4.64864319302931,45.6306637689947));
#274235=CARTESIAN_POINT('Ctrl Pts',(4.79296103895619,4.65778558018572,45.6918369098494));
#274236=CARTESIAN_POINT('Origin',(4.76104848420342,-17.542318193471,0.972561099047131));
#274237=CARTESIAN_POINT('Origin',(15.4290484842034,-17.542318193471,0.972561099047131));
#274238=CARTESIAN_POINT('',(4.79296103895619,10.0856588106982,42.5580528390859));
#274239=CARTESIAN_POINT('',(4.76104848420342,9.29693337302781,42.0901940653058));
#274240=CARTESIAN_POINT('Ctrl Pts',(4.79296103895619,10.0856588106982,42.5580528390859));
#274241=CARTESIAN_POINT('Ctrl Pts',(4.77035892158037,9.84587799202021,42.3673225637814));
#274242=CARTESIAN_POINT('Ctrl Pts',(4.76104848420342,9.58069867729854,42.2097778062576));
#274243=CARTESIAN_POINT('Ctrl Pts',(4.76104848420342,9.29693337302781,42.0901940653058));
#274244=CARTESIAN_POINT('Ctrl Pts',(6.14788848420341,14.0986965788221,45.1772933060682));
#274245=CARTESIAN_POINT('Ctrl Pts',(6.12358695752485,14.0562453442149,45.1549457809498));
#274246=CARTESIAN_POINT('Ctrl Pts',(6.099576183545,14.0137261587332,45.1324101459422));
#274247=CARTESIAN_POINT('Ctrl Pts',(5.43709796638899,12.8243387873176,44.4976954825596));
#274248=CARTESIAN_POINT('Ctrl Pts',(5.01156238585602,11.637359420282,43.7485486597646));
#274249=CARTESIAN_POINT('Ctrl Pts',(4.82218298524757,10.3566033615287,42.7713458847073));
#274250=CARTESIAN_POINT('Ctrl Pts',(4.80568122363092,10.2206044108969,42.6653934162803));
#274251=CARTESIAN_POINT('Ctrl Pts',(4.79296103895619,10.0856588106982,42.5580528390859));
#274252=CARTESIAN_POINT('',(4.79296103895619,13.4703202947425,40.098952328026));
#274253=CARTESIAN_POINT('Ctrl Pts',(4.79296103895619,13.4703202947425,40.098952328026));
#274254=CARTESIAN_POINT('Ctrl Pts',(4.80658157259404,13.5349809886778,40.2718952098376));
#274255=CARTESIAN_POINT('Ctrl Pts',(4.8245384335836,13.597757209446,40.4455016851685));
#274256=CARTESIAN_POINT('Ctrl Pts',(5.02532215959839,14.1467333648809,42.0165270533357));
#274257=CARTESIAN_POINT('Ctrl Pts',(5.47477154367343,14.4959246740922,43.4154003485369));
#274258=CARTESIAN_POINT('Ctrl Pts',(6.14788848420341,14.7212691391912,44.7249678641909));
#274259=CARTESIAN_POINT('',(4.76104848420342,13.2690897233691,39.2042535488964));
#274260=CARTESIAN_POINT('Ctrl Pts',(4.76104848420342,13.2690897233691,39.2042535488964));
#274261=CARTESIAN_POINT('Ctrl Pts',(4.76104848420342,13.2795592535557,39.3276041062441));
#274262=CARTESIAN_POINT('Ctrl Pts',(4.76253146428083,13.2968253885752,39.4503723241485));
#274263=CARTESIAN_POINT('Ctrl Pts',(4.76582551084842,13.3208566282573,39.5720421023193));
#274264=CARTESIAN_POINT('Ctrl Pts',(4.76903289751316,13.3442556531684,39.6905109873215));
#274265=CARTESIAN_POINT('Ctrl Pts',(4.77395775595489,13.3740686583141,39.807938232017));
#274266=CARTESIAN_POINT('Ctrl Pts',(4.78087052304866,13.4102701796273,39.923810455727));
#274267=CARTESIAN_POINT('Ctrl Pts',(4.78437875699033,13.4286424760013,39.9826156870622));
#274268=CARTESIAN_POINT('Ctrl Pts',(4.78839842591226,13.4486602237479,40.041019836584));
#274269=CARTESIAN_POINT('Ctrl Pts',(4.79296103895619,13.4703202947425,40.098952328026));
#274270=CARTESIAN_POINT('Origin',(4.76104848420342,-17.542318193471,0.972561099047131));
#274271=CARTESIAN_POINT('Origin',(15.4290484842034,-17.542318193471,0.972561099047131));
#274272=CARTESIAN_POINT('',(4.79296103895619,26.7032738510938,24.1023216086087));
#274273=CARTESIAN_POINT('Ctrl Pts',(4.79296103895619,26.7032738510938,24.1023216086087));
#274274=CARTESIAN_POINT('Ctrl Pts',(4.80658157259404,26.8326865415184,24.2340129191292));
#274275=CARTESIAN_POINT('Ctrl Pts',(4.8245384335836,26.9606475878415,24.3670769367848));
#274276=CARTESIAN_POINT('Ctrl Pts',(5.02532215959839,28.1011558454284,25.578991307125));
#274277=CARTESIAN_POINT('Ctrl Pts',(5.47477154367343,28.9891310079851,26.7148967508737));
#274278=CARTESIAN_POINT('Ctrl Pts',(6.14788848420341,29.7276425156794,27.8195903550057));
#274279=CARTESIAN_POINT('',(4.76104848420342,26.1555337986896,23.3668214500611));
#274280=CARTESIAN_POINT('Ctrl Pts',(4.76104848420342,26.1555337986896,23.3668214500611));
#274281=CARTESIAN_POINT('Ctrl Pts',(4.76104848420342,26.2152697101275,23.475250045361));
#274282=CARTESIAN_POINT('Ctrl Pts',(4.76253148048463,26.2809778173993,23.5803821574501));
#274283=CARTESIAN_POINT('Ctrl Pts',(4.76582556302885,26.3524194305639,23.6817591254482));
#274284=CARTESIAN_POINT('Ctrl Pts',(4.76903298691825,26.4219816026365,23.7804691318395));
#274285=CARTESIAN_POINT('Ctrl Pts',(4.77395790368511,26.4969796196788,23.8756186960783));
#274286=CARTESIAN_POINT('Ctrl Pts',(4.78087075471303,26.5771814108115,23.9667491847313));
#274287=CARTESIAN_POINT('Ctrl Pts',(4.78437893387748,26.617882743947,24.0129966852556));
#274288=CARTESIAN_POINT('Ctrl Pts',(4.78839852622406,26.6599240776223,24.0582085586405));
#274289=CARTESIAN_POINT('Ctrl Pts',(4.79296103895619,26.7032738510938,24.1023216086087));
#274290=CARTESIAN_POINT('',(4.76104848420342,23.70060616555,27.6188808395637));
#274291=CARTESIAN_POINT('Origin',(4.76104848420342,-17.542318193471,0.972561099047131));
#274292=CARTESIAN_POINT('',(4.79296103895619,24.6114380135418,27.7254875603422));
#274293=CARTESIAN_POINT('Ctrl Pts',(4.79296103895619,24.6114380135418,27.7254875603422));
#274294=CARTESIAN_POINT('Ctrl Pts',(4.77035892158035,24.3148103438982,27.6487744289659));
#274295=CARTESIAN_POINT('Ctrl Pts',(4.76104848420342,24.008477759664,27.6127082756377));
#274296=CARTESIAN_POINT('Ctrl Pts',(4.76104848420342,23.70060616555,27.6188808395637));
#274297=CARTESIAN_POINT('Ctrl Pts',(6.14788848420342,29.3428715129083,28.4860332810845));
#274298=CARTESIAN_POINT('Ctrl Pts',(6.12358695752486,29.2950008230139,28.4828842736815));
#274299=CARTESIAN_POINT('Ctrl Pts',(6.099576183545,29.2469915457218,28.4795910574544));
#274300=CARTESIAN_POINT('Ctrl Pts',(5.43709796638904,27.9022704036925,28.3835177865884));
#274301=CARTESIAN_POINT('Ctrl Pts',(5.01156238585603,26.5132053307471,28.181926112665));
#274302=CARTESIAN_POINT('Ctrl Pts',(4.82218298524757,24.9457122745935,27.8101373762519));
#274303=CARTESIAN_POINT('Ctrl Pts',(4.80568122363092,24.7783762996661,27.7686607366362));
#274304=CARTESIAN_POINT('Ctrl Pts',(4.79296103895619,24.6114380135418,27.7254875603422));
#274305=CARTESIAN_POINT('Origin',(15.4290484842034,-17.542318193471,0.972561099047131));
#274306=CARTESIAN_POINT('',(4.76104848420342,28.3394307068727,18.4617086838663));
#274307=CARTESIAN_POINT('Ctrl Pts',(4.79296103895619,29.2525234772273,18.3766132024512));
#274308=CARTESIAN_POINT('Ctrl Pts',(4.77035892158037,28.9464282770021,18.3632487973896));
#274309=CARTESIAN_POINT('Ctrl Pts',(4.76104848420342,28.639291219787,18.3916609015845));
#274310=CARTESIAN_POINT('Ctrl Pts',(4.76104848420342,28.3394307068727,18.4617086838663));
#274311=CARTESIAN_POINT('',(4.79296103895618,30.5453491237196,14.397704993804));
#274312=CARTESIAN_POINT('Ctrl Pts',(4.79296103895619,30.5453491237196,14.397704993804));
#274313=CARTESIAN_POINT('Ctrl Pts',(4.80658157259404,30.6993139993992,14.4996121219477));
#274314=CARTESIAN_POINT('Ctrl Pts',(4.8245384335836,30.8521443547454,14.6031637740616));
#274315=CARTESIAN_POINT('Ctrl Pts',(5.02532215959839,32.2197009363848,15.5514699074782));
#274316=CARTESIAN_POINT('Ctrl Pts',(5.47477154367344,33.3244397325698,16.4779326744902));
#274317=CARTESIAN_POINT('Ctrl Pts',(6.14788848420341,34.276491707006,17.4049408966648));
#274318=CARTESIAN_POINT('',(4.76104848420342,29.8566594240743,13.7921588388053));
#274319=CARTESIAN_POINT('Ctrl Pts',(4.76104848420342,29.8566594240743,13.7921588388053));
#274320=CARTESIAN_POINT('Ctrl Pts',(4.76104848420342,29.9376329966339,13.8857975921032));
#274321=CARTESIAN_POINT('Ctrl Pts',(4.76253146088426,30.0237628247058,13.9749702764883));
#274322=CARTESIAN_POINT('Ctrl Pts',(4.76582549808585,30.1147200651718,14.0592778788154));
#274323=CARTESIAN_POINT('Ctrl Pts',(4.76903287597333,30.2032844085363,14.1413675222838));
#274324=CARTESIAN_POINT('Ctrl Pts',(4.77395772034131,30.2964254868314,14.2188444200085));
#274325=CARTESIAN_POINT('Ctrl Pts',(4.78087046544997,30.3938209389826,14.2913082108793));
#274326=CARTESIAN_POINT('Ctrl Pts',(4.78437871324177,30.443249548684,14.3280838955475));
#274327=CARTESIAN_POINT('Ctrl Pts',(4.78839840126576,30.4937736154865,14.3635679095932));
#274328=CARTESIAN_POINT('Ctrl Pts',(4.79296103895619,30.5453491237196,14.397704993804));
#274329=CARTESIAN_POINT('Origin',(4.76104848420342,-17.542318193471,0.972561099047131));
#274330=CARTESIAN_POINT('Origin',(15.4290484842034,-17.542318193471,0.972561099047131));
#274331=CARTESIAN_POINT('',(4.79296103895619,18.1280311274453,35.9051306570905));
#274332=CARTESIAN_POINT('',(4.76104848420342,17.2592679242297,35.6114809593723));
#274333=CARTESIAN_POINT('Ctrl Pts',(4.79296103895619,18.1280311274453,35.9051306570905));
#274334=CARTESIAN_POINT('Ctrl Pts',(4.77035892158039,17.853835040925,35.7684215313513));
#274335=CARTESIAN_POINT('Ctrl Pts',(4.76104848420342,17.5616951335496,35.6694533844648));
#274336=CARTESIAN_POINT('Ctrl Pts',(4.76104848420342,17.2592679242297,35.6114809593723));
#274337=CARTESIAN_POINT('Ctrl Pts',(6.14788848420341,22.5979451061385,37.632776967928));
#274338=CARTESIAN_POINT('Ctrl Pts',(6.12358695752485,22.5517752211263,37.6197438978156));
#274339=CARTESIAN_POINT('Ctrl Pts',(6.099576183545,22.5054997598841,37.6065409562476));
#274340=CARTESIAN_POINT('Ctrl Pts',(5.43709796638902,21.2101387573402,37.2329838705376));
#274341=CARTESIAN_POINT('Ctrl Pts',(5.01156238585603,19.8933413547557,36.7469945903896));
#274342=CARTESIAN_POINT('Ctrl Pts',(4.82218298524757,18.4374010075269,36.0574301982373));
#274343=CARTESIAN_POINT('Ctrl Pts',(4.80568122363092,18.2823452034071,35.9820688172288));
#274344=CARTESIAN_POINT('Ctrl Pts',(4.79296103895619,18.1280311274453,35.9051306570905));
#274345=CARTESIAN_POINT('',(4.79296103895619,20.927453892214,32.7960567002406));
#274346=CARTESIAN_POINT('Ctrl Pts',(4.79296103895619,20.927453892214,32.7960567002406));
#274347=CARTESIAN_POINT('Ctrl Pts',(4.80658157259404,21.026658441821,32.9517766509431));
#274348=CARTESIAN_POINT('Ctrl Pts',(4.8245384335836,21.1241576673716,33.1085374980568));
#274349=CARTESIAN_POINT('Ctrl Pts',(5.02532215959839,21.9877719172835,34.5310936319264));
#274350=CARTESIAN_POINT('Ctrl Pts',(5.47477154367344,22.6201746706307,35.826797233841));
#274351=CARTESIAN_POINT('Ctrl Pts',(6.1478884842034,23.1128692149255,37.0608958085218));
#274352=CARTESIAN_POINT('',(4.76104848420342,20.5446023556894,31.962747424394));
#274353=CARTESIAN_POINT('Ctrl Pts',(4.76104848420342,20.5446023556894,31.962747424394));
#274354=CARTESIAN_POINT('Ctrl Pts',(4.76104848420342,20.5804893278971,32.0812264100145));
#274355=CARTESIAN_POINT('Ctrl Pts',(4.76253148100033,20.6229033704963,32.197722642335));
#274356=CARTESIAN_POINT('Ctrl Pts',(4.76582556519821,20.6717063717276,32.3117378555962));
#274357=CARTESIAN_POINT('Ctrl Pts',(4.76903299054366,20.7192254919687,32.422753622897));
#274358=CARTESIAN_POINT('Ctrl Pts',(4.77395790968128,20.7728019328613,32.5314169312464));
#274359=CARTESIAN_POINT('Ctrl Pts',(4.78087076460355,20.8323040513083,32.6372309180115));
#274360=CARTESIAN_POINT('Ctrl Pts',(4.78437894136499,20.8625005405358,32.6909300298225));
#274361=CARTESIAN_POINT('Ctrl Pts',(4.78839853042471,20.8942230647019,32.743894749579));
#274362=CARTESIAN_POINT('Ctrl Pts',(4.79296103895619,20.927453892214,32.7960567002406));
#274363=CARTESIAN_POINT('Origin',(4.76104848420342,-17.542318193471,0.972561099047131));
#274364=CARTESIAN_POINT('Origin',(15.4290484842034,-17.542318193471,0.972561099047131));
#274365=CARTESIAN_POINT('',(4.79296103895619,-67.370398971297,-2.16122297171674));
#274366=CARTESIAN_POINT('Ctrl Pts',(4.79296103895618,-67.370398971297,-2.16122297171673));
#274367=CARTESIAN_POINT('Ctrl Pts',(4.80658157259404,-67.5421870283591,
-2.22889208697901));
#274368=CARTESIAN_POINT('Ctrl Pts',(4.8245384335836,-67.7132072728381,-2.29840566945804));
#274369=CARTESIAN_POINT('Ctrl Pts',(5.02532215959839,-69.248043393648,-2.94165803744303));
#274370=CARTESIAN_POINT('Ctrl Pts',(5.47477154367342,-70.521263436943,-3.61818725913814));
#274371=CARTESIAN_POINT('Ctrl Pts',(6.14788848420341,-71.6452466383859,
-4.32699539176736));
#274372=CARTESIAN_POINT('',(4.76104848420342,-66.5708586689849,-1.71209609297323));
#274373=CARTESIAN_POINT('Ctrl Pts',(4.76104848420342,-66.5708586689849,
-1.71209609297323));
#274374=CARTESIAN_POINT('Ctrl Pts',(4.76104848420342,-66.669531832499,-1.78685361572226));
#274375=CARTESIAN_POINT('Ctrl Pts',(4.76253147480136,-66.7723200664169,
-1.85617057016433));
#274376=CARTESIAN_POINT('Ctrl Pts',(4.76582554519776,-66.8788187601492,
-1.91972502885798));
#274377=CARTESIAN_POINT('Ctrl Pts',(4.76903295628211,-66.9825157215496,
-1.98160751791974));
#274378=CARTESIAN_POINT('Ctrl Pts',(4.77395785306817,-67.0897304064449,
-2.03802645188551));
#274379=CARTESIAN_POINT('Ctrl Pts',(4.78087067578871,-67.2000642630108,
-2.08865723673717));
#274380=CARTESIAN_POINT('Ctrl Pts',(4.78437887355539,-67.2560577413395,
-2.11435192232688));
#274381=CARTESIAN_POINT('Ctrl Pts',(4.78839849197368,-67.3128541568119,
-2.13855546647373));
#274382=CARTESIAN_POINT('Ctrl Pts',(4.79296103895619,-67.370398971297,-2.16122297171674));
#274383=CARTESIAN_POINT('',(4.76104848420342,-66.0576390431341,-6.59505465837713));
#274384=CARTESIAN_POINT('Origin',(4.76104848420342,-17.542318193471,0.972561099047131));
#274385=CARTESIAN_POINT('',(4.79296103895619,-66.9330862002819,-6.32197605563978));
#274386=CARTESIAN_POINT('Ctrl Pts',(4.79296103895618,-66.9330862002819,
-6.32197605563978));
#274387=CARTESIAN_POINT('Ctrl Pts',(4.77035892158033,-66.6309012985319,
-6.37254446552365));
#274388=CARTESIAN_POINT('Ctrl Pts',(4.76104848420342,-66.3363831315434,
-6.46419308195223));
#274389=CARTESIAN_POINT('Ctrl Pts',(4.76104848420342,-66.0576390431341,
-6.59505465837713));
#274390=CARTESIAN_POINT('Ctrl Pts',(6.14788848420341,-71.5648075951267,
-5.0923217656847));
#274391=CARTESIAN_POINT('Ctrl Pts',(6.12358695752485,-71.5197947271193,
-5.10891576798505));
#274392=CARTESIAN_POINT('Ctrl Pts',(6.099576183545,-71.4745965982113,-5.12543439754196));
#274393=CARTESIAN_POINT('Ctrl Pts',(5.43709796638902,-70.2070561874331,
-5.58461446052352));
#274394=CARTESIAN_POINT('Ctrl Pts',(5.01156238585603,-68.8560873789502,
-5.96543496729592));
#274395=CARTESIAN_POINT('Ctrl Pts',(4.82218298524757,-67.2728911150327,
-6.26334591964759));
#274396=CARTESIAN_POINT('Ctrl Pts',(4.80568122363092,-67.1031520260742,
-6.29351679663613));
#274397=CARTESIAN_POINT('Ctrl Pts',(4.79296103895619,-66.933086200282,-6.32197605563978));
#274398=CARTESIAN_POINT('Origin',(15.4290484842034,-17.542318193471,0.972561099047131));
#274399=CARTESIAN_POINT('',(4.79296103895619,-67.370398971297,4.1063451698103));
#274400=CARTESIAN_POINT('',(4.76104848420342,-66.570858668985,3.65721829106681));
#274401=CARTESIAN_POINT('Ctrl Pts',(4.79296103895618,-67.370398971297,4.1063451698103));
#274402=CARTESIAN_POINT('Ctrl Pts',(4.7703589215748,-67.0853312982033,3.99405402711951));
#274403=CARTESIAN_POINT('Ctrl Pts',(4.76104848420342,-66.8163038786029,
3.84317438275566));
#274404=CARTESIAN_POINT('Ctrl Pts',(4.76104848420342,-66.570858668985,3.65721829106682));
#274405=CARTESIAN_POINT('Ctrl Pts',(6.14788848420341,-71.645246638386,6.27211758986087));
#274406=CARTESIAN_POINT('Ctrl Pts',(6.12358695752485,-71.6046674966181,
6.24652750482824));
#274407=CARTESIAN_POINT('Ctrl Pts',(6.099576183545,-71.5638914714703,6.22097262755666));
#274408=CARTESIAN_POINT('Ctrl Pts',(5.43709796638903,-70.4195187631187,
5.50829028066173));
#274409=CARTESIAN_POINT('Ctrl Pts',(5.01156238585603,-69.1772488998961,
4.85490940643834));
#274410=CARTESIAN_POINT('Ctrl Pts',(4.82218298524757,-67.6905884426711,
4.23434351103579));
#274411=CARTESIAN_POINT('Ctrl Pts',(4.80568122363092,-67.5308314381037,
4.16954119911417));
#274412=CARTESIAN_POINT('Ctrl Pts',(4.79296103895618,-67.370398971297,4.1063451698103));
#274413=CARTESIAN_POINT('',(4.79296103895619,-66.933086200282,8.26709825373337));
#274414=CARTESIAN_POINT('Ctrl Pts',(4.79296103895619,-66.933086200282,8.26709825373337));
#274415=CARTESIAN_POINT('Ctrl Pts',(4.80658157259404,-67.1151894763023,
8.23662461640187));
#274416=CARTESIAN_POINT('Ctrl Pts',(4.8245384335836,-67.2969252045845,8.20418718067529));
#274417=CARTESIAN_POINT('Ctrl Pts',(5.02532215959839,-68.9319611611245,
7.89410179327018));
#274418=CARTESIAN_POINT('Ctrl Pts',(5.47477154367344,-70.31801662605,7.49707369022733));
#274419=CARTESIAN_POINT('Ctrl Pts',(6.14788848420342,-71.5648075951268,
7.03744396377821));
#274420=CARTESIAN_POINT('',(4.76104848420342,-66.0576390431342,8.54017685647074));
#274421=CARTESIAN_POINT('Ctrl Pts',(4.76104848420342,-66.0576390431342,
8.54017685647073));
#274422=CARTESIAN_POINT('Ctrl Pts',(4.76104848420342,-66.1696919168572,
8.48757155896645));
#274423=CARTESIAN_POINT('Ctrl Pts',(4.76253129040183,-66.2846386577921,
8.44114267243526));
#274424=CARTESIAN_POINT('Ctrl Pts',(4.76582494299244,-66.4020164824655,
8.40112098163002));
#274425=CARTESIAN_POINT('Ctrl Pts',(4.76903192598719,-66.5163056120359,
8.3621524267195));
#274426=CARTESIAN_POINT('Ctrl Pts',(4.77395615055237,-66.6328994339606,
8.32925854949861));
#274427=CARTESIAN_POINT('Ctrl Pts',(4.7808679979395,-66.7513405603554,8.30267399608132));
#274428=CARTESIAN_POINT('Ctrl Pts',(4.78437682990909,-66.8114677575475,
8.2891782219846));
#274429=CARTESIAN_POINT('Ctrl Pts',(4.78839733376406,-66.8720705537315,
8.27730877122192));
#274430=CARTESIAN_POINT('Ctrl Pts',(4.79296103895619,-66.933086200282,8.26709825373337));
#274431=CARTESIAN_POINT('Origin',(4.76104848420342,-17.542318193471,0.972561099047131));
#274432=CARTESIAN_POINT('Origin',(15.4290484842034,-17.542318193471,0.972561099047131));
#274433=CARTESIAN_POINT('',(4.79296103895619,-65.6299855106617,14.3977049938037));
#274434=CARTESIAN_POINT('',(4.76104848420342,-64.9412958110163,13.792158838805));
#274435=CARTESIAN_POINT('Ctrl Pts',(4.79296103895619,-65.6299855106617,
14.3977049938037));
#274436=CARTESIAN_POINT('Ctrl Pts',(4.77035892158033,-65.3744938915815,
14.228598780128));
#274437=CARTESIAN_POINT('Ctrl Pts',(4.76104848420342,-65.1427150085247,
14.0250822723247));
#274438=CARTESIAN_POINT('Ctrl Pts',(4.76104848420342,-64.9412958110163,
13.792158838805));
#274439=CARTESIAN_POINT('Ctrl Pts',(6.14788848420341,-69.361128093948,17.4049408966644));
#274440=CARTESIAN_POINT('Ctrl Pts',(6.12358695752485,-69.3267561816353,
17.3714731384103));
#274441=CARTESIAN_POINT('Ctrl Pts',(6.099576183545,-69.2921843682116,17.3379988841867));
#274442=CARTESIAN_POINT('Ctrl Pts',(5.437097966389,-68.3209939409511,16.402961891767));
#274443=CARTESIAN_POINT('Ctrl Pts',(5.01156238585602,-67.2417161770838,
15.5055765295655));
#274444=CARTESIAN_POINT('Ctrl Pts',(4.82218298524757,-65.9165657223203,
14.5894773985467));
#274445=CARTESIAN_POINT('Ctrl Pts',(4.80568122363092,-65.7737729498428,
14.492875823679));
#274446=CARTESIAN_POINT('Ctrl Pts',(4.79296103895619,-65.6299855106617,
14.3977049938037));
#274447=CARTESIAN_POINT('',(4.76104848420342,-63.4240670938148,18.461708683866));
#274448=CARTESIAN_POINT('Ctrl Pts',(4.76104848420342,-63.4240670938148,
18.461708683866));
#274449=CARTESIAN_POINT('Ctrl Pts',(4.76104848420342,-63.5446128669712,
18.4335490439355));
#274450=CARTESIAN_POINT('Ctrl Pts',(4.76253139478368,-63.6667050910714,
18.4120329930263));
#274451=CARTESIAN_POINT('Ctrl Pts',(4.76582528398501,-63.7898431598502,
18.3972900560778));
#274452=CARTESIAN_POINT('Ctrl Pts',(4.76903250936003,-63.9097414061722,
18.3829350129682));
#274453=CARTESIAN_POINT('Ctrl Pts',(4.7739571145476,-64.0306310087032,18.3750015769542));
#274454=CARTESIAN_POINT('Ctrl Pts',(4.78086951428214,-64.1520158222007,
18.3736241726316));
#274455=CARTESIAN_POINT('Ctrl Pts',(4.78437798712838,-64.2136261657077,
18.3729250542574));
#274456=CARTESIAN_POINT('Ctrl Pts',(4.78839798959814,-64.2753635517415,
18.373915117182));
#274457=CARTESIAN_POINT('Ctrl Pts',(4.79296103895619,-64.3371598641695,
18.3766132024509));
#274458=CARTESIAN_POINT('Origin',(4.76104848420342,-17.542318193471,0.972561099047131));
#274459=CARTESIAN_POINT('Origin',(15.4290484842034,-17.542318193471,0.972561099047131));
#274460=CARTESIAN_POINT('',(4.79296103895619,-59.6960744004839,27.7254875603419));
#274461=CARTESIAN_POINT('Ctrl Pts',(4.79296103895618,-59.6960744004839,
27.7254875603419));
#274462=CARTESIAN_POINT('Ctrl Pts',(4.80658157259404,-59.8748287660646,
27.7717165825615));
#274463=CARTESIAN_POINT('Ctrl Pts',(4.8245384335836,-60.0540461088455,27.8160020905443));
#274464=CARTESIAN_POINT('Ctrl Pts',(5.0253221595984,-61.673848869565,28.1977540296704));
#274465=CARTESIAN_POINT('Ctrl Pts',(5.47477154367345,-63.1015594214269,
28.3988103564998));
#274466=CARTESIAN_POINT('Ctrl Pts',(6.14788848420342,-64.4275078998505,
28.4860332810842));
#274467=CARTESIAN_POINT('',(4.76104848420342,-58.7852425524921,27.6188808395635));
#274468=CARTESIAN_POINT('Ctrl Pts',(4.76104848420342,-58.7852425524921,
27.6188808395635));
#274469=CARTESIAN_POINT('Ctrl Pts',(4.76104848420342,-58.9090110779737,
27.6163993857685));
#274470=CARTESIAN_POINT('Ctrl Pts',(4.76253144835227,-59.0329109135381,
27.6207381048775));
#274471=CARTESIAN_POINT('Ctrl Pts',(4.7658254588955,-59.1564254863122,27.6319196149988));
#274472=CARTESIAN_POINT('Ctrl Pts',(4.76903280861577,-59.2766905629532,
27.6428069551847));
#274473=CARTESIAN_POINT('Ctrl Pts',(4.77395760905528,-59.3965901622967,
27.6601819444716));
#274474=CARTESIAN_POINT('Ctrl Pts',(4.7808702920541,-59.5156110492459,27.6840729200258));
#274475=CARTESIAN_POINT('Ctrl Pts',(4.78437858069741,-59.5760159059524,
27.6961979427165));
#274476=CARTESIAN_POINT('Ctrl Pts',(4.78839832599606,-59.6361938640674,
27.710001400664));
#274477=CARTESIAN_POINT('Ctrl Pts',(4.79296103895619,-59.6960744004839,
27.7254875603419));
#274478=CARTESIAN_POINT('',(4.76104848420342,-61.2401701856317,23.3668214500608));
#274479=CARTESIAN_POINT('Origin',(4.76104848420342,-17.542318193471,0.972561099047131));
#274480=CARTESIAN_POINT('',(4.79296103895619,-61.7879102380359,24.1023216086084));
#274481=CARTESIAN_POINT('Ctrl Pts',(4.79296103895618,-61.7879102380359,
24.1023216086084));
#274482=CARTESIAN_POINT('Ctrl Pts',(4.77035892157486,-61.5731608825862,
23.8837910768667));
#274483=CARTESIAN_POINT('Ctrl Pts',(4.76104848420342,-61.3887603854858,
23.636532353564));
#274484=CARTESIAN_POINT('Ctrl Pts',(4.76104848420342,-61.2401701856317,
23.3668214500608));
#274485=CARTESIAN_POINT('Ctrl Pts',(6.14788848420341,-64.8122789026216,
27.8195903550054));
#274486=CARTESIAN_POINT('Ctrl Pts',(6.12358695752485,-64.7856164372667,
27.7797076251616));
#274487=CARTESIAN_POINT('Ctrl Pts',(6.099576183545,-64.7587597897078,27.7397769795229));
#274488=CARTESIAN_POINT('Ctrl Pts',(5.43709796638903,-64.0031973254985,
26.6232509449525));
#274489=CARTESIAN_POINT('Ctrl Pts',(5.01156238585602,-63.1340812782167,
25.5210811412337));
#274490=CARTESIAN_POINT('Ctrl Pts',(4.82218298524757,-62.0283562595653,
24.3494867025556));
#274491=CARTESIAN_POINT('Ctrl Pts',(4.80568122363092,-61.9087684485308,
24.2253078171093));
#274492=CARTESIAN_POINT('Ctrl Pts',(4.79296103895619,-61.7879102380359,
24.1023216086084));
#274493=CARTESIAN_POINT('Origin',(15.4290484842034,-17.542318193471,0.972561099047131));
#274494=CARTESIAN_POINT('',(4.79296103895619,-56.0120902791562,32.7960567002403));
#274495=CARTESIAN_POINT('',(4.76104848420342,-55.6292387426316,31.9627474243937));
#274496=CARTESIAN_POINT('Ctrl Pts',(4.79296103895618,-56.0120902791562,
32.7960567002403));
#274497=CARTESIAN_POINT('Ctrl Pts',(4.77035892158035,-55.8474687647536,
32.5376526833993));
#274498=CARTESIAN_POINT('Ctrl Pts',(4.76104848420342,-55.718505840154,32.25745813731));
#274499=CARTESIAN_POINT('Ctrl Pts',(4.76104848420342,-55.6292387426316,
31.9627474243937));
#274500=CARTESIAN_POINT('Ctrl Pts',(6.14788848420341,-58.1975056018678,
37.0608958085216));
#274501=CARTESIAN_POINT('Ctrl Pts',(6.12358695752485,-58.1797178611475,
37.0163411737608));
#274502=CARTESIAN_POINT('Ctrl Pts',(6.09957618354499,-58.1617501438242,
36.9716992975299));
#274503=CARTESIAN_POINT('Ctrl Pts',(5.43709796638901,-57.6548373479429,
35.7224817662058));
#274504=CARTESIAN_POINT('Ctrl Pts',(5.01156238585602,-57.0338675589944,
34.4636976301899));
#274505=CARTESIAN_POINT('Ctrl Pts',(4.82218298524757,-56.1958934656274,
33.0878121827565));
#274506=CARTESIAN_POINT('Ctrl Pts',(4.80568122363092,-56.104737177224,32.941483199902));
#274507=CARTESIAN_POINT('Ctrl Pts',(4.79296103895619,-56.0120902791562,
32.7960567002403));
#274508=CARTESIAN_POINT('',(4.79296103895619,-53.2126675143875,35.9051306570903));
#274509=CARTESIAN_POINT('Ctrl Pts',(4.79296103895618,-53.2126675143875,
35.9051306570903));
#274510=CARTESIAN_POINT('Ctrl Pts',(4.80658157259404,-53.3779041140264,
35.9875145866475));
#274511=CARTESIAN_POINT('Ctrl Pts',(4.8245384335836,-53.543997653034,36.0680937307897));
#274512=CARTESIAN_POINT('Ctrl Pts',(5.02532215959839,-55.0490331459571,
36.7782794048937));
#274513=CARTESIAN_POINT('Ctrl Pts',(5.47477154367343,-56.4037428359424,
37.2717798834302));
#274514=CARTESIAN_POINT('Ctrl Pts',(6.14788848420341,-57.6825814930807,
37.6327769679277));
#274515=CARTESIAN_POINT('',(4.76104848420342,-52.343904311172,35.6114809593721));
#274516=CARTESIAN_POINT('Ctrl Pts',(4.76104848420342,-52.343904311172,35.6114809593721));
#274517=CARTESIAN_POINT('Ctrl Pts',(4.76104848420342,-52.465485215972,35.6347868646577));
#274518=CARTESIAN_POINT('Ctrl Pts',(4.7625314749205,-52.5857765087052,35.6647913142045));
#274519=CARTESIAN_POINT('Ctrl Pts',(4.76582554549142,-52.7042682136469,
35.7014090350176));
#274520=CARTESIAN_POINT('Ctrl Pts',(4.76903295680144,-52.8196426800984,
35.7370634295895));
#274521=CARTESIAN_POINT('Ctrl Pts',(4.77395785392526,-52.9333107491858,
35.778987834308));
#274522=CARTESIAN_POINT('Ctrl Pts',(4.78087067704644,-53.0447645175907,
35.8271032630079));
#274523=CARTESIAN_POINT('Ctrl Pts',(4.78437887452713,-53.1013263336066,
35.851521423691));
#274524=CARTESIAN_POINT('Ctrl Pts',(4.78839849253279,-53.1573172853332,
35.8775340508823));
#274525=CARTESIAN_POINT('Ctrl Pts',(4.79296103895619,-53.2126675143875,
35.9051306570903));
#274526=CARTESIAN_POINT('Origin',(4.76104848420342,-17.542318193471,0.972561099047131));
#274527=CARTESIAN_POINT('Origin',(15.4290484842034,-17.542318193471,0.972561099047131));
#274528=CARTESIAN_POINT('',(4.79296103895619,-45.1702951976404,42.5580528390857));
#274529=CARTESIAN_POINT('Ctrl Pts',(4.79296103895619,-45.1702951976404,
42.5580528390857));
#274530=CARTESIAN_POINT('Ctrl Pts',(4.80658157259404,-45.3147923990402,
42.672991102937));
#274531=CARTESIAN_POINT('Ctrl Pts',(4.8245384335836,-45.4605030496147,42.7863421879778));
#274532=CARTESIAN_POINT('Ctrl Pts',(5.02532215959839,-46.7849940017391,
43.7939230752526));
#274533=CARTESIAN_POINT('Ctrl Pts',(5.47477154367344,-48.0074955157771,
44.5582993665061));
#274534=CARTESIAN_POINT('Ctrl Pts',(6.14788848420341,-49.1833329657644,
45.177293306068));
#274535=CARTESIAN_POINT('',(4.76104848420342,-44.3815697599701,42.0901940653056));
#274536=CARTESIAN_POINT('Ctrl Pts',(4.76104848420342,-44.3815697599701,
42.0901940653057));
#274537=CARTESIAN_POINT('Ctrl Pts',(4.76104848420342,-44.4956485670493,
42.1382689014767));
#274538=CARTESIAN_POINT('Ctrl Pts',(4.76253148285844,-44.6070732100943,
42.1926278033787));
#274539=CARTESIAN_POINT('Ctrl Pts',(4.76582557106135,-44.7153625908546,
42.2530813329808));
#274540=CARTESIAN_POINT('Ctrl Pts',(4.76903300061106,-44.8208031675407,
42.3119444918539));
#274541=CARTESIAN_POINT('Ctrl Pts',(4.7739579263149,-44.9232710031647,42.3765858961933));
#274542=CARTESIAN_POINT('Ctrl Pts',(4.78087079057214,-45.0222857184793,
42.4468226877301));
#274543=CARTESIAN_POINT('Ctrl Pts',(4.78437896120848,-45.0725341399594,
42.4824667623845));
#274544=CARTESIAN_POINT('Ctrl Pts',(4.7883985416886,-45.1218926824315,42.5195517400314));
#274545=CARTESIAN_POINT('Ctrl Pts',(4.79296103895619,-45.1702951976404,
42.5580528390857));
#274546=CARTESIAN_POINT('',(4.76104848420342,-48.3537261103113,39.2042535488962));
#274547=CARTESIAN_POINT('Origin',(4.76104848420342,-17.542318193471,0.972561099047131));
#274548=CARTESIAN_POINT('',(4.79296103895619,-48.5549566816847,40.0989523280257));
#274549=CARTESIAN_POINT('Ctrl Pts',(4.79296103895619,-48.5549566816847,
40.0989523280257));
#274550=CARTESIAN_POINT('Ctrl Pts',(4.77035892158593,-48.4476577584246,
39.8119683215992));
#274551=CARTESIAN_POINT('Ctrl Pts',(4.76104848420342,-48.3797687049592,
39.5110837989026));
#274552=CARTESIAN_POINT('Ctrl Pts',(4.76104848420342,-48.3537261103113,
39.2042535488962));
#274553=CARTESIAN_POINT('Ctrl Pts',(6.14788848420341,-49.8059055261334,
44.7249678641907));
#274554=CARTESIAN_POINT('Ctrl Pts',(6.12358695752485,-49.7977699196723,
44.677688575849));
#274555=CARTESIAN_POINT('Ctrl Pts',(6.099576183545,-49.7894764080503,44.6302865332326));
#274556=CARTESIAN_POINT('Ctrl Pts',(5.43709796638902,-49.5533678021145,
43.3029743056845));
#274557=CARTESIAN_POINT('Ctrl Pts',(5.01156238585602,-49.2076836310201,
41.9425907444318));
#274558=CARTESIAN_POINT('Ctrl Pts',(4.82218298524757,-48.6740839518635,
40.4225470845268));
#274559=CARTESIAN_POINT('Ctrl Pts',(4.80568122363092,-48.6153431533108,
40.2604632829792));
#274560=CARTESIAN_POINT('Ctrl Pts',(4.79296103895619,-48.5549566816847,
40.0989523280258));
#274561=CARTESIAN_POINT('Origin',(15.4290484842034,-17.542318193471,0.972561099047131));
#274562=CARTESIAN_POINT('',(4.79296103895619,-39.742421967128,45.6918369098492));
#274563=CARTESIAN_POINT('',(4.76104848420342,-39.7316071024862,44.7748512573257));
#274564=CARTESIAN_POINT('Ctrl Pts',(4.79296103895619,-39.742421967128,45.6918369098492));
#274565=CARTESIAN_POINT('Ctrl Pts',(4.77035892158033,-39.6971351127824,
45.3888154918811));
#274566=CARTESIAN_POINT('Ctrl Pts',(4.76104848420342,-39.6932870078947,
45.0803910900121));
#274567=CARTESIAN_POINT('Ctrl Pts',(4.76104848420342,-39.7316071024862,
44.7748512573257));
#274568=CARTESIAN_POINT('Ctrl Pts',(6.14788848420341,-40.004231866093,50.4768497968822));
#274569=CARTESIAN_POINT('Ctrl Pts',(6.12358695752485,-40.0061039589323,
50.4289121867311));
#274570=CARTESIAN_POINT('Ctrl Pts',(6.099576183545,-40.0078471192661,50.3808216744519));
#274571=CARTESIAN_POINT('Ctrl Pts',(5.43709796638902,-40.0528617823301,
49.0334246641744));
#274572=CARTESIAN_POINT('Ctrl Pts',(5.01156238585603,-39.9975712861431,
47.6308969671561));
#274573=CARTESIAN_POINT('Ctrl Pts',(4.82218298524757,-39.7916668876715,
46.0331282966962));
#274574=CARTESIAN_POINT('Ctrl Pts',(4.80568122363092,-39.7679088337358,
45.8623735163475));
#274575=CARTESIAN_POINT('Ctrl Pts',(4.79296103895618,-39.742421967128,45.6918369098492));
#274576=CARTESIAN_POINT('',(4.79296103895619,-35.9204477120687,47.3934894827124));
#274577=CARTESIAN_POINT('Ctrl Pts',(4.79296103895619,-35.9204477120687,
47.3934894827124));
#274578=CARTESIAN_POINT('Ctrl Pts',(4.80658157259404,-36.0378902941536,
47.5359587271926));
#274579=CARTESIAN_POINT('Ctrl Pts',(4.82453843358361,-36.1568498016675,
47.6771277667969));
#274580=CARTESIAN_POINT('Ctrl Pts',(5.02532215959839,-37.2429096027727,
48.938067747559));
#274581=CARTESIAN_POINT('Ctrl Pts',(5.47477154367343,-38.2797737584869,
49.9399129397173));
#274582=CARTESIAN_POINT('Ctrl Pts',(6.14788848420341,-39.3012202624647,
50.7898507289222));
#274583=CARTESIAN_POINT('',(4.76104848420342,-35.2462311262942,46.7718693063201));
#274584=CARTESIAN_POINT('Ctrl Pts',(4.76104848420342,-35.2462311262942,
46.7718693063201));
#274585=CARTESIAN_POINT('Ctrl Pts',(4.76104848420342,-35.3478213939069,
46.8426116844765));
#274586=CARTESIAN_POINT('Ctrl Pts',(4.76253147347933,-35.4455089937174,
46.9189489429545));
#274587=CARTESIAN_POINT('Ctrl Pts',(4.7658255397648,-35.5388627266735,47.00059575335));
#274588=CARTESIAN_POINT('Ctrl Pts',(4.76903294718426,-35.6297605501445,
47.0800946348976));
#274589=CARTESIAN_POINT('Ctrl Pts',(4.77395783802111,-35.7165492566998,
47.1646273892827));
#274590=CARTESIAN_POINT('Ctrl Pts',(4.7808706510644,-35.7987969832442,47.253915274399));
#274591=CARTESIAN_POINT('Ctrl Pts',(4.78437885482598,-35.8405371231608,
47.2992282450329));
#274592=CARTESIAN_POINT('Ctrl Pts',(4.78839848145743,-35.8811072172091,
47.3457656462587));
#274593=CARTESIAN_POINT('Ctrl Pts',(4.79296103895619,-35.9204477120687,
47.3934894827124));
#274594=CARTESIAN_POINT('Origin',(4.76104848420342,-17.542318193471,0.972561099047131));
#274595=CARTESIAN_POINT('Origin',(15.4290484842034,-17.542318193471,0.972561099047131));
#274596=CARTESIAN_POINT('Ctrl Pts',(4.79296103895619,-19.6341540310225,
-48.9101258718094));
#274597=CARTESIAN_POINT('Ctrl Pts',(4.80658157259404,-19.5848123558664,
-49.0880462045495));
#274598=CARTESIAN_POINT('Ctrl Pts',(4.8245384335836,-19.5335560594086,-49.2653957301879));
#274599=CARTESIAN_POINT('Ctrl Pts',(5.02532215959839,-19.0542615562759,
-50.8590620396541));
#274600=CARTESIAN_POINT('Ctrl Pts',(5.47477154367343,-18.5145261669709,
-52.1960238102323));
#274601=CARTESIAN_POINT('Ctrl Pts',(6.14788848420341,-17.9270891962415,
-53.3879403389487));
#274602=CARTESIAN_POINT('Origin',(4.76104848420342,-17.542318193471,0.972561099047131));
#274603=CARTESIAN_POINT('Ctrl Pts',(6.1478884842034,-17.1575471906993,-53.3879403389487));
#274604=CARTESIAN_POINT('Ctrl Pts',(6.12358695752485,-17.1363389661598,
-53.344908601702));
#274605=CARTESIAN_POINT('Ctrl Pts',(6.099576183545,-17.1151863364266,-53.3016847398361));
#274606=CARTESIAN_POINT('Ctrl Pts',(5.43709796638902,-16.5260276586066,
-52.0890854343997));
#274607=CARTESIAN_POINT('Ctrl Pts',(5.01156238585603,-16.0060786329429,
-50.7853239567576));
#274608=CARTESIAN_POINT('Ctrl Pts',(4.82218298524757,-15.5443105954408,
-49.2419407816664));
#274609=CARTESIAN_POINT('Ctrl Pts',(4.80568122363092,-15.496562431548,-49.0762852566043));
#274610=CARTESIAN_POINT('Ctrl Pts',(4.79296103895619,-15.4504823559185,
-48.9101258718094));
#274611=CARTESIAN_POINT('Origin',(15.4290484842034,-17.542318193471,0.972561099047131));
#274612=CARTESIAN_POINT('Ctrl Pts',(6.14788848420341,-28.4681391279529,
-52.280031346979));
#274613=CARTESIAN_POINT('Ctrl Pts',(6.12358695752485,-28.4384475527539,
-52.2423493942589));
#274614=CARTESIAN_POINT('Ctrl Pts',(6.099576183545,-28.408770412527,-52.2044679564935));
#274615=CARTESIAN_POINT('Ctrl Pts',(5.43709796638901,-27.5803726934881,
-51.1408598320948));
#274616=CARTESIAN_POINT('Ctrl Pts',(5.01156238585602,-26.8007185482917,
-49.9736921518748));
#274617=CARTESIAN_POINT('Ctrl Pts',(4.82218298524757,-26.0281538448006,
-48.5600425755891));
#274618=CARTESIAN_POINT('Ctrl Pts',(4.80568122363092,-25.9470073725404,
-48.4079344226897));
#274619=CARTESIAN_POINT('Ctrl Pts',(4.79296103895619,-25.8673877784838,
-48.2549866055504));
#274620=CARTESIAN_POINT('Ctrl Pts',(4.79296103895619,-29.9596361897448,
-47.3851523537532));
#274621=CARTESIAN_POINT('Ctrl Pts',(4.80658157259404,-29.9483644657855,
-47.5694434114541));
#274622=CARTESIAN_POINT('Ctrl Pts',(4.8245384335836,-29.935101282124,-47.7535742077102));
#274623=CARTESIAN_POINT('Ctrl Pts',(5.02532215959839,-29.7976223708404,
-49.4120660152309));
#274624=CARTESIAN_POINT('Ctrl Pts',(5.47477154367343,-29.5476514770401,
-50.8320292607793));
#274625=CARTESIAN_POINT('Ctrl Pts',(6.1478884842034,-29.2208647943379,-52.1200345674514));
#274626=CARTESIAN_POINT('Origin',(4.76104848420342,-17.542318193471,0.972561099047131));
#274627=CARTESIAN_POINT('Origin',(15.4290484842034,-17.542318193471,0.972561099047131));
#274628=CARTESIAN_POINT('Ctrl Pts',(6.14788848420341,-39.301220262464,-48.8447285308283));
#274629=CARTESIAN_POINT('Ctrl Pts',(6.12358695752485,-39.2643430009178,
-48.8140432447869));
#274630=CARTESIAN_POINT('Ctrl Pts',(6.09957618354499,-39.2274383836317,
-48.7831598317274));
#274631=CARTESIAN_POINT('Ctrl Pts',(5.437097966389,-38.1960065787892,-47.9150276671609));
#274632=CARTESIAN_POINT('Ctrl Pts',(5.01156238585601,-37.1907219414009,
-46.9354646126805));
#274633=CARTESIAN_POINT('Ctrl Pts',(4.82218298524757,-36.14112535664,-45.7133319051272));
#274634=CARTESIAN_POINT('Ctrl Pts',(4.80568122363092,-36.0301270662342,
-45.5814189805682));
#274635=CARTESIAN_POINT('Ctrl Pts',(4.79296103895618,-35.920447712068,-45.4483672846184));
#274636=CARTESIAN_POINT('Ctrl Pts',(4.79296103895619,-39.7424219671274,
-43.7467147117553));
#274637=CARTESIAN_POINT('Ctrl Pts',(4.80658157259404,-39.7697128227896,
-43.9293220908689));
#274638=CARTESIAN_POINT('Ctrl Pts',(4.8245384335836,-39.7950224166943,-44.1121867583887));
#274639=CARTESIAN_POINT('Ctrl Pts',(5.02532215959839,-40.0053675853797,
-45.7630200136485));
#274640=CARTESIAN_POINT('Ctrl Pts',(5.47477154367342,-40.0560861146367,
-47.2039255265971));
#274641=CARTESIAN_POINT('Ctrl Pts',(6.14788848420341,-40.0042318660923,
-48.5317275987882));
#274642=CARTESIAN_POINT('Origin',(4.76104848420342,-17.542318193471,0.972561099047131));
#274643=CARTESIAN_POINT('Origin',(15.4290484842034,-17.542318193471,0.972561099047131));
#274644=CARTESIAN_POINT('Ctrl Pts',(4.79296103895618,-48.5549566816842,
-38.1538301299319));
#274645=CARTESIAN_POINT('Ctrl Pts',(4.80658157259404,-48.6196173756195,
-38.3267730117436));
#274646=CARTESIAN_POINT('Ctrl Pts',(4.8245384335836,-48.6823935963878,-38.5003794870745));
#274647=CARTESIAN_POINT('Ctrl Pts',(5.02532215959839,-49.2313697518226,
-40.0714048552417));
#274648=CARTESIAN_POINT('Ctrl Pts',(5.47477154367344,-49.5805610610339,
-41.4702781504429));
#274649=CARTESIAN_POINT('Ctrl Pts',(6.14788848420341,-49.8059055261328,
-42.7798456660969));
#274650=CARTESIAN_POINT('Origin',(4.76104848420342,-17.542318193471,0.972561099047131));
#274651=CARTESIAN_POINT('Ctrl Pts',(6.14788848420341,-49.1833329657638,
-43.2321711079742));
#274652=CARTESIAN_POINT('Ctrl Pts',(6.12358695752485,-49.1408817311566,
-43.2098235828558));
#274653=CARTESIAN_POINT('Ctrl Pts',(6.099576183545,-49.0983625456749,-43.1872879478481));
#274654=CARTESIAN_POINT('Ctrl Pts',(5.43709796638902,-47.9089751742594,
-42.5525732844655));
#274655=CARTESIAN_POINT('Ctrl Pts',(5.01156238585602,-46.7219958072237,
-41.8034264616706));
#274656=CARTESIAN_POINT('Ctrl Pts',(4.82218298524757,-45.4412397484704,
-40.8262236866132));
#274657=CARTESIAN_POINT('Ctrl Pts',(4.80568122363092,-45.3052407978386,
-40.7202712181862));
#274658=CARTESIAN_POINT('Ctrl Pts',(4.79296103895619,-45.1702951976398,
-40.6129306409918));
#274659=CARTESIAN_POINT('Origin',(15.4290484842034,-17.542318193471,0.972561099047131));
#274660=CARTESIAN_POINT('Ctrl Pts',(6.14788848420341,-57.6825814930802,
-35.687654769834));
#274661=CARTESIAN_POINT('Ctrl Pts',(6.12358695752484,-57.636411608068,-35.6746216997216));
#274662=CARTESIAN_POINT('Ctrl Pts',(6.09957618354498,-57.5901361468258,
-35.6614187581536));
#274663=CARTESIAN_POINT('Ctrl Pts',(5.43709796638901,-56.2947751442819,
-35.2878616724436));
#274664=CARTESIAN_POINT('Ctrl Pts',(5.01156238585601,-54.9779777416974,
-34.8018723922956));
#274665=CARTESIAN_POINT('Ctrl Pts',(4.82218298524757,-53.5220373944686,
-34.1123080001433));
#274666=CARTESIAN_POINT('Ctrl Pts',(4.80568122363092,-53.3669815903488,
-34.0369466191348));
#274667=CARTESIAN_POINT('Ctrl Pts',(4.79296103895619,-53.212667514387,-33.9600084589965));
#274668=CARTESIAN_POINT('Ctrl Pts',(4.79296103895619,-56.0120902791558,
-30.8509345021466));
#274669=CARTESIAN_POINT('Ctrl Pts',(4.80658157259404,-56.1112948287628,
-31.0066544528491));
#274670=CARTESIAN_POINT('Ctrl Pts',(4.8245384335836,-56.2087940543133,-31.1634152999628));
#274671=CARTESIAN_POINT('Ctrl Pts',(5.02532215959839,-57.0724083042252,
-32.5859714338324));
#274672=CARTESIAN_POINT('Ctrl Pts',(5.47477154367343,-57.7048110575724,
-33.881675035747));
#274673=CARTESIAN_POINT('Ctrl Pts',(6.14788848420341,-58.1975056018673,
-35.1157736104278));
#274674=CARTESIAN_POINT('Origin',(4.76104848420342,-17.542318193471,0.972561099047131));
#274675=CARTESIAN_POINT('Origin',(15.4290484842034,-17.542318193471,0.972561099047131));
#274676=CARTESIAN_POINT('Ctrl Pts',(4.79296103895619,-61.7879102380356,
-22.1571994105147));
#274677=CARTESIAN_POINT('Ctrl Pts',(4.80658157259404,-61.9173229284602,
-22.2888907210352));
#274678=CARTESIAN_POINT('Ctrl Pts',(4.8245384335836,-62.0452839747833,-22.4219547386908));
#274679=CARTESIAN_POINT('Ctrl Pts',(5.02532215959839,-63.1857922323702,
-23.633869109031));
#274680=CARTESIAN_POINT('Ctrl Pts',(5.47477154367342,-64.0737673949269,
-24.7697745527797));
#274681=CARTESIAN_POINT('Ctrl Pts',(6.14788848420341,-64.8122789026212,
-25.8744681569118));
#274682=CARTESIAN_POINT('Origin',(4.76104848420342,-17.542318193471,0.972561099047131));
#274683=CARTESIAN_POINT('Ctrl Pts',(6.14788848420341,-64.4275078998501,
-26.5409110829905));
#274684=CARTESIAN_POINT('Ctrl Pts',(6.12358695752485,-64.3796372099557,
-26.5377620755876));
#274685=CARTESIAN_POINT('Ctrl Pts',(6.099576183545,-64.3316279326636,-26.5344688593604));
#274686=CARTESIAN_POINT('Ctrl Pts',(5.43709796638901,-62.9869067906343,
-26.4383955884944));
#274687=CARTESIAN_POINT('Ctrl Pts',(5.01156238585603,-61.5978417176889,
-26.2368039145711));
#274688=CARTESIAN_POINT('Ctrl Pts',(4.82218298524757,-60.0303486615353,
-25.865015178158));
#274689=CARTESIAN_POINT('Ctrl Pts',(4.80568122363092,-59.8630126866079,
-25.8235385385422));
#274690=CARTESIAN_POINT('Ctrl Pts',(4.79296103895619,-59.6960744004836,
-25.7803653622482));
#274691=CARTESIAN_POINT('Origin',(15.4290484842034,-17.542318193471,0.972561099047131));
#274692=CARTESIAN_POINT('Ctrl Pts',(6.14788848420341,-69.1233265363499,
-16.1916966375046));
#274693=CARTESIAN_POINT('Ctrl Pts',(6.12358695752485,-69.0758472204306,
-16.1985693195453));
#274694=CARTESIAN_POINT('Ctrl Pts',(6.099576183545,-69.0282023628804,-16.2053297580107));
#274695=CARTESIAN_POINT('Ctrl Pts',(5.43709796638902,-67.6928918479603,
-16.3909391649362));
#274696=CARTESIAN_POINT('Ctrl Pts',(5.01156238585603,-66.2922679138154,
-16.4825556207321));
#274697=CARTESIAN_POINT('Ctrl Pts',(4.82218298524757,-64.6817291169572,
-16.4447914918798));
#274698=CARTESIAN_POINT('Ctrl Pts',(4.80568122363092,-64.5094263562936,
-16.4390123218349));
#274699=CARTESIAN_POINT('Ctrl Pts',(4.79296103895618,-64.3371598641692,
-16.4314910043572));
#274700=CARTESIAN_POINT('',(4.79296103895618,-65.6299855106615,-12.4525827957101));
#274701=CARTESIAN_POINT('Ctrl Pts',(4.79296103895619,-65.6299855106615,
-12.4525827957101));
#274702=CARTESIAN_POINT('Ctrl Pts',(4.80658157259404,-65.7839503863411,
-12.5544899238537));
#274703=CARTESIAN_POINT('Ctrl Pts',(4.8245384335836,-65.9367807416872,-12.6580415759677));
#274704=CARTESIAN_POINT('Ctrl Pts',(5.02532215959839,-67.3043373233267,
-13.6063477093843));
#274705=CARTESIAN_POINT('Ctrl Pts',(5.47477154367343,-68.4090761195117,
-14.5328104763962));
#274706=CARTESIAN_POINT('Ctrl Pts',(6.14788848420341,-69.3611280939478,
-15.4598186985709));
#274707=CARTESIAN_POINT('',(4.76104848420342,-64.9412958110162,-11.8470366407114));
#274708=CARTESIAN_POINT('Ctrl Pts',(4.76104848420342,-64.9412958110162,
-11.8470366407114));
#274709=CARTESIAN_POINT('Ctrl Pts',(4.76104848420342,-65.022269383582,-11.9406753940164));
#274710=CARTESIAN_POINT('Ctrl Pts',(4.76253146088449,-65.108399211661,-12.0298480784081));
#274711=CARTESIAN_POINT('Ctrl Pts',(4.76582549808661,-65.1993564521347,
-12.1141556807409));
#274712=CARTESIAN_POINT('Ctrl Pts',(4.76903287597436,-65.2879207954999,
-12.1962453242087));
#274713=CARTESIAN_POINT('Ctrl Pts',(4.77395772034264,-65.3810618737959,
-12.2737222219327));
#274714=CARTESIAN_POINT('Ctrl Pts',(4.78087046545162,-65.4784573259478,
-12.3461860128027));
#274715=CARTESIAN_POINT('Ctrl Pts',(4.78437871324304,-65.5278859356418,
-12.3829616974648));
#274716=CARTESIAN_POINT('Ctrl Pts',(4.78839840126648,-65.5784100024365,
-12.4184457115046));
#274717=CARTESIAN_POINT('Ctrl Pts',(4.79296103895619,-65.6299855106615,
-12.4525827957101));
#274718=CARTESIAN_POINT('Origin',(4.76104848420342,-17.542318193471,0.972561099047131));
#274719=CARTESIAN_POINT('Origin',(15.4290484842034,-17.542318193471,0.972561099047131));
#274720=CARTESIAN_POINT('Ctrl Pts',(4.79296103895619,24.6114380135421,-25.7803653622474));
#274721=CARTESIAN_POINT('Ctrl Pts',(4.80658157259404,24.7901923791228,-25.8265943844669));
#274722=CARTESIAN_POINT('Ctrl Pts',(4.8245384335836,24.9694097219037,-25.8708798924498));
#274723=CARTESIAN_POINT('Ctrl Pts',(5.02532215959839,26.5892124826232,-26.2526318315758));
#274724=CARTESIAN_POINT('Ctrl Pts',(5.47477154367343,28.016923034485,-26.4536881584052));
#274725=CARTESIAN_POINT('Ctrl Pts',(6.14788848420341,29.3428715129087,-26.5409110829896));
#274726=CARTESIAN_POINT('Origin',(4.76104848420342,-17.542318193471,0.972561099047131));
#274727=CARTESIAN_POINT('Ctrl Pts',(6.14788848420341,29.7276425156798,-25.8744681569108));
#274728=CARTESIAN_POINT('Ctrl Pts',(6.12358695752485,29.7009800503249,-25.834585427067));
#274729=CARTESIAN_POINT('Ctrl Pts',(6.099576183545,29.674123402766,-25.7946547814283));
#274730=CARTESIAN_POINT('Ctrl Pts',(5.43709796638902,28.9185609385567,-24.6781287468579));
#274731=CARTESIAN_POINT('Ctrl Pts',(5.01156238585602,28.0494448912749,-23.5759589431392));
#274732=CARTESIAN_POINT('Ctrl Pts',(4.82218298524757,26.9437198726235,-22.4043645044611));
#274733=CARTESIAN_POINT('Ctrl Pts',(4.80568122363092,26.8241320615889,-22.2801856190147));
#274734=CARTESIAN_POINT('Ctrl Pts',(4.79296103895619,26.7032738510941,-22.1571994105139));
#274735=CARTESIAN_POINT('Origin',(15.4290484842034,-17.542318193471,0.972561099047131));
#274736=CARTESIAN_POINT('Ctrl Pts',(6.14788848420341,23.112869214926,-35.115773610427));
#274737=CARTESIAN_POINT('Ctrl Pts',(6.12358695752485,23.0950814742058,-35.0712189756663));
#274738=CARTESIAN_POINT('Ctrl Pts',(6.099576183545,23.0771137568824,-35.0265770994354));
#274739=CARTESIAN_POINT('Ctrl Pts',(5.43709796638905,22.5702009610012,-33.7773595681114));
#274740=CARTESIAN_POINT('Ctrl Pts',(5.01156238585603,21.9492311720527,-32.5185754320954));
#274741=CARTESIAN_POINT('Ctrl Pts',(4.82218298524757,21.1112570786857,-31.1426899846619));
#274742=CARTESIAN_POINT('Ctrl Pts',(4.80568122363092,21.0201007902822,-30.9963610018075));
#274743=CARTESIAN_POINT('Ctrl Pts',(4.79296103895619,20.9274538922144,-30.8509345021458));
#274744=CARTESIAN_POINT('Ctrl Pts',(4.79296103895619,18.1280311274457,-33.9600084589958));
#274745=CARTESIAN_POINT('Ctrl Pts',(4.80658157259404,18.2932677270847,-34.042392388553));
#274746=CARTESIAN_POINT('Ctrl Pts',(4.8245384335836,18.4593612660923,-34.1229715326951));
#274747=CARTESIAN_POINT('Ctrl Pts',(5.02532215959839,19.9643967590154,-34.8331572067992));
#274748=CARTESIAN_POINT('Ctrl Pts',(5.47477154367342,21.3191064490006,-35.3266576853357));
#274749=CARTESIAN_POINT('Ctrl Pts',(6.1478884842034,22.597945106139,-35.6876547698332));
#274750=CARTESIAN_POINT('Origin',(4.76104848420342,-17.542318193471,0.972561099047131));
#274751=CARTESIAN_POINT('Origin',(15.4290484842034,-17.542318193471,0.972561099047131));
#274752=CARTESIAN_POINT('Ctrl Pts',(6.14788848420341,14.7212691391918,-42.7798456660962));
#274753=CARTESIAN_POINT('Ctrl Pts',(6.12358695752485,14.7131335327306,-42.7325663777545));
#274754=CARTESIAN_POINT('Ctrl Pts',(6.099576183545,14.7048400211086,-42.6851643351381));
#274755=CARTESIAN_POINT('Ctrl Pts',(5.43709796638902,14.4687314151729,-41.35785210759));
#274756=CARTESIAN_POINT('Ctrl Pts',(5.01156238585603,14.1230472440783,-39.9974685463373));
#274757=CARTESIAN_POINT('Ctrl Pts',(4.82218298524757,13.5894475649218,-38.4774248864324));
#274758=CARTESIAN_POINT('Ctrl Pts',(4.80568122363092,13.5307067663691,-38.3153410848847));
#274759=CARTESIAN_POINT('Ctrl Pts',(4.79296103895619,13.470320294743,-38.1538301299313));
#274760=CARTESIAN_POINT('Ctrl Pts',(4.79296103895619,10.0856588106987,-40.6129306409912));
#274761=CARTESIAN_POINT('Ctrl Pts',(4.80658157259404,10.2301560120985,-40.7278689048426));
#274762=CARTESIAN_POINT('Ctrl Pts',(4.8245384335836,10.375866662673,-40.8412199898834));
#274763=CARTESIAN_POINT('Ctrl Pts',(5.02532215959839,11.7003576147974,-41.8488008771582));
#274764=CARTESIAN_POINT('Ctrl Pts',(5.47477154367342,12.9228591288354,-42.6131771684116));
#274765=CARTESIAN_POINT('Ctrl Pts',(6.14788848420341,14.0986965788227,-43.2321711079735));
#274766=CARTESIAN_POINT('Origin',(4.76104848420342,-17.542318193471,0.972561099047131));
#274767=CARTESIAN_POINT('Origin',(15.4290484842034,-17.542318193471,0.972561099047131));
#274768=CARTESIAN_POINT('Ctrl Pts',(4.79296103895619,29.2525234772276,-16.4314910043563));
#274769=CARTESIAN_POINT('Ctrl Pts',(4.80658157259404,29.4369831852156,-16.4395446891357));
#274770=CARTESIAN_POINT('Ctrl Pts',(4.82453843358361,29.62149167391,-16.4456010717549));
#274771=CARTESIAN_POINT('Ctrl Pts',(5.02532215959839,31.2852685491064,-16.482234884314));
#274772=CARTESIAN_POINT('Ctrl Pts',(5.47477154367342,32.7235821608131,-16.3820599331787));
#274773=CARTESIAN_POINT('Ctrl Pts',(6.1478884842034,34.0386901494082,-16.1916966375036));
#274774=CARTESIAN_POINT('',(4.76104848420342,29.8566594240745,-11.8470366407105));
#274775=CARTESIAN_POINT('Origin',(4.76104848420342,-17.542318193471,0.972561099047131));
#274776=CARTESIAN_POINT('',(4.79296103895619,30.5453491237198,-12.4525827957091));
#274777=CARTESIAN_POINT('Ctrl Pts',(4.79296103895619,30.5453491237198,-12.4525827957091));
#274778=CARTESIAN_POINT('Ctrl Pts',(4.77035892158032,30.2898575046396,-12.2834765820334));
#274779=CARTESIAN_POINT('Ctrl Pts',(4.76104848420342,30.0580786215828,-12.0799600742301));
#274780=CARTESIAN_POINT('Ctrl Pts',(4.76104848420342,29.8566594240745,-11.8470366407104));
#274781=CARTESIAN_POINT('Ctrl Pts',(6.14788848420342,34.2764917070062,-15.4598186985698));
#274782=CARTESIAN_POINT('Ctrl Pts',(6.12358695752485,34.2421197946934,-15.4263509403157));
#274783=CARTESIAN_POINT('Ctrl Pts',(6.099576183545,34.2075479812697,-15.3928766860921));
#274784=CARTESIAN_POINT('Ctrl Pts',(5.43709796638905,33.2363575540093,-14.4578396936725));
#274785=CARTESIAN_POINT('Ctrl Pts',(5.01156238585603,32.157079790142,-13.5604543314709));
#274786=CARTESIAN_POINT('Ctrl Pts',(4.82218298524757,30.8319293353784,-12.6443552004521));
#274787=CARTESIAN_POINT('Ctrl Pts',(4.80568122363092,30.6891365629009,-12.5477536255844));
#274788=CARTESIAN_POINT('Ctrl Pts',(4.79296103895619,30.5453491237198,-12.4525827957091));
#274789=CARTESIAN_POINT('Origin',(15.4290484842034,-17.542318193471,0.972561099047131));
#274790=CARTESIAN_POINT('',(4.79296103895619,31.8484498133401,-6.32197605563879));
#274791=CARTESIAN_POINT('Ctrl Pts',(4.79296103895619,31.8484498133401,-6.32197605563879));
#274792=CARTESIAN_POINT('Ctrl Pts',(4.80658157259404,32.0305530893604,-6.29150241830728));
#274793=CARTESIAN_POINT('Ctrl Pts',(4.8245384335836,32.2122888176425,-6.25906498258073));
#274794=CARTESIAN_POINT('Ctrl Pts',(5.02532215959839,33.8473247741825,-5.94897959517561));
#274795=CARTESIAN_POINT('Ctrl Pts',(5.47477154367343,35.2333802391081,-5.55195149213274));
#274796=CARTESIAN_POINT('Ctrl Pts',(6.14788848420341,36.4801712081848,-5.09232176568362));
#274797=CARTESIAN_POINT('',(4.76104848420342,30.9730026561923,-6.59505465837617));
#274798=CARTESIAN_POINT('Ctrl Pts',(4.76104848420342,30.9730026561923,-6.59505465837617));
#274799=CARTESIAN_POINT('Ctrl Pts',(4.76104848420342,31.085055529905,-6.54244936087672));
#274800=CARTESIAN_POINT('Ctrl Pts',(4.76253129040156,31.200002270829,-6.49602047434924));
#274801=CARTESIAN_POINT('Ctrl Pts',(4.76582494299153,31.3173800954912,-6.45599878354649));
#274802=CARTESIAN_POINT('Ctrl Pts',(4.76903192598598,31.4316692250621,-6.41703022863448));
#274803=CARTESIAN_POINT('Ctrl Pts',(4.77395615055087,31.5482630469874,-6.38413635141219));
#274804=CARTESIAN_POINT('Ctrl Pts',(4.78086799793772,31.666704173383,-6.35755179799359));
#274805=CARTESIAN_POINT('Ctrl Pts',(4.78437682990773,31.7268313705851,-6.34405602389403));
#274806=CARTESIAN_POINT('Ctrl Pts',(4.78839733376329,31.7874341667793,-6.33218657312908));
#274807=CARTESIAN_POINT('Ctrl Pts',(4.79296103895619,31.8484498133401,-6.3219760556388));
#274808=CARTESIAN_POINT('',(4.76104848420342,31.4862222820429,-1.71209609297289));
#274809=CARTESIAN_POINT('Origin',(4.76104848420342,-17.542318193471,0.972561099047131));
#274810=CARTESIAN_POINT('',(4.79296103895619,32.2857625843551,-2.16122297171639));
#274811=CARTESIAN_POINT('Ctrl Pts',(4.79296103895619,32.2857625843551,-2.16122297171639));
#274812=CARTESIAN_POINT('Ctrl Pts',(4.77035892158039,32.0006949113319,-2.0489318290534));
#274813=CARTESIAN_POINT('Ctrl Pts',(4.76104848420342,31.7316674917223,-1.89805218470827));
#274814=CARTESIAN_POINT('Ctrl Pts',(4.76104848420342,31.4862222820429,-1.71209609297289));
#274815=CARTESIAN_POINT('Ctrl Pts',(6.14788848420341,36.560610251444,-4.32699539176698));
#274816=CARTESIAN_POINT('Ctrl Pts',(6.12358695752485,36.5200311096761,-4.30140530673435));
#274817=CARTESIAN_POINT('Ctrl Pts',(6.099576183545,36.4792550845282,-4.27585042946278));
#274818=CARTESIAN_POINT('Ctrl Pts',(5.43709796638903,35.3348823761767,-3.56316808256783));
#274819=CARTESIAN_POINT('Ctrl Pts',(5.01156238585603,34.0926125129541,-2.90978720834442));
#274820=CARTESIAN_POINT('Ctrl Pts',(4.82218298524757,32.6059520557291,-2.28922131294187));
#274821=CARTESIAN_POINT('Ctrl Pts',(4.80568122363092,32.4461950511617,-2.22441900102026));
#274822=CARTESIAN_POINT('Ctrl Pts',(4.79296103895619,32.2857625843551,-2.16122297171639));
#274823=CARTESIAN_POINT('Origin',(15.4290484842034,-17.542318193471,0.972561099047131));
#274824=CARTESIAN_POINT('Ctrl Pts',(6.14788848420341,4.91959547915134,-48.5317275987877));
#274825=CARTESIAN_POINT('Ctrl Pts',(6.12358695752485,4.92146757199067,-48.4837899886367));
#274826=CARTESIAN_POINT('Ctrl Pts',(6.099576183545,4.9232107323245,-48.4356994763575));
#274827=CARTESIAN_POINT('Ctrl Pts',(5.43709796638903,4.96822539538845,-47.08830246608));
#274828=CARTESIAN_POINT('Ctrl Pts',(5.01156238585602,4.91293489920149,-45.6857747690617));
#274829=CARTESIAN_POINT('Ctrl Pts',(4.82218298524757,4.70703050072981,-44.0880060986017));
#274830=CARTESIAN_POINT('Ctrl Pts',(4.80568122363092,4.68327244679418,-43.917251318253));
#274831=CARTESIAN_POINT('Ctrl Pts',(4.79296103895619,4.65778558018633,-43.7467147117548));
#274832=CARTESIAN_POINT('Ctrl Pts',(4.79296103895618,0.835811325126994,
-45.448367284618));
#274833=CARTESIAN_POINT('Ctrl Pts',(4.80658157259404,0.953253907211932,
-45.5908365290982));
#274834=CARTESIAN_POINT('Ctrl Pts',(4.8245384335836,1.07221341472582,-45.7320055687025));
#274835=CARTESIAN_POINT('Ctrl Pts',(5.02532215959839,2.158273215831,-46.9929455494646));
#274836=CARTESIAN_POINT('Ctrl Pts',(5.47477154367344,3.19513737154524,-47.9947907416229));
#274837=CARTESIAN_POINT('Ctrl Pts',(6.14788848420341,4.21658387552305,-48.8447285308278));
#274838=CARTESIAN_POINT('Origin',(4.76104848420342,-17.542318193471,0.972561099047131));
#274839=CARTESIAN_POINT('Origin',(15.4290484842034,-17.542318193471,0.972561099047131));
#274840=CARTESIAN_POINT('Ctrl Pts',(6.1478884842034,-5.863771592603,-52.1200345674512));
#274841=CARTESIAN_POINT('Ctrl Pts',(6.12358695752484,-5.85197361990358,
-52.0735337390846));
#274842=CARTESIAN_POINT('Ctrl Pts',(6.099576183545,-5.84026997208509,-52.026856543293));
#274843=CARTESIAN_POINT('Ctrl Pts',(5.43709796638902,-5.51609939680166,
-50.7182624651634));
#274844=CARTESIAN_POINT('Ctrl Pts',(5.01156238585602,-5.2785797580845,-49.3348878228138));
#274845=CARTESIAN_POINT('Ctrl Pts',(4.82218298524757,-5.14778986561914,
-47.7292242996427));
#274846=CARTESIAN_POINT('Ctrl Pts',(4.80568122363092,-5.13552683397687,
-47.5572613437665));
#274847=CARTESIAN_POINT('Ctrl Pts',(4.79296103895619,-5.12500019719618,
-47.3851523537529));
#274848=CARTESIAN_POINT('Ctrl Pts',(4.79296103895618,-9.21724860845719,
-48.2549866055502));
#274849=CARTESIAN_POINT('Ctrl Pts',(4.80658157259404,-9.13199345007622,
-48.4187602410321));
#274850=CARTESIAN_POINT('Ctrl Pts',(4.8245384335836,-9.04498418693225,-48.5815774707651));
#274851=CARTESIAN_POINT('Ctrl Pts',(5.02532215959839,-8.24482156164778,
-50.0407674171938));
#274852=CARTESIAN_POINT('Ctrl Pts',(5.47477154367339,-7.43891070328836,
-51.236296067973));
#274853=CARTESIAN_POINT('Ctrl Pts',(6.14788848420341,-6.61649725898798,
-52.2800313469787));
#274854=CARTESIAN_POINT('Origin',(4.76104848420342,-17.542318193471,0.972561099047131));
#274855=CARTESIAN_POINT('Origin',(0.884028484203416,-17.542318193471,0.972561099047131));
#274856=CARTESIAN_POINT('',(11.5201159294509,31.84844981334,8.2670982537337));
#274857=CARTESIAN_POINT('Ctrl Pts',(11.5520284842034,30.9730026561921,8.54017685647109));
#274858=CARTESIAN_POINT('Ctrl Pts',(11.5520284842034,31.085055529906,8.4875715589711));
#274859=CARTESIAN_POINT('Ctrl Pts',(11.5505456780052,31.2000022708313,8.44114267244317));
#274860=CARTESIAN_POINT('Ctrl Pts',(11.5472520254152,31.3173800954948,8.40112098164014));
#274861=CARTESIAN_POINT('Ctrl Pts',(11.5440450424208,31.4316692250642,8.36215242672879));
#274862=CARTESIAN_POINT('Ctrl Pts',(11.5391208178559,31.5482630469879,8.329258549507));
#274863=CARTESIAN_POINT('Ctrl Pts',(11.5322089704692,31.6667041733819,8.30267399608871));
#274864=CARTESIAN_POINT('Ctrl Pts',(11.5287001384991,31.7268313705843,8.28917822198906));
#274865=CARTESIAN_POINT('Ctrl Pts',(11.5246796346436,31.7874341667788,8.27730877122404));
#274866=CARTESIAN_POINT('Ctrl Pts',(11.5201159294506,31.84844981334,8.2670982537337));
#274867=CARTESIAN_POINT('',(11.520115929451,32.2857625843551,4.10634516981065));
#274868=CARTESIAN_POINT('Ctrl Pts',(11.5201159294506,32.285762584355,4.10634516981064));
#274869=CARTESIAN_POINT('Ctrl Pts',(11.5379482942249,32.0608530926385,4.01775096495828));
#274870=CARTESIAN_POINT('Ctrl Pts',(11.5475950755165,31.8451991447526,3.90484982591719));
#274871=CARTESIAN_POINT('Ctrl Pts',(11.5516325551658,31.5894123057798,3.73310893941423));
#274872=CARTESIAN_POINT('Ctrl Pts',(11.5520284842034,31.5372399615042,3.69587069864284));
#274873=CARTESIAN_POINT('Ctrl Pts',(11.5520284842034,31.4862222820429,3.65721829106713));
#274874=CARTESIAN_POINT('',(10.1651884842034,36.560610251444,6.27211758986124));
#274875=CARTESIAN_POINT('Ctrl Pts',(10.1651884842034,36.560610251444,6.27211758986124));
#274876=CARTESIAN_POINT('Ctrl Pts',(10.189490010882,36.5200311096761,6.2465275048286));
#274877=CARTESIAN_POINT('Ctrl Pts',(10.2135007848618,36.4792550845282,6.22097262755701));
#274878=CARTESIAN_POINT('Ctrl Pts',(10.8759790020178,35.3348823761766,5.50829028066204));
#274879=CARTESIAN_POINT('Ctrl Pts',(11.3015145825508,34.092612512954,4.85490940643868));
#274880=CARTESIAN_POINT('Ctrl Pts',(11.4908939831593,32.605952055729,4.23434351103614));
#274881=CARTESIAN_POINT('Ctrl Pts',(11.5073957447759,32.4461950511616,4.16954119911451));
#274882=CARTESIAN_POINT('Ctrl Pts',(11.5201159294506,32.285762584355,4.10634516981064));
#274883=CARTESIAN_POINT('',(10.1651884842034,36.4801712081847,7.03744396377858));
#274884=CARTESIAN_POINT('Origin',(10.1651884842034,-17.542318193471,0.972561099047131));
#274885=CARTESIAN_POINT('Ctrl Pts',(11.5201159294506,31.84844981334,8.2670982537337));
#274886=CARTESIAN_POINT('Ctrl Pts',(11.5064953958128,32.0305530893603,8.2366246164022));
#274887=CARTESIAN_POINT('Ctrl Pts',(11.4885385348232,32.2122888176424,8.20418718067565));
#274888=CARTESIAN_POINT('Ctrl Pts',(11.2877548088084,33.8473247741825,7.89410179327056));
#274889=CARTESIAN_POINT('Ctrl Pts',(10.8383054247334,35.233380239108,7.49707369022769));
#274890=CARTESIAN_POINT('Ctrl Pts',(10.1651884842034,36.4801712081847,7.03744396377858));
#274891=CARTESIAN_POINT('Origin',(0.561048484203417,-17.542318193471,0.972561099047131));
#274892=CARTESIAN_POINT('',(6.14788848420341,36.4801712081847,7.03744396377859));
#274893=CARTESIAN_POINT('',(8.15653848420342,36.4801712081847,7.03744396377858));
#274894=CARTESIAN_POINT('',(6.14788848420341,36.560610251444,6.27211758986124));
#274895=CARTESIAN_POINT('',(8.15653848420341,36.560610251444,6.27211758986124));
#274896=CARTESIAN_POINT('Origin',(6.14788848420341,-17.542318193471,0.972561099047131));
#274897=CARTESIAN_POINT('Origin',(15.4290484842034,-17.542318193471,0.972561099047131));
#274898=CARTESIAN_POINT('',(4.79296103895619,31.84844981334,8.2670982537337));
#274899=CARTESIAN_POINT('',(4.76104848420342,30.9730026561922,8.54017685647106));
#274900=CARTESIAN_POINT('Ctrl Pts',(4.79296103895619,31.84844981334,8.2670982537337));
#274901=CARTESIAN_POINT('Ctrl Pts',(4.77035892158034,31.5462649115901,8.31766666361755));
#274902=CARTESIAN_POINT('Ctrl Pts',(4.76104848420342,31.2517467446016,8.40931528004612));
#274903=CARTESIAN_POINT('Ctrl Pts',(4.76104848420342,30.9730026561922,8.54017685647107));
#274904=CARTESIAN_POINT('Ctrl Pts',(6.14788848420341,36.4801712081847,7.03744396377859));
#274905=CARTESIAN_POINT('Ctrl Pts',(6.12358695752485,36.4351583401774,7.05403796607894));
#274906=CARTESIAN_POINT('Ctrl Pts',(6.099576183545,36.3899602112693,7.07055659563583));
#274907=CARTESIAN_POINT('Ctrl Pts',(5.43709796638902,35.1224198004911,7.52973665861739));
#274908=CARTESIAN_POINT('Ctrl Pts',(5.01156238585602,33.7714509920082,7.91055716538982));
#274909=CARTESIAN_POINT('Ctrl Pts',(4.82218298524757,32.1882547280908,8.20846811774149));
#274910=CARTESIAN_POINT('Ctrl Pts',(4.80568122363092,32.0185156391322,8.23863899473005));
#274911=CARTESIAN_POINT('Ctrl Pts',(4.79296103895619,31.84844981334,8.2670982537337));
#274912=CARTESIAN_POINT('',(4.79296103895619,32.2857625843551,4.10634516981065));
#274913=CARTESIAN_POINT('Ctrl Pts',(4.79296103895619,32.2857625843551,4.10634516981065));
#274914=CARTESIAN_POINT('Ctrl Pts',(4.80658157259404,32.4575506414171,4.17401428507293));
#274915=CARTESIAN_POINT('Ctrl Pts',(4.8245384335836,32.6285708858962,4.24352786755193));
#274916=CARTESIAN_POINT('Ctrl Pts',(5.02532215959839,34.163407006706,4.88678023553691));
#274917=CARTESIAN_POINT('Ctrl Pts',(5.47477154367344,35.4366270500011,5.56330945723206));
#274918=CARTESIAN_POINT('Ctrl Pts',(6.14788848420341,36.560610251444,6.27211758986124));
#274919=CARTESIAN_POINT('',(4.76104848420342,31.4862222820429,3.65721829106715));
#274920=CARTESIAN_POINT('Ctrl Pts',(4.76104848420342,31.4862222820429,3.65721829106714));
#274921=CARTESIAN_POINT('Ctrl Pts',(4.76104848420342,31.5848954455554,3.73197581381493));
#274922=CARTESIAN_POINT('Ctrl Pts',(4.76253147480131,31.6876836794715,3.80129276825595));
#274923=CARTESIAN_POINT('Ctrl Pts',(4.7658255451976,31.7941823732019,3.86484722694874));
#274924=CARTESIAN_POINT('Ctrl Pts',(4.76903295628176,31.8978793345982,3.9267297160083));
#274925=CARTESIAN_POINT('Ctrl Pts',(4.7739578530675,32.0050940194892,3.98314864997226));
#274926=CARTESIAN_POINT('Ctrl Pts',(4.78087067578756,32.1154278760504,4.03377943482262));
#274927=CARTESIAN_POINT('Ctrl Pts',(4.78437887355451,32.1714213543851,4.05947412041549));
#274928=CARTESIAN_POINT('Ctrl Pts',(4.78839849197318,32.2282177698636,4.08367766456516));
#274929=CARTESIAN_POINT('Ctrl Pts',(4.79296103895619,32.2857625843551,4.10634516981065));
#274930=CARTESIAN_POINT('Origin',(4.76104848420342,-17.542318193471,0.972561099047131));
#274931=CARTESIAN_POINT('Origin',(4.76104848420342,-17.542318193471,0.972561099047131));
#274932=CARTESIAN_POINT('Origin',(4.76104848420342,-22.8798040147369,51.7553464718149));
#274933=CARTESIAN_POINT('Origin',(4.76104848420342,-12.2048323722054,51.7553464718149));
#274934=CARTESIAN_POINT('Origin',(4.76104848420342,-1.76313447216181,49.5358950681846));
#274935=CARTESIAN_POINT('Origin',(4.76104848420342,7.98893738233642,45.193992937372));
#274936=CARTESIAN_POINT('Origin',(4.76104848420342,16.6251708556151,38.9194020372516));
#274937=CARTESIAN_POINT('Origin',(4.76104848420342,23.7681211036458,30.9863520989864));
#274938=CARTESIAN_POINT('Origin',(4.76104848420342,29.1056069249115,21.7415554718757));
#274939=CARTESIAN_POINT('Origin',(4.76104848420342,32.4043545769244,11.5890541299801));
#274940=CARTESIAN_POINT('Origin',(4.76104848420342,33.520192958144,0.972561099047131));
#274941=CARTESIAN_POINT('Origin',(4.76104848420342,32.4043545769246,-9.6439319318852));
#274942=CARTESIAN_POINT('Origin',(4.76104848420342,-67.4889909638663,-9.6439319318862));
#274943=CARTESIAN_POINT('Origin',(4.76104848420342,-68.604829345086,0.972561099046774));
#274944=CARTESIAN_POINT('Origin',(4.76104848420342,-67.4889909638665,11.5890541299798));
#274945=CARTESIAN_POINT('Origin',(4.76104848420342,-64.1902433118537,21.7415554718754));
#274946=CARTESIAN_POINT('Origin',(4.76104848420342,-58.852757490588,30.9863520989862));
#274947=CARTESIAN_POINT('Origin',(4.76104848420342,-51.7098072425573,38.9194020372514));
#274948=CARTESIAN_POINT('Origin',(4.76104848420342,-43.0735737692787,45.1939929373718));
#274949=CARTESIAN_POINT('Origin',(4.76104848420342,-33.3215019147805,49.5358950681845));
#274950=CARTESIAN_POINT('Origin',(11.5520284842034,22.8992029103953,27.9355151336363));
#274951=CARTESIAN_POINT('',(11.5520284842034,32.2857625843551,4.10634516981065));
#274952=CARTESIAN_POINT('Origin',(11.5520284842034,22.8992029103953,-25.990392935542));
#274953=CARTESIAN_POINT('',(11.5520284842034,32.2857625843551,-2.16122297171639));
#274954=CARTESIAN_POINT('Origin',(11.5520284842034,33.520192958144,0.972561099047131));
#274955=CARTESIAN_POINT('Origin',(11.5520284842034,16.4095452815284,35.7545749286233));
#274956=CARTESIAN_POINT('',(11.5520284842034,30.5453491237196,14.397704993804));
#274957=CARTESIAN_POINT('Origin',(11.5520284842034,27.6213720070744,-16.9929226666352));
#274958=CARTESIAN_POINT('',(11.5520284842034,31.84844981334,8.2670982537337));
#274959=CARTESIAN_POINT('Origin',(11.5520284842034,32.4043545769244,11.5890541299801));
#274960=CARTESIAN_POINT('Origin',(11.5520284842034,13.5002200109301,-36.4290209703537));
#274961=CARTESIAN_POINT('Origin',(11.5520284842034,-40.1302762914843,-42.0658132711382));
#274962=CARTESIAN_POINT('Origin',(11.5520284842034,20.5980922391598,-29.1576000604339));
#274963=CARTESIAN_POINT('Origin',(11.5520284842034,-30.6884940271654,-45.8216220909116));
#274964=CARTESIAN_POINT('Origin',(11.5520284842034,26.0290455134887,-20.5693465272905));
#274965=CARTESIAN_POINT('Origin',(11.5520284842034,-20.6721607965636,-47.5323005618802));
#274966=CARTESIAN_POINT('Origin',(11.5520284842034,27.6213720070741,18.93804486473));
#274967=CARTESIAN_POINT('',(11.5520284842034,31.8484498133401,-6.32197605563879));
#274968=CARTESIAN_POINT('Origin',(11.5520284842034,16.4095452815289,-33.8094527305286));
#274969=CARTESIAN_POINT('',(11.5520284842034,30.5453491237198,-12.4525827957091));
#274970=CARTESIAN_POINT('Origin',(11.5520284842034,32.4043545769246,-9.6439319318852));
#274971=CARTESIAN_POINT('Origin',(11.5520284842034,30.3696711225592,9.15539674730717));
#274972=CARTESIAN_POINT('Origin',(11.5520284842034,8.43602829968808,-40.1083716185434));
#274973=CARTESIAN_POINT('Origin',(11.5520284842034,29.5557211152235,-11.0396082613347));
#274974=CARTESIAN_POINT('Origin',(11.5520284842034,-10.5190384255555,-47.1230838261165));
#274975=CARTESIAN_POINT('Origin',(11.5520284842034,31.0239863977013,-0.984880553546538));
#274976=CARTESIAN_POINT('Origin',(11.5520284842034,-0.672867081840852,-44.6118566186133));
#274977=CARTESIAN_POINT('Origin',(11.5520284842034,-51.4941816684702,-33.8094527305293));
#274978=CARTESIAN_POINT('',(11.5520284842034,-65.6299855106615,-12.4525827957101));
#274979=CARTESIAN_POINT('Origin',(11.5520284842034,-62.7060083940165,18.9380448647291));
#274980=CARTESIAN_POINT('',(11.5520284842034,-66.9330862002819,-6.32197605563978));
#274981=CARTESIAN_POINT('Origin',(11.5520284842034,-67.4889909638663,-9.6439319318862));
#274982=CARTESIAN_POINT('Origin',(11.5520284842034,-34.4117693051002,-44.6118566186136));
#274983=CARTESIAN_POINT('Origin',(11.5520284842034,-66.1086227846432,-0.984880553547528));
#274984=CARTESIAN_POINT('Origin',(11.5520284842034,-43.5206646866292,-40.1083716185439));
#274985=CARTESIAN_POINT('Origin',(11.5520284842034,-65.4543075095014,9.15539674730621));
#274986=CARTESIAN_POINT('Origin',(11.5520284842034,-14.4124755903774,-47.5323005618801));
#274987=CARTESIAN_POINT('Origin',(11.5520284842034,-61.1136819004303,-20.5693465272914));
#274988=CARTESIAN_POINT('Origin',(11.5520284842034,-24.5655979613854,-47.1230838261167));
#274989=CARTESIAN_POINT('Origin',(11.5520284842034,-64.6403575021652,-11.0396082613357));
#274990=CARTESIAN_POINT('Origin',(11.5520284842034,-4.39614235977561,-45.8216220909114));
#274991=CARTESIAN_POINT('Origin',(11.5520284842034,-55.6827286261012,-29.1576000604346));
#274992=CARTESIAN_POINT('Origin',(11.5520284842034,5.04563990454314,-42.0658132711378));
#274993=CARTESIAN_POINT('Origin',(11.5520284842034,-48.5848563978714,-36.4290209703543));
#274994=CARTESIAN_POINT('Origin',(11.5520284842034,-55.6827286261016,31.1027222585284));
#274995=CARTESIAN_POINT('',(11.5520284842034,-35.9204477120687,47.3934894827124));
#274996=CARTESIAN_POINT('Origin',(11.5520284842034,-4.39614235977625,47.7667442890058));
#274997=CARTESIAN_POINT('',(11.5520284842034,-29.9596361897455,49.3302745518473));
#274998=CARTESIAN_POINT('Origin',(11.5520284842034,-33.3215019147805,49.5358950681845));
#274999=CARTESIAN_POINT('Origin',(11.5520284842034,-64.6403575021654,12.9847304594293));
#275000=CARTESIAN_POINT('',(11.5520284842034,-53.2126675143875,35.9051306570903));
#275001=CARTESIAN_POINT('Origin',(11.5520284842034,-24.5655979613861,49.0682060242108));
#275002=CARTESIAN_POINT('',(11.5520284842034,-48.5549566816847,40.0989523280257));
#275003=CARTESIAN_POINT('Origin',(11.5520284842034,-51.7098072425573,38.9194020372514));
#275004=CARTESIAN_POINT('Origin',(11.5520284842034,-61.1136819004306,22.5144687253851));
#275005=CARTESIAN_POINT('',(11.5520284842034,-45.1702951976404,42.5580528390857));
#275006=CARTESIAN_POINT('Origin',(11.5520284842034,-14.412475590378,49.4774227599744));
#275007=CARTESIAN_POINT('',(11.5520284842034,-39.742421967128,45.6918369098492));
#275008=CARTESIAN_POINT('Origin',(11.5520284842034,-43.0735737692787,45.1939929373718));
#275009=CARTESIAN_POINT('Origin',(11.5520284842034,-43.5206646866298,42.0534938166378));
#275010=CARTESIAN_POINT('',(11.5520284842034,-61.7879102380359,24.1023216086084));
#275011=CARTESIAN_POINT('Origin',(11.5520284842034,-64.1902433118537,21.7415554718754));
#275012=CARTESIAN_POINT('Origin',(11.5520284842034,-66.1086227846432,2.93000275164114));
#275013=CARTESIAN_POINT('',(11.5520284842034,-59.6960744004839,27.7254875603419));
#275014=CARTESIAN_POINT('Origin',(11.5520284842034,-34.4117693051008,46.5569788167076));
#275015=CARTESIAN_POINT('',(11.5520284842034,-56.0120902791562,32.7960567002403));
#275016=CARTESIAN_POINT('Origin',(11.5520284842034,-58.852757490588,30.9863520989862));
#275017=CARTESIAN_POINT('Origin',(11.5520284842034,-62.7060083940162,-16.9929226666355));
#275018=CARTESIAN_POINT('',(11.5520284842034,-66.933086200282,8.26709825373337));
#275019=CARTESIAN_POINT('Origin',(11.5520284842034,-51.4941816684706,35.7545749286231));
#275020=CARTESIAN_POINT('',(11.5520284842034,-65.6299855106617,14.3977049938037));
#275021=CARTESIAN_POINT('Origin',(11.5520284842034,-67.4889909638665,11.5890541299798));
#275022=CARTESIAN_POINT('Origin',(11.5520284842034,-57.9838392973371,-25.9903929355423));
#275023=CARTESIAN_POINT('',(11.5520284842034,-67.370398971297,-2.16122297171674));
#275024=CARTESIAN_POINT('Origin',(11.5520284842034,-57.9838392973375,27.935515133636));
#275025=CARTESIAN_POINT('',(11.5520284842034,-67.370398971297,4.1063451698103));
#275026=CARTESIAN_POINT('Origin',(11.5520284842034,-68.604829345086,0.972561099046774));
#275027=CARTESIAN_POINT('Origin',(11.5520284842034,-0.672867081841461,46.5569788167077));
#275028=CARTESIAN_POINT('',(11.5520284842034,20.927453892214,32.7960567002406));
#275029=CARTESIAN_POINT('Origin',(11.5520284842034,31.0239863977013,2.93000275164145));
#275030=CARTESIAN_POINT('',(11.5520284842034,24.6114380135418,27.7254875603422));
#275031=CARTESIAN_POINT('Origin',(11.5520284842034,23.7681211036458,30.9863520989864));
#275032=CARTESIAN_POINT('Origin',(11.5520284842034,-10.5190384255562,49.0682060242109));
#275033=CARTESIAN_POINT('',(11.5520284842034,13.4703202947425,40.098952328026));
#275034=CARTESIAN_POINT('Origin',(11.5520284842034,29.5557211152234,12.9847304594296));
#275035=CARTESIAN_POINT('',(11.5520284842034,18.1280311274453,35.9051306570905));
#275036=CARTESIAN_POINT('Origin',(11.5520284842034,16.6251708556151,38.9194020372516));
#275037=CARTESIAN_POINT('Origin',(11.5520284842034,8.43602829968752,42.053493816638));
#275038=CARTESIAN_POINT('',(11.5520284842034,26.7032738510938,24.1023216086087));
#275039=CARTESIAN_POINT('Origin',(11.5520284842034,29.1056069249115,21.7415554718757));
#275040=CARTESIAN_POINT('Origin',(11.5520284842034,-20.6721607965643,49.4774227599744));
#275041=CARTESIAN_POINT('',(11.5520284842034,4.65778558018571,45.6918369098494));
#275042=CARTESIAN_POINT('Origin',(11.5520284842034,26.0290455134884,22.5144687253854));
#275043=CARTESIAN_POINT('',(11.5520284842034,10.0856588106982,42.5580528390859));
#275044=CARTESIAN_POINT('Origin',(11.5520284842034,7.98893738233642,45.193992937372));
#275045=CARTESIAN_POINT('Origin',(11.5520284842034,-30.688494027166,47.7667442890057));
#275046=CARTESIAN_POINT('',(11.5520284842034,-5.12500019719682,49.3302745518473));
#275047=CARTESIAN_POINT('Origin',(11.5520284842034,20.5980922391594,31.1027222585287));
#275048=CARTESIAN_POINT('',(11.5520284842034,0.835811325126388,47.3934894827125));
#275049=CARTESIAN_POINT('Origin',(11.5520284842034,-1.76313447216181,49.5358950681846));
#275050=CARTESIAN_POINT('Origin',(11.5520284842034,-40.1302762914848,44.0109354692322));
#275051=CARTESIAN_POINT('',(11.5520284842034,-15.4504823559191,50.8552480699037));
#275052=CARTESIAN_POINT('Origin',(11.5520284842034,13.5002200109296,38.3741431684484));
#275053=CARTESIAN_POINT('',(11.5520284842034,-9.21724860845784,50.2001088036446));
#275054=CARTESIAN_POINT('Origin',(11.5520284842034,-12.2048323722054,51.7553464718149));
#275055=CARTESIAN_POINT('Origin',(11.5520284842034,-48.5848563978719,38.3741431684482));
#275056=CARTESIAN_POINT('',(11.5520284842034,-25.8673877784845,50.2001088036445));
#275057=CARTESIAN_POINT('Origin',(11.5520284842034,5.04563990454256,44.0109354692323));
#275058=CARTESIAN_POINT('',(11.5520284842034,-19.6341540310232,50.8552480699037));
#275059=CARTESIAN_POINT('Origin',(11.5520284842034,-22.8798040147369,51.7553464718149));
#275060=CARTESIAN_POINT('Origin',(19.4612584842034,-7.33631819347099,3.49256109904713));
#275061=CARTESIAN_POINT('',(19.4612584842034,-7.33631819347099,3.49256109904713));
#275062=CARTESIAN_POINT('',(19.4612584842034,-7.33631819347099,-1.54743890095287));
#275063=CARTESIAN_POINT('Origin',(19.4612584842034,-7.33631819347099,-1.54743890095287));
#275064=CARTESIAN_POINT('Origin',(19.4612584842034,-17.542318193471,3.49256109904713));
#310587=UNCERTAINTY_MEASURE_WITH_UNIT(LENGTH_MEASURE(0.01),#310624,
'DISTANCE_ACCURACY_VALUE',
'Maximum model space distance between geometric entities at asserted c
onnectivities');
#310601=UNCERTAINTY_MEASURE_WITH_UNIT(LENGTH_MEASURE(0.01),#310624,
'DISTANCE_ACCURACY_VALUE',
'Maximum model space distance between geometric entities at asserted c
onnectivities');
#310609=(
GEOMETRIC_REPRESENTATION_CONTEXT(3)
GLOBAL_UNCERTAINTY_ASSIGNED_CONTEXT((#310587))
GLOBAL_UNIT_ASSIGNED_CONTEXT((#310624,#310626,#310627))
REPRESENTATION_CONTEXT('','3D')
);
#310623=(
GEOMETRIC_REPRESENTATION_CONTEXT(3)
GLOBAL_UNCERTAINTY_ASSIGNED_CONTEXT((#310601))
GLOBAL_UNIT_ASSIGNED_CONTEXT((#310624,#310626,#310627))
REPRESENTATION_CONTEXT('','3D')
);
#310624=(
LENGTH_UNIT()
NAMED_UNIT(*)
SI_UNIT(.MILLI.,.METRE.)
);
#310626=(
NAMED_UNIT(*)
PLANE_ANGLE_UNIT()
SI_UNIT($,.RADIAN.)
);
#310627=(
NAMED_UNIT(*)
SI_UNIT($,.STERADIAN.)
SOLID_ANGLE_UNIT()
);
#310635=SHAPE_DEFINITION_REPRESENTATION(#310656,#310900);
#310656=PRODUCT_DEFINITION_SHAPE('',$,#310922);
#310900=SHAPE_REPRESENTATION('',(#103547),#310609);
#310914=PRODUCT_DEFINITION_CONTEXT('part definition',#310979,'design');
#310922=PRODUCT_DEFINITION('30-Tooth Sprocket','30-Tooth Sprocket',#310943,
#310914);
#310943=PRODUCT_DEFINITION_FORMATION('',$,#310988);
#310979=APPLICATION_CONTEXT(
'Core Data for Automotive Mechanical Design Process');
#310980=PRODUCT_CONTEXT('part definition',#310979,'mechanical');
#310988=PRODUCT('30-Tooth Sprocket','30-Tooth Sprocket',$,(#310980));
#311003=PRESENTATION_STYLE_ASSIGNMENT((#311010));
#311010=SURFACE_STYLE_USAGE(.BOTH.,#311017);
#311017=SURFACE_SIDE_STYLE('',(#311024));
#311024=SURFACE_STYLE_FILL_AREA(#311031);
#311031=FILL_AREA_STYLE('Opaque(97,158,199)',(#311038));
#311038=FILL_AREA_STYLE_COLOUR('Opaque(97,158,199)',#311045);
#311045=COLOUR_RGB('Opaque(97,158,199)',0.380392156862745,0.619607843137255,
0.780392156862745);
ENDSEC;
END-ISO-10303-21;
